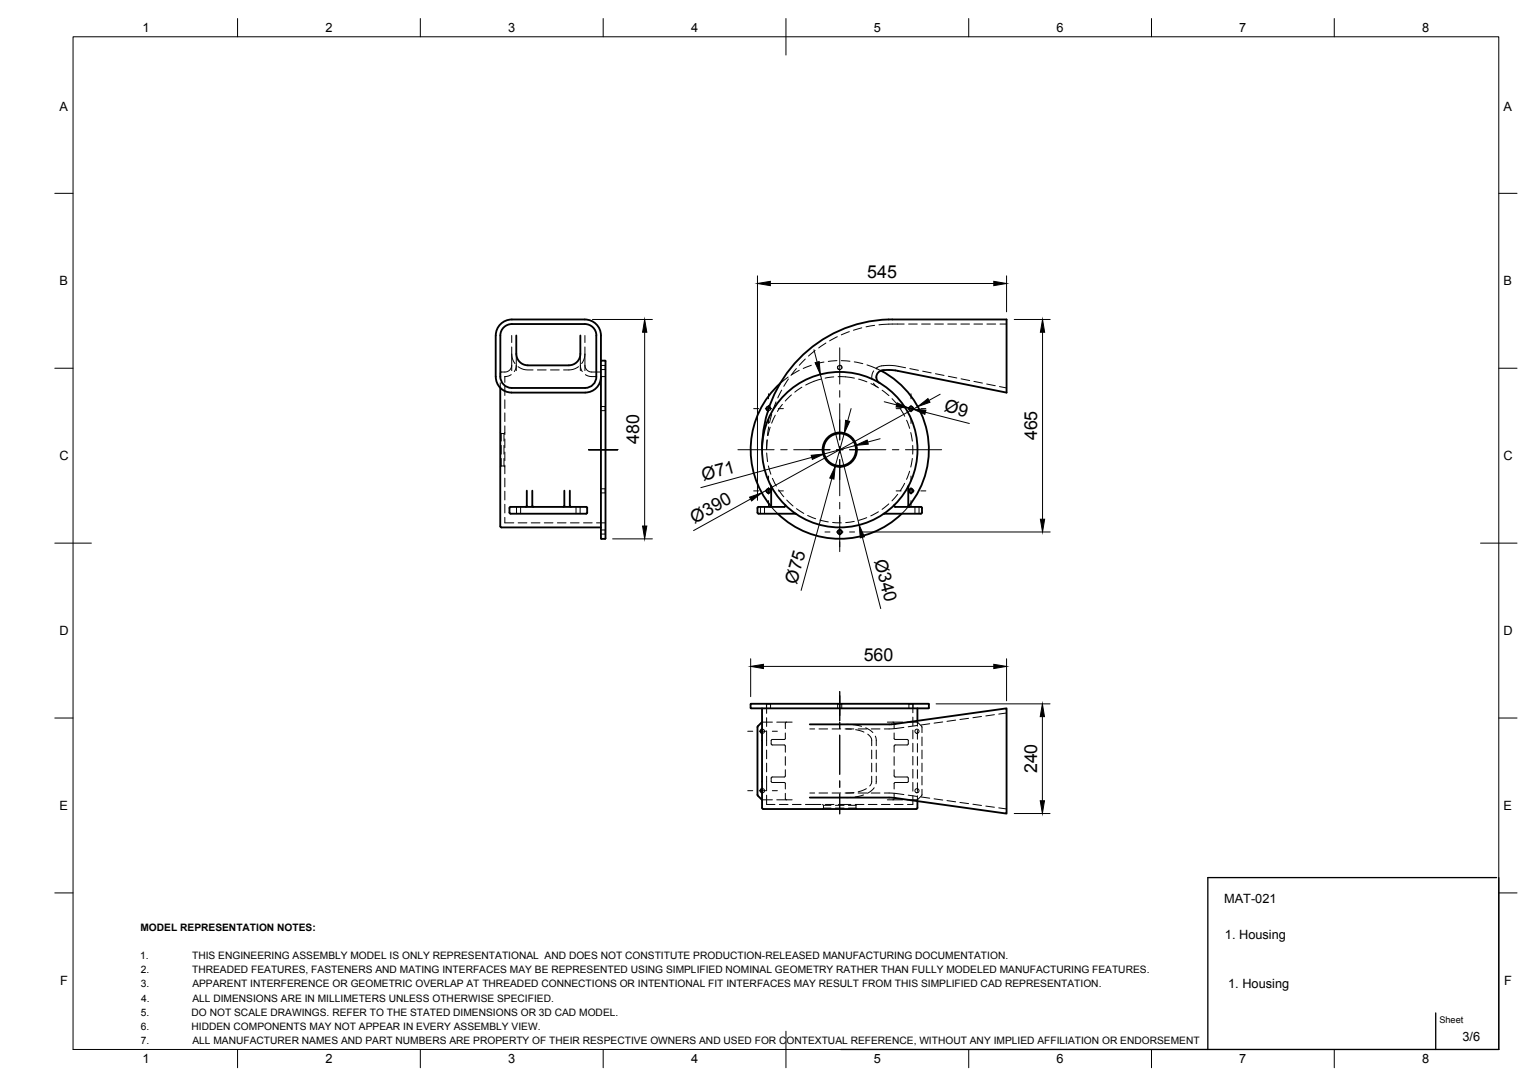
ISO-10303-21;
HEADER;
/* Generated by software containing ST-Developer
 * from STEP Tools, Inc. (www.steptools.com) 
 */

FILE_DESCRIPTION(
/* description */ ('STEP AP214'),
/* implementation_level */ '2;1');

FILE_NAME(
/* name */ '1. Housing.step',
/* time_stamp */ '2026-11-14T06:27:21-08:00',
/* author */ (''),
/* organization */ (''),
/* preprocessor_version */ 'ST-DEVELOPER v20.2',
/* originating_system */ 'Autodesk Translation Framework v15.17.0.0',
/* authorisation */ '');

FILE_SCHEMA (('AUTOMOTIVE_DESIGN { 1 0 10303 214 3 1 1 }'));
ENDSEC;

DATA;
#10=MECHANICAL_DESIGN_GEOMETRIC_PRESENTATION_REPRESENTATION('',(#35),#27541);
#27=SHAPE_REPRESENTATION_RELATIONSHIP('SRR','None',#27561,#31);
#31=ADVANCED_BREP_SHAPE_REPRESENTATION('',(#62),#27537);
#35=STYLED_ITEM('',(#27590),#62);
#62=MANIFOLD_SOLID_BREP('Body1',#11823);
#89=(
BOUNDED_SURFACE()
B_SPLINE_SURFACE(3,2,((#19385,#19386,#19387),(#19388,#19389,#19390),(#19391,
#19392,#19393),(#19394,#19395,#19396)),.UNSPECIFIED.,.F.,.F.,.F.)
B_SPLINE_SURFACE_WITH_KNOTS((4,4),(3,3),(4.8580615908835,4.90978454023457),
(0.,1.),.UNSPECIFIED.)
GEOMETRIC_REPRESENTATION_ITEM()
RATIONAL_B_SPLINE_SURFACE(((1.,0.714186893169771,1.),(1.,0.715014795561183,
1.),(1.,0.715838114785164,1.),(1.,0.716655802814478,1.)))
REPRESENTATION_ITEM('')
SURFACE()
);
#90=(
BOUNDED_SURFACE()
B_SPLINE_SURFACE(3,2,((#19398,#19399,#19400),(#19401,#19402,#19403),(#19404,
#19405,#19406),(#19407,#19408,#19409),(#19410,#19411,#19412),(#19413,#19414,
#19415)),.UNSPECIFIED.,.F.,.F.,.F.)
B_SPLINE_SURFACE_WITH_KNOTS((4,2,4),(3,3),(0.,0.00940850202008467,0.0188170040401693),
(0.,1.),.UNSPECIFIED.)
GEOMETRIC_REPRESENTATION_ITEM()
RATIONAL_B_SPLINE_SURFACE(((1.,0.707106781186548,1.),(1.,0.707160279657923,
1.),(1.,0.707792511111606,1.),(1.,0.710169444241066,1.),(1.,0.711914113489046,
1.),(1.,0.71418689316977,1.)))
REPRESENTATION_ITEM('')
SURFACE()
);
#91=(
BOUNDED_SURFACE()
B_SPLINE_SURFACE(3,2,((#19609,#19610,#19611),(#19612,#19613,#19614),(#19615,
#19616,#19617),(#19618,#19619,#19620)),.UNSPECIFIED.,.F.,.F.,.F.)
B_SPLINE_SURFACE_WITH_KNOTS((4,4),(3,3),(4.51499342053481,4.56671636988588),
(0.,1.),.UNSPECIFIED.)
GEOMETRIC_REPRESENTATION_ITEM()
RATIONAL_B_SPLINE_SURFACE(((1.,0.716655802814478,1.),(1.,0.715838114785163,
1.),(1.,0.715014795561185,1.),(1.,0.71418689316977,1.)))
REPRESENTATION_ITEM('')
SURFACE()
);
#92=(
BOUNDED_SURFACE()
B_SPLINE_SURFACE(3,2,((#19622,#19623,#19624),(#19625,#19626,#19627),(#19628,
#19629,#19630),(#19631,#19632,#19633),(#19634,#19635,#19636),(#19637,#19638,
#19639)),.UNSPECIFIED.,.F.,.F.,.F.)
B_SPLINE_SURFACE_WITH_KNOTS((4,2,4),(3,3),(0.,0.00940850202008465,0.0188170040401693),
(0.,1.),.UNSPECIFIED.)
GEOMETRIC_REPRESENTATION_ITEM()
RATIONAL_B_SPLINE_SURFACE(((1.,0.707106781186548,1.),(1.,0.707160279657923,
1.),(1.,0.707792511111607,1.),(1.,0.710169444241066,1.),(1.,0.711914113489046,
1.),(1.,0.714186893169771,1.)))
REPRESENTATION_ITEM('')
SURFACE()
);
#93=(
BOUNDED_SURFACE()
B_SPLINE_SURFACE(3,2,((#19835,#19836,#19837),(#19838,#19839,#19840),(#19841,
#19842,#19843),(#19844,#19845,#19846)),.UNSPECIFIED.,.F.,.F.,.F.)
B_SPLINE_SURFACE_WITH_KNOTS((4,4),(3,3),(0.,0.00696902930539232),(0.,1.),
 .UNSPECIFIED.)
GEOMETRIC_REPRESENTATION_ITEM()
RATIONAL_B_SPLINE_SURFACE(((1.,0.707106781186548,1.),(1.,0.707276293971192,
1.),(1.,0.707276133936197,1.),(1.,0.707106781186548,1.)))
REPRESENTATION_ITEM('')
SURFACE()
);
#94=(
BOUNDED_SURFACE()
B_SPLINE_SURFACE(3,2,((#20013,#20014,#20015),(#20016,#20017,#20018),(#20019,
#20020,#20021),(#20022,#20023,#20024)),.UNSPECIFIED.,.F.,.F.,.F.)
B_SPLINE_SURFACE_WITH_KNOTS((4,4),(3,3),(-3.46944695195361E-18,0.0069690293053924),
(0.,1.),.UNSPECIFIED.)
GEOMETRIC_REPRESENTATION_ITEM()
RATIONAL_B_SPLINE_SURFACE(((1.,0.707106781186547,1.),(1.,0.707276133936197,
1.),(1.,0.707276293971194,1.),(1.,0.707106781186547,1.)))
REPRESENTATION_ITEM('')
SURFACE()
);
#95=(
BOUNDED_SURFACE()
B_SPLINE_SURFACE(3,2,((#20196,#20197,#20198),(#20199,#20200,#20201),(#20202,
#20203,#20204),(#20205,#20206,#20207),(#20208,#20209,#20210),(#20211,#20212,
#20213),(#20214,#20215,#20216),(#20217,#20218,#20219),(#20220,#20221,#20222),
(#20223,#20224,#20225),(#20226,#20227,#20228),(#20229,#20230,#20231),(#20232,
#20233,#20234),(#20235,#20236,#20237),(#20238,#20239,#20240),(#20241,#20242,
#20243),(#20244,#20245,#20246),(#20247,#20248,#20249),(#20250,#20251,#20252),
(#20253,#20254,#20255),(#20256,#20257,#20258),(#20259,#20260,#20261),(#20262,
#20263,#20264),(#20265,#20266,#20267),(#20268,#20269,#20270),(#20271,#20272,
#20273),(#20274,#20275,#20276),(#20277,#20278,#20279),(#20280,#20281,#20282),
(#20283,#20284,#20285),(#20286,#20287,#20288),(#20289,#20290,#20291),(#20292,
#20293,#20294),(#20295,#20296,#20297),(#20298,#20299,#20300),(#20301,#20302,
#20303),(#20304,#20305,#20306),(#20307,#20308,#20309),(#20310,#20311,#20312),
(#20313,#20314,#20315),(#20316,#20317,#20318),(#20319,#20320,#20321)),
 .UNSPECIFIED.,.F.,.F.,.F.)
B_SPLINE_SURFACE_WITH_KNOTS((4,2,2,2,2,2,2,2,2,2,2,2,2,2,2,2,2,2,2,2,4),
(3,3),(-2.08303249130885E-5,0.0143336398395062,0.0286672796790123,0.0430009195185185,
0.0501677394382716,0.0573345593580246,0.0716681991975308,0.086001839037037,
0.100335478876543,0.10391888883642,0.107502298796296,0.114669118716049,
0.143336398395062,0.157670038234568,0.164836858154321,0.168420268114197,
0.172003678074074,0.200670957753086,0.215004597592592,0.222171417512345,
0.229338237432099),(-2.08303249131434E-5,1.),.UNSPECIFIED.)
GEOMETRIC_REPRESENTATION_ITEM()
RATIONAL_B_SPLINE_SURFACE(((1.0000122047894,0.707042750109083,1.),(1.00001165037919,
0.720350516962147,1.),(1.00001112382429,0.732989659531489,1.),(1.00001011791998,
0.757134849634084,1.),(1.00000963848844,0.768642868569314,1.),(1.00000871933328,
0.790705778250952,1.),(1.00000827963345,0.801260098384088,1.),(1.00000764642268,
0.816459351757556,1.),(1.00000743975533,0.821420084465031,1.),(1.00000703478498,
0.83114077643061,1.),(1.00000683745965,0.835877268408073,1.),(1.00000626125477,
0.849708182685712,1.),(1.00000589749541,0.858439668308409,1.),(1.00000520616899,
0.875033898554219,1.),(1.00000487861603,0.882896305052256,1.),(1.00000425655478,
0.897827931239669,1.),(1.00000396205458,0.904896956720407,1.),(1.00000361326943,
0.913269009275214,1.),(1.00000354448169,0.914920153464801,1.),(1.00000340882056,
0.918176490920243,1.),(1.00000334190225,0.919782762301647,1.),(1.00000314471007,
0.924516058194436,1.),(1.00000301778241,0.927562762018953,1.),(1.00000240476706,
0.942277255118144,1.),(1.00000198296934,0.952401862584738,1.),(1.0000014408388,
0.965414874578938,1.),(1.00000127533739,0.969387482068598,1.),(1.00000104925894,
0.974814148585356,1.),(1.00000097760072,0.976534194128842,1.),(1.0000008756353,
0.978981717570214,1.),(1.00000084253972,0.979776126225882,1.),(1.00000077837346,
0.981316338884772,1.),(1.00000074729348,0.982062366173435,1.),(1.00000047647086,
0.988563047871222,1.),(1.0000002985221,0.992834434768701,1.),(1.00000011982054,
0.997123891622385,1.),(1.00000007504731,0.998198604512223,1.),(1.00000003010649,
0.999277339877407,1.),(1.00000001883456,0.999547905223287,1.),(1.00000000377558,
0.999909373055038,1.),(0.999999999994412,1.00000013413799,1.),(1.,1.,1.)))
REPRESENTATION_ITEM('')
SURFACE()
);
#96=(
BOUNDED_SURFACE()
B_SPLINE_SURFACE(3,2,((#20325,#20326,#20327),(#20328,#20329,#20330),(#20331,
#20332,#20333),(#20334,#20335,#20336),(#20337,#20338,#20339),(#20340,#20341,
#20342),(#20343,#20344,#20345),(#20346,#20347,#20348),(#20349,#20350,#20351),
(#20352,#20353,#20354),(#20355,#20356,#20357),(#20358,#20359,#20360),(#20361,
#20362,#20363),(#20364,#20365,#20366),(#20367,#20368,#20369),(#20370,#20371,
#20372),(#20373,#20374,#20375),(#20376,#20377,#20378),(#20379,#20380,#20381),
(#20382,#20383,#20384),(#20385,#20386,#20387),(#20388,#20389,#20390),(#20391,
#20392,#20393),(#20394,#20395,#20396),(#20397,#20398,#20399),(#20400,#20401,
#20402),(#20403,#20404,#20405),(#20406,#20407,#20408),(#20409,#20410,#20411),
(#20412,#20413,#20414),(#20415,#20416,#20417),(#20418,#20419,#20420),(#20421,
#20422,#20423),(#20424,#20425,#20426),(#20427,#20428,#20429),(#20430,#20431,
#20432),(#20433,#20434,#20435),(#20436,#20437,#20438),(#20439,#20440,#20441),
(#20442,#20443,#20444),(#20445,#20446,#20447),(#20448,#20449,#20450),(#20451,
#20452,#20453),(#20454,#20455,#20456)),.UNSPECIFIED.,.F.,.F.,.F.)
B_SPLINE_SURFACE_WITH_KNOTS((4,2,2,2,2,2,2,2,2,2,2,2,2,2,2,2,2,2,2,2,2,
4),(3,3),(0.,0.0134129175527026,0.0268258351054052,0.0335322938817565,0.0368855232699322,
0.0402387526581078,0.0469452114344592,0.0536516702108105,0.0603581289871618,
0.0637113583753374,0.0670645877635131,0.0737710465398644,0.0804775053162157,
0.0838307347043914,0.087183964092567,0.0905371934807427,0.0938904228689183,
0.0955670375630061,0.097243652257094,0.10059688164527,0.103950111033445,
0.107303340421621),(0.,1.),.UNSPECIFIED.)
GEOMETRIC_REPRESENTATION_ITEM()
RATIONAL_B_SPLINE_SURFACE(((1.,0.707106781186548,1.),(1.,0.692435075400818,
1.),(1.,0.677415299381314,1.),(1.,0.646471084851157,1.),(1.,0.63054857897306,
1.),(1.,0.605783714123967,1.),(1.,0.597381263170599,1.),(1.,0.584523409966303,
1.),(1.,0.580195037882829,1.),(1.,0.571447189603745,1.),(1.,0.56702021135895,
1.),(1.,0.553648440044157,1.),(1.,0.544640272160397,1.),(1.,0.526415110072128,
1.),(1.,0.51719794329847,1.),(1.,0.498539063660432,1.),(1.,0.489096977102246,
1.),(1.,0.474763871347392,1.),(1.,0.469957977677047,1.),(1.,0.460292200732756,
1.),(1.,0.455439380592845,1.),(1.,0.440953583986291,1.),(1.,0.431346601606819,
1.),(1.,0.412377017907544,1.),(1.,0.403011528923584,1.),(1.,0.389351796591827,
1.),(1.,0.384854537462147,1.),(1.,0.376177060931741,1.),(1.,0.371982004193461,
1.),(1.,0.363944301803223,1.),(1.,0.360101535707161,1.),(1.,0.352850425245751,
1.),(1.,0.349441929276512,1.),(1.,0.344732409186674,1.),(1.,0.343226443951063,
1.),(1.,0.340393341785211,1.),(1.,0.339063346120003,1.),(1.,0.335345379291585,
1.),(1.,0.333229400572389,1.),(1.,0.329790328424277,1.),(1.,0.328467328740303,
1.),(1.,0.326681697649074,1.),(1.,0.326219073225421,1.),(1.,0.326219127150631,
1.)))
REPRESENTATION_ITEM('')
SURFACE()
);
#97=(
BOUNDED_SURFACE()
B_SPLINE_SURFACE(3,2,((#20457,#20458,#20459),(#20460,#20461,#20462),(#20463,
#20464,#20465),(#20466,#20467,#20468),(#20469,#20470,#20471),(#20472,#20473,
#20474),(#20475,#20476,#20477),(#20478,#20479,#20480),(#20481,#20482,#20483),
(#20484,#20485,#20486),(#20487,#20488,#20489),(#20490,#20491,#20492),(#20493,
#20494,#20495),(#20496,#20497,#20498),(#20499,#20500,#20501),(#20502,#20503,
#20504),(#20505,#20506,#20507),(#20508,#20509,#20510),(#20511,#20512,#20513),
(#20514,#20515,#20516),(#20517,#20518,#20519),(#20520,#20521,#20522),(#20523,
#20524,#20525),(#20526,#20527,#20528),(#20529,#20530,#20531),(#20532,#20533,
#20534),(#20535,#20536,#20537),(#20538,#20539,#20540),(#20541,#20542,#20543),
(#20544,#20545,#20546),(#20547,#20548,#20549),(#20550,#20551,#20552),(#20553,
#20554,#20555),(#20556,#20557,#20558),(#20559,#20560,#20561),(#20562,#20563,
#20564),(#20565,#20566,#20567),(#20568,#20569,#20570),(#20571,#20572,#20573),
(#20574,#20575,#20576),(#20577,#20578,#20579),(#20580,#20581,#20582),(#20583,
#20584,#20585),(#20586,#20587,#20588),(#20589,#20590,#20591),(#20592,#20593,
#20594)),.UNSPECIFIED.,.F.,.F.,.F.)
B_SPLINE_SURFACE_WITH_KNOTS((4,2,2,2,2,2,2,2,2,2,2,2,2,2,2,2,2,2,2,2,2,
2,4),(3,3),(0.,0.00337857504716453,0.00675715009432906,0.0101357251414936,
0.0118250126650759,0.0135143001886581,0.0168928752358226,0.0202714502829872,
0.0236500253301517,0.025339312853734,0.0270286003773162,0.0337857504716453,
0.0405429005659744,0.0439214756131389,0.0473000506603034,0.0540572007546325,
0.0608143508489615,0.0675715009432906,0.0709500759904551,0.0743286510376197,
0.0810858011319487,0.0946001013206068,0.108114401509265),(0.,1.),
 .UNSPECIFIED.)
GEOMETRIC_REPRESENTATION_ITEM()
RATIONAL_B_SPLINE_SURFACE(((1.,0.32621912715063,1.),(1.,0.326219068852315,
1.),(1.,0.326681715050001,1.),(1.,0.328468620211654,1.),(1.,0.32979287514018,
1.),(1.,0.333236641150815,1.),(1.,0.33535605687756,1.),(1.,0.339081365168914,
1.),(1.,0.340414170801098,1.),(1.,0.34325369454111,1.),(1.,0.344759275422739,
1.),(1.,0.349467998468122,1.),(1.,0.352877852486234,1.),(1.,0.360137129421262,
1.),(1.,0.363986689978637,1.),(1.,0.372044278816161,1.),(1.,0.37625241873187,
1.),(1.,0.382785172371532,1.),(1.,0.385002445825604,1.),(1.,0.389470383554178,
1.),(1.,0.391724641087319,1.),(1.,0.403081163733532,1.),(1.,0.412431784451128,
1.),(1.,0.431385484934698,1.),(1.,0.440991365631289,1.),(1.,0.455485214499389,
1.),(1.,0.460343755015816,1.),(1.,0.469998884973711,1.),(1.,0.474798889815344,
1.),(1.,0.48911283545623,1.),(1.,0.498540168051125,1.),(1.,0.517166334136202,
1.),(1.,0.526365537230034,1.),(1.,0.544552008443698,1.),(1.,0.553539446694172,
1.),(1.,0.566878228388953,1.),(1.,0.571308885947455,1.),(1.,0.580076325189919,
1.),(1.,0.584413767367782,1.),(1.,0.597296867359364,1.),(1.,0.605713540127583,
1.),(1.,0.630514573129104,1.),(1.,0.646452607022068,1.),(1.,0.677415122211174,
1.),(1.,0.692437606205447,1.),(1.,0.707106781186548,1.)))
REPRESENTATION_ITEM('')
SURFACE()
);
#98=(
BOUNDED_SURFACE()
B_SPLINE_SURFACE(3,2,((#20598,#20599,#20600),(#20601,#20602,#20603),(#20604,
#20605,#20606),(#20607,#20608,#20609),(#20610,#20611,#20612),(#20613,#20614,
#20615),(#20616,#20617,#20618),(#20619,#20620,#20621),(#20622,#20623,#20624),
(#20625,#20626,#20627),(#20628,#20629,#20630),(#20631,#20632,#20633),(#20634,
#20635,#20636),(#20637,#20638,#20639),(#20640,#20641,#20642),(#20643,#20644,
#20645),(#20646,#20647,#20648),(#20649,#20650,#20651),(#20652,#20653,#20654),
(#20655,#20656,#20657),(#20658,#20659,#20660),(#20661,#20662,#20663),(#20664,
#20665,#20666),(#20667,#20668,#20669),(#20670,#20671,#20672),(#20673,#20674,
#20675),(#20676,#20677,#20678),(#20679,#20680,#20681),(#20682,#20683,#20684),
(#20685,#20686,#20687),(#20688,#20689,#20690),(#20691,#20692,#20693),(#20694,
#20695,#20696),(#20697,#20698,#20699),(#20700,#20701,#20702),(#20703,#20704,
#20705),(#20706,#20707,#20708),(#20709,#20710,#20711),(#20712,#20713,#20714),
(#20715,#20716,#20717),(#20718,#20719,#20720),(#20721,#20722,#20723)),
 .UNSPECIFIED.,.F.,.F.,.F.)
B_SPLINE_SURFACE_WITH_KNOTS((4,2,2,2,2,2,2,2,2,2,2,2,2,2,2,2,2,2,2,2,4),
(3,3),(-2.08246099844738E-5,0.0143336398395062,0.0286672796790123,0.0430009195185185,
0.0501677394382716,0.0573345593580247,0.0716681991975308,0.086001839037037,
0.100335478876543,0.10391888883642,0.107502298796296,0.114669118716049,
0.143336398395062,0.157670038234568,0.164836858154321,0.168420268114197,
0.172003678074074,0.200670957753086,0.215004597592593,0.222171417512346,
0.229338237432099),(0.,1.00002082460998),.UNSPECIFIED.)
GEOMETRIC_REPRESENTATION_ITEM()
RATIONAL_B_SPLINE_SURFACE(((1.,0.707042767677887,1.00001220144021),(1.,
0.720350528626315,1.00001164718235),(1.,0.732989665864678,1.00001112077214),
(1.,0.757134851024669,1.00001011514401),(1.,0.768642869892271,1.000009635844),
(1.,0.790705779446232,1.00000871694103),(1.,0.801260099519581,1.00000827736183),
(1.,0.816459352806589,1.00000764432479),(1.,0.821420085485447,1.00000743771414),
(1.,0.831140777395743,1.00000703285491),(1.,0.835877269346536,1.00000683558371),
(1.,0.849708183543533,1.00000625953692),(1.,0.85843966911793,1.00000589587736),
(1.,0.875033899267846,1.00000520474062),(1.,0.882896305722012,1.00000487727752),
(1.,0.897827931823032,1.00000425538694),(1.,0.904896957262567,1.00000396096755),
(1.,0.913269009771199,1.00000361227809),(1.,0.914920153950816,1.00000354350922),
(1.,0.918176491388049,1.00000340788531),(1.,0.919782762760141,1.00000334098536),
(1.,0.924516058625678,1.00000314384728),(1.,0.927562762433317,1.00000301695444),
(1.,0.94227725544642,1.00000240410729),(1.,0.952401862855693,1.00000198242528),
(1.,0.965414874777115,1.00000144044349),(1.,0.969387482243809,1.00000127498749),
(1.,0.974814148729155,1.00000104897106),(1.,0.976534194262543,1.0000009773325),
(1.,0.97898171769053,1.00000087539506),(1.,0.979776126341324,1.00000084230856),
(1.,0.981316338991679,1.00000077815991),(1.,0.982062366275678,1.00000074708845),
(1.,0.988563047938719,1.00000047634013),(1.,0.992834434811244,1.0000002984402),
(1.,0.997123891638026,1.00000011978767),(1.,0.998198604522518,1.00000007502672),
(1.,0.999277339881537,1.00000003009823),(1.,0.999547905226004,1.00000001882939),
(1.,0.999909373055422,1.00000000377454),(1.,1.00000013413809,0.999999999994413),
(1.,1.,1.)))
REPRESENTATION_ITEM('')
SURFACE()
);
#99=(
BOUNDED_SURFACE()
B_SPLINE_SURFACE(3,2,((#20852,#20853,#20854),(#20855,#20856,#20857),(#20858,
#20859,#20860),(#20861,#20862,#20863)),.UNSPECIFIED.,.F.,.F.,.F.)
B_SPLINE_SURFACE_WITH_KNOTS((4,4),(3,3),(4.8580615908835,4.90978454023457),
(0.,1.),.UNSPECIFIED.)
GEOMETRIC_REPRESENTATION_ITEM()
RATIONAL_B_SPLINE_SURFACE(((1.,0.714186893169771,1.),(1.,0.715014795561184,
1.),(1.,0.715838114785164,1.),(1.,0.716655802814478,1.)))
REPRESENTATION_ITEM('')
SURFACE()
);
#100=(
BOUNDED_SURFACE()
B_SPLINE_SURFACE(3,2,((#20865,#20866,#20867),(#20868,#20869,#20870),(#20871,
#20872,#20873),(#20874,#20875,#20876),(#20877,#20878,#20879),(#20880,#20881,
#20882)),.UNSPECIFIED.,.F.,.F.,.F.)
B_SPLINE_SURFACE_WITH_KNOTS((4,2,4),(3,3),(0.,0.00940850202008467,0.0188170040401693),
(0.,1.),.UNSPECIFIED.)
GEOMETRIC_REPRESENTATION_ITEM()
RATIONAL_B_SPLINE_SURFACE(((1.,0.707106781186548,1.),(1.,0.707160279657923,
1.),(1.,0.707792511111606,1.),(1.,0.710169444241066,1.),(1.,0.711914113489048,
1.),(1.,0.714186893169771,1.)))
REPRESENTATION_ITEM('')
SURFACE()
);
#101=(
BOUNDED_SURFACE()
B_SPLINE_SURFACE(3,2,((#21103,#21104,#21105),(#21106,#21107,#21108),(#21109,
#21110,#21111),(#21112,#21113,#21114)),.UNSPECIFIED.,.F.,.F.,.F.)
B_SPLINE_SURFACE_WITH_KNOTS((4,4),(3,3),(4.51499342053481,4.56671636988588),
(0.,1.),.UNSPECIFIED.)
GEOMETRIC_REPRESENTATION_ITEM()
RATIONAL_B_SPLINE_SURFACE(((1.,0.716655802814478,1.),(1.,0.715838114785163,
1.),(1.,0.715014795561185,1.),(1.,0.71418689316977,1.)))
REPRESENTATION_ITEM('')
SURFACE()
);
#102=(
BOUNDED_SURFACE()
B_SPLINE_SURFACE(3,2,((#21116,#21117,#21118),(#21119,#21120,#21121),(#21122,
#21123,#21124),(#21125,#21126,#21127),(#21128,#21129,#21130),(#21131,#21132,
#21133)),.UNSPECIFIED.,.F.,.F.,.F.)
B_SPLINE_SURFACE_WITH_KNOTS((4,2,4),(3,3),(-1.38777878078145E-17,0.00940850202008464,
0.0188170040401693),(0.,1.),.UNSPECIFIED.)
GEOMETRIC_REPRESENTATION_ITEM()
RATIONAL_B_SPLINE_SURFACE(((1.,0.707106781186548,1.),(1.,0.707160279657923,
1.),(1.,0.707792511111607,1.),(1.,0.710169444241066,1.),(1.,0.711914113489046,
1.),(1.,0.714186893169771,1.)))
REPRESENTATION_ITEM('')
SURFACE()
);
#103=(
BOUNDED_SURFACE()
B_SPLINE_SURFACE(3,2,((#21362,#21363,#21364),(#21365,#21366,#21367),(#21368,
#21369,#21370),(#21371,#21372,#21373)),.UNSPECIFIED.,.F.,.F.,.F.)
B_SPLINE_SURFACE_WITH_KNOTS((4,4),(3,3),(0.,0.00696902930539231),(0.,1.),
 .UNSPECIFIED.)
GEOMETRIC_REPRESENTATION_ITEM()
RATIONAL_B_SPLINE_SURFACE(((1.,0.707106781186548,1.),(1.,0.707276293971192,
1.),(1.,0.707276133936197,1.),(1.,0.707106781186548,1.)))
REPRESENTATION_ITEM('')
SURFACE()
);
#104=(
BOUNDED_SURFACE()
B_SPLINE_SURFACE(3,2,((#21540,#21541,#21542),(#21543,#21544,#21545),(#21546,
#21547,#21548),(#21549,#21550,#21551)),.UNSPECIFIED.,.F.,.F.,.F.)
B_SPLINE_SURFACE_WITH_KNOTS((4,4),(3,3),(-3.46944695195361E-18,0.0069690293053924),
(0.,1.),.UNSPECIFIED.)
GEOMETRIC_REPRESENTATION_ITEM()
RATIONAL_B_SPLINE_SURFACE(((1.,0.707106781186547,1.),(1.,0.707276133936196,
1.),(1.,0.707276293971194,1.),(1.,0.707106781186547,1.)))
REPRESENTATION_ITEM('')
SURFACE()
);
#105=(
BOUNDED_SURFACE()
B_SPLINE_SURFACE(3,2,((#21711,#21712,#21713),(#21714,#21715,#21716),(#21717,
#21718,#21719),(#21720,#21721,#21722),(#21723,#21724,#21725),(#21726,#21727,
#21728),(#21729,#21730,#21731),(#21732,#21733,#21734),(#21735,#21736,#21737),
(#21738,#21739,#21740),(#21741,#21742,#21743),(#21744,#21745,#21746),(#21747,
#21748,#21749),(#21750,#21751,#21752),(#21753,#21754,#21755),(#21756,#21757,
#21758),(#21759,#21760,#21761),(#21762,#21763,#21764),(#21765,#21766,#21767),
(#21768,#21769,#21770),(#21771,#21772,#21773),(#21774,#21775,#21776),(#21777,
#21778,#21779),(#21780,#21781,#21782),(#21783,#21784,#21785),(#21786,#21787,
#21788),(#21789,#21790,#21791),(#21792,#21793,#21794),(#21795,#21796,#21797),
(#21798,#21799,#21800),(#21801,#21802,#21803),(#21804,#21805,#21806),(#21807,
#21808,#21809),(#21810,#21811,#21812),(#21813,#21814,#21815),(#21816,#21817,
#21818),(#21819,#21820,#21821),(#21822,#21823,#21824),(#21825,#21826,#21827),
(#21828,#21829,#21830),(#21831,#21832,#21833),(#21834,#21835,#21836)),
 .UNSPECIFIED.,.F.,.F.,.F.)
B_SPLINE_SURFACE_WITH_KNOTS((4,2,2,2,2,2,2,2,2,2,2,2,2,2,2,2,2,2,2,2,4),
(3,3),(-1.33632684703268E-5,0.0143336398395061,0.0286672796790123,0.0430009195185185,
0.0501677394382715,0.0573345593580246,0.0716681991975308,0.086001839037037,
0.100335478876543,0.10391888883642,0.107502298796296,0.114669118716049,
0.143336398395062,0.157670038234568,0.164836858154321,0.168420268114197,
0.172003678074074,0.200670957753086,0.215004597592592,0.222171417512345,
0.229338237432099),(-1.33632684703573E-5,1.),.UNSPECIFIED.)
GEOMETRIC_REPRESENTATION_ITEM()
RATIONAL_B_SPLINE_SURFACE(((1.00000782911927,0.707065704608532,1.),(1.000007473655,
0.72036575434847,1.),(1.00000713604048,0.732997937829732,1.),(1.00000649089595,
0.757136663085689,1.),(1.00000618332875,0.768644596089292,1.),(1.00000559366798,
0.790707341030961,1.),(1.00000531158966,0.801261582354705,1.),(1.00000490536929,
0.816460722237655,1.),(1.00000477278707,0.821421417903966,1.),(1.00000451298858,
0.831142037285297,1.),(1.0000043863995,0.835878493896513,1.),(1.00000401674981,
0.849709304899285,1.),(1.00000378338918,0.858440725325112,1.),(1.00000333988619,
0.875034831663981,1.),(1.00000312975286,0.882897179455003,1.),(1.00000273068518,
0.89782869414732,1.),(1.00000254175602,0.904897666844873,1.),(1.00000231800172,
0.913269656887061,1.),(1.00000227387268,0.914920788747183,1.),(1.00000218684271,
0.918177101888678,1.),(1.00000214391296,0.919783361275745,1.),(1.0000020174093,
0.924516621825683,1.),(1.00000193598206,0.92756330290103,1.),(1.00000154271755,
0.942277686126561,1.),(1.00000127212388,0.952402217994254,1.),(1.00000092433373,
0.965415132823172,1.),(1.00000081816048,0.969387710649768,1.),(1.00000067312556,
0.974814336645346,1.),(1.00000062715504,0.976534369345689,1.),(1.00000056174171,
0.978981874511646,1.),(1.00000054051007,0.979776277235544,1.),(1.00000049934583,
0.981316478393818,1.),(1.00000047940725,0.982062500111768,1.),(1.00000030566784,
0.988563133271413,1.),(1.00000019150931,0.992834488272736,1.),(1.00000007686784,
0.997123913098267,1.),(1.0000000481447,0.998198617963065,1.),(1.00000001931406,
0.999277345273439,1.),(1.00000001208284,0.999547908599034,1.),(1.00000000242213,
0.99990937373174,1.),(0.999999999996415,1.00000013413699,1.),(1.,1.,1.)))
REPRESENTATION_ITEM('')
SURFACE()
);
#106=(
BOUNDED_SURFACE()
B_SPLINE_SURFACE(3,2,((#21840,#21841,#21842),(#21843,#21844,#21845),(#21846,
#21847,#21848),(#21849,#21850,#21851),(#21852,#21853,#21854),(#21855,#21856,
#21857),(#21858,#21859,#21860),(#21861,#21862,#21863),(#21864,#21865,#21866),
(#21867,#21868,#21869),(#21870,#21871,#21872),(#21873,#21874,#21875),(#21876,
#21877,#21878),(#21879,#21880,#21881),(#21882,#21883,#21884),(#21885,#21886,
#21887),(#21888,#21889,#21890),(#21891,#21892,#21893),(#21894,#21895,#21896),
(#21897,#21898,#21899),(#21900,#21901,#21902),(#21903,#21904,#21905),(#21906,
#21907,#21908),(#21909,#21910,#21911),(#21912,#21913,#21914),(#21915,#21916,
#21917),(#21918,#21919,#21920),(#21921,#21922,#21923),(#21924,#21925,#21926),
(#21927,#21928,#21929),(#21930,#21931,#21932),(#21933,#21934,#21935),(#21936,
#21937,#21938),(#21939,#21940,#21941),(#21942,#21943,#21944),(#21945,#21946,
#21947),(#21948,#21949,#21950),(#21951,#21952,#21953),(#21954,#21955,#21956),
(#21957,#21958,#21959),(#21960,#21961,#21962),(#21963,#21964,#21965),(#21966,
#21967,#21968),(#21969,#21970,#21971),(#21972,#21973,#21974),(#21975,#21976,
#21977)),.UNSPECIFIED.,.F.,.F.,.F.)
B_SPLINE_SURFACE_WITH_KNOTS((4,2,2,2,2,2,2,2,2,2,2,2,2,2,2,2,2,2,2,2,2,
2,4),(3,3),(0.,0.0134129175527026,0.0268258351054052,0.0335322938817565,
0.0368855232699322,0.0402387526581078,0.0469452114344592,0.0536516702108105,
0.0603581289871618,0.0637113583753374,0.0670645877635131,0.0737710465398644,
0.07712427592804,0.0804775053162157,0.0838307347043914,0.087183964092567,
0.0905371934807427,0.0938904228689183,0.0955670375630061,0.097243652257094,
0.10059688164527,0.103950111033445,0.107303340421621),(0.,1.),
 .UNSPECIFIED.)
GEOMETRIC_REPRESENTATION_ITEM()
RATIONAL_B_SPLINE_SURFACE(((1.,0.707106781186548,1.),(1.,0.692435075401192,
1.),(1.,0.677415299380816,1.),(1.,0.646471084851654,1.),(1.,0.630548578972812,
1.),(1.,0.605783714124091,1.),(1.,0.597381263170474,1.),(1.,0.584523409966366,
1.),(1.,0.580195037882892,1.),(1.,0.571447189603682,1.),(1.,0.56702021135914,
1.),(1.,0.553648440043779,1.),(1.,0.544640272160396,1.),(1.,0.526415110072127,
1.),(1.,0.517197943298344,1.),(1.,0.498539063660557,1.),(1.,0.489096977102497,
1.),(1.,0.474763871347267,1.),(1.,0.469957977677141,1.),(1.,0.460292200732662,
1.),(1.,0.455439380593066,1.),(1.,0.440953583985851,1.),(1.,0.431346601607069,
1.),(1.,0.417119413832237,1.),(1.,0.412408247679678,1.),(1.,0.403077747649425,
1.),(1.,0.398458284812998,1.),(1.,0.389351796591827,1.),(1.,0.384854537462053,
1.),(1.,0.376177060931835,1.),(1.,0.371982004193336,1.),(1.,0.363944301803349,
1.),(1.,0.360101535706815,1.),(1.,0.352850425246096,1.),(1.,0.349441929276512,
1.),(1.,0.344732409186674,1.),(1.,0.343226443951127,1.),(1.,0.340393341785148,
1.),(1.,0.339063346120349,1.),(1.,0.335345379290893,1.),(1.,0.333229400572264,
1.),(1.,0.329790328424402,1.),(1.,0.328467328740178,1.),(1.,0.326681697649199,
1.),(1.,0.326219073225326,1.),(1.,0.326219127150631,1.)))
REPRESENTATION_ITEM('')
SURFACE()
);
#107=(
BOUNDED_SURFACE()
B_SPLINE_SURFACE(3,2,((#21978,#21979,#21980),(#21981,#21982,#21983),(#21984,
#21985,#21986),(#21987,#21988,#21989),(#21990,#21991,#21992),(#21993,#21994,
#21995),(#21996,#21997,#21998),(#21999,#22000,#22001),(#22002,#22003,#22004),
(#22005,#22006,#22007),(#22008,#22009,#22010),(#22011,#22012,#22013),(#22014,
#22015,#22016),(#22017,#22018,#22019),(#22020,#22021,#22022),(#22023,#22024,
#22025),(#22026,#22027,#22028),(#22029,#22030,#22031),(#22032,#22033,#22034),
(#22035,#22036,#22037),(#22038,#22039,#22040),(#22041,#22042,#22043),(#22044,
#22045,#22046),(#22047,#22048,#22049),(#22050,#22051,#22052),(#22053,#22054,
#22055),(#22056,#22057,#22058),(#22059,#22060,#22061),(#22062,#22063,#22064),
(#22065,#22066,#22067),(#22068,#22069,#22070),(#22071,#22072,#22073),(#22074,
#22075,#22076),(#22077,#22078,#22079),(#22080,#22081,#22082),(#22083,#22084,
#22085),(#22086,#22087,#22088),(#22089,#22090,#22091),(#22092,#22093,#22094),
(#22095,#22096,#22097),(#22098,#22099,#22100),(#22101,#22102,#22103),(#22104,
#22105,#22106),(#22107,#22108,#22109),(#22110,#22111,#22112),(#22113,#22114,
#22115),(#22116,#22117,#22118),(#22119,#22120,#22121)),.UNSPECIFIED.,.F.,
 .F.,.F.)
B_SPLINE_SURFACE_WITH_KNOTS((4,2,2,2,2,2,2,2,2,2,2,2,2,2,2,2,2,2,2,2,2,
2,2,4),(3,3),(0.,0.00337857504716453,0.00675715009432906,0.0101357251414936,
0.0118250126650759,0.0135143001886581,0.0168928752358226,0.0202714502829872,
0.0236500253301517,0.025339312853734,0.0270286003773162,0.0304071754244808,
0.0337857504716453,0.0405429005659744,0.0439214756131389,0.0473000506603034,
0.0540572007546325,0.0608143508489615,0.0675715009432906,0.0709500759904551,
0.0743286510376197,0.0810858011319487,0.0946001013206068,0.108114401509265),
(0.,1.),.UNSPECIFIED.)
GEOMETRIC_REPRESENTATION_ITEM()
RATIONAL_B_SPLINE_SURFACE(((1.,0.32621912715063,1.),(1.,0.326219068852551,
1.),(1.,0.326681715049687,1.),(1.,0.328468620211968,1.),(1.,0.329792875139961,
1.),(1.,0.333236641151033,1.),(1.,0.33535605687756,1.),(1.,0.339081365168914,
1.),(1.,0.340414170800971,1.),(1.,0.343253694541237,1.),(1.,0.344759275422691,
1.),(1.,0.349467998468217,1.),(1.,0.352877852486455,1.),(1.,0.360137129421043,
1.),(1.,0.363986689978511,1.),(1.,0.372044278816287,1.),(1.,0.37625241873225,
1.),(1.,0.382785172371342,1.),(1.,0.385002445825604,1.),(1.,0.389470383554178,
1.),(1.,0.391724641087209,1.),(1.,0.398538554675267,1.),(1.,0.403148955697984,
1.),(1.,0.412464720989499,1.),(1.,0.417170209572146,1.),(1.,0.431385484934447,
1.),(1.,0.44099136563173,1.),(1.,0.455485214499169,1.),(1.,0.460343755015469,
1.),(1.,0.469998884974058,1.),(1.,0.474798889815438,1.),(1.,0.489112835456042,
1.),(1.,0.498540168051997,1.),(1.,0.517166334135328,1.),(1.,0.526365537230033,
1.),(1.,0.544552008443698,1.),(1.,0.553539446694675,1.),(1.,0.566878228388702,
1.),(1.,0.571308885947581,1.),(1.,0.580076325189793,1.),(1.,0.584413767367218,
1.),(1.,0.597296867360491,1.),(1.,0.605713540127086,1.),(1.,0.630514573130101,
1.),(1.,0.646452607020576,1.),(1.,0.677415122212667,1.),(1.,0.692437606204326,
1.),(1.,0.707106781186548,1.)))
REPRESENTATION_ITEM('')
SURFACE()
);
#108=(
BOUNDED_SURFACE()
B_SPLINE_SURFACE(3,2,((#22125,#22126,#22127),(#22128,#22129,#22130),(#22131,
#22132,#22133),(#22134,#22135,#22136),(#22137,#22138,#22139),(#22140,#22141,
#22142),(#22143,#22144,#22145),(#22146,#22147,#22148),(#22149,#22150,#22151),
(#22152,#22153,#22154),(#22155,#22156,#22157),(#22158,#22159,#22160),(#22161,
#22162,#22163),(#22164,#22165,#22166),(#22167,#22168,#22169),(#22170,#22171,
#22172),(#22173,#22174,#22175),(#22176,#22177,#22178),(#22179,#22180,#22181),
(#22182,#22183,#22184),(#22185,#22186,#22187),(#22188,#22189,#22190),(#22191,
#22192,#22193),(#22194,#22195,#22196),(#22197,#22198,#22199),(#22200,#22201,
#22202),(#22203,#22204,#22205),(#22206,#22207,#22208),(#22209,#22210,#22211),
(#22212,#22213,#22214),(#22215,#22216,#22217),(#22218,#22219,#22220),(#22221,
#22222,#22223),(#22224,#22225,#22226),(#22227,#22228,#22229),(#22230,#22231,
#22232),(#22233,#22234,#22235),(#22236,#22237,#22238),(#22239,#22240,#22241),
(#22242,#22243,#22244),(#22245,#22246,#22247),(#22248,#22249,#22250)),
 .UNSPECIFIED.,.F.,.F.,.F.)
B_SPLINE_SURFACE_WITH_KNOTS((4,2,2,2,2,2,2,2,2,2,2,2,2,2,2,2,2,2,2,2,4),
(3,3),(-1.33640092427433E-5,0.0143336398395062,0.0286672796790123,0.0430009195185185,
0.0501677394382716,0.0573345593580247,0.0716681991975309,0.086001839037037,
0.100335478876543,0.10391888883642,0.107502298796296,0.114669118716049,
0.143336398395062,0.157670038234568,0.164836858154321,0.168420268114198,
0.172003678074074,0.200670957753086,0.215004597592593,0.222171417512346,
0.229338237432099),(0.,1.00001336400924),.UNSPECIFIED.)
GEOMETRIC_REPRESENTATION_ITEM()
RATIONAL_B_SPLINE_SURFACE(((1.,0.707065702331389,1.00000782955332),(1.,
0.720365752837665,1.00000747406933),(1.,0.732997937007419,1.00000713643607),
(1.,0.757136662906848,1.00000649125576),(1.,0.768644595917913,1.00000618367152),
(1.,0.790707340875925,1.00000559397806),(1.,0.801261582208021,1.0000053118841),
(1.,0.81646072210143,1.00000490564121),(1.,0.821421417771145,1.00000477305165),
(1.,0.83114203716075,1.00000451323875),(1.,0.835878493775337,1.00000438664265),
(1.,0.849709304787154,1.00000401697248),(1.,0.858440725220516,1.00000378359891),
(1.,0.875034831571146,1.00000334007133),(1.,0.882897179367727,1.00000312992635),
(1.,0.897828694072166,1.00000273083655),(1.,0.904897666774157,1.00000254189692),
(1.,0.913269656822881,1.00000231813022),(1.,0.914920788684494,1.00000227399873),
(1.,0.918177101827732,1.00000218696394),(1.,0.919783361216391,1.0000021440318),
(1.,0.924516621769634,1.00000201752113),(1.,0.927563302847372,1.00000193608938),
(1.,0.942277686083803,1.00000154280307),(1.,0.952402217960055,1.0000012721944),
(1.,0.965415132797023,1.00000092438497),(1.,0.969387710627092,1.00000081820584),
(1.,0.97481433662669,1.00000067316288),(1.,0.976534369328306,1.00000062718981),
(1.,0.978981874496077,1.00000056177285),(1.,0.979776277220496,1.00000054054004),
(1.,0.981316478380045,1.00000049937351),(1.,0.982062500098414,1.00000047943383),
(1.,0.988563133263475,1.00000030568479),(1.,0.99283448826902,1.00000019151993),
(1.,0.99712391309534,1.0000000768721),(1.,0.998198617961198,1.00000004814737),
(1.,0.99927734527317,1.00000001931513),(1.,0.999547908598833,1.00000001208351),
(1.,0.999909373731539,1.00000000242226),(1.,1.00000013413709,0.999999999996415),
(1.,1.,1.)))
REPRESENTATION_ITEM('')
SURFACE()
);
#109=(
BOUNDED_SURFACE()
B_SPLINE_SURFACE(3,2,((#22566,#22567,#22568),(#22569,#22570,#22571),(#22572,
#22573,#22574),(#22575,#22576,#22577),(#22578,#22579,#22580),(#22581,#22582,
#22583),(#22584,#22585,#22586),(#22587,#22588,#22589),(#22590,#22591,#22592),
(#22593,#22594,#22595),(#22596,#22597,#22598),(#22599,#22600,#22601),(#22602,
#22603,#22604),(#22605,#22606,#22607),(#22608,#22609,#22610),(#22611,#22612,
#22613),(#22614,#22615,#22616),(#22617,#22618,#22619),(#22620,#22621,#22622),
(#22623,#22624,#22625)),.UNSPECIFIED.,.F.,.F.,.F.)
B_SPLINE_SURFACE_WITH_KNOTS((4,2,2,2,2,2,2,2,2,4),(3,3),(0.00505837679447142,
0.00808192097035447,0.00959369305829599,0.0111054651462375,0.012617237234179,
0.0141290093221206,0.0148848953660913,0.0156407814100621,0.0163966674540328,
0.0171525534980036),(0.,1.),.UNSPECIFIED.)
GEOMETRIC_REPRESENTATION_ITEM()
RATIONAL_B_SPLINE_SURFACE(((1.,0.707106781186547,1.),(1.,0.739053872509116,
1.),(1.,0.768433399252105,1.),(1.,0.809724042302045,1.),(1.,0.823019853650823,
1.),(1.,0.848781685567262,1.),(1.,0.861247499610797,1.),(1.,0.885026508477437,
1.),(1.,0.896438871456505,1.),(1.,0.917922922305835,1.),(1.,0.927944217122039,
1.),(1.,0.94161381312465,1.),(1.,0.945967473187117,1.),(1.,0.953895740028491,
1.),(1.,0.957485583333028,1.),(1.,0.963663001673968,1.),(1.,0.966147540420567,
1.),(1.,0.969624030438212,1.),(1.,0.970601281761249,1.),(1.,0.970581776826274,
1.)))
REPRESENTATION_ITEM('')
SURFACE()
);
#110=(
BOUNDED_SURFACE()
B_SPLINE_SURFACE(3,2,((#22864,#22865,#22866),(#22867,#22868,#22869),(#22870,
#22871,#22872),(#22873,#22874,#22875),(#22876,#22877,#22878),(#22879,#22880,
#22881),(#22882,#22883,#22884),(#22885,#22886,#22887),(#22888,#22889,#22890),
(#22891,#22892,#22893),(#22894,#22895,#22896),(#22897,#22898,#22899),(#22900,
#22901,#22902),(#22903,#22904,#22905),(#22906,#22907,#22908),(#22909,#22910,
#22911),(#22912,#22913,#22914),(#22915,#22916,#22917),(#22918,#22919,#22920),
(#22921,#22922,#22923),(#22924,#22925,#22926),(#22927,#22928,#22929)),
 .UNSPECIFIED.,.F.,.F.,.F.)
B_SPLINE_SURFACE_WITH_KNOTS((4,2,2,2,2,2,2,2,2,2,4),(3,3),(0.00605768062302923,
0.00847740131122415,0.00968726165532161,0.0108971219994191,0.0115020521714678,
0.0121069823435165,0.013316842687614,0.0139217728596627,0.0145267030317114,
0.0151316332037602,0.0157365633758089),(0.,1.),.UNSPECIFIED.)
GEOMETRIC_REPRESENTATION_ITEM()
RATIONAL_B_SPLINE_SURFACE(((1.,0.707106781186548,1.),(1.,0.678435467809058,
1.),(1.,0.648724429803459,1.),(1.,0.601883782649935,1.),(1.,0.58582572598482,
1.),(1.,0.553093074718013,1.),(1.,0.5366611790602,1.),(1.,0.512036824267513,
1.),(1.,0.503834051867292,1.),(1.,0.487490014313552,1.),(1.,0.479322252109144,
1.),(1.,0.455536119849462,1.),(1.,0.440447953764078,1.),(1.,0.420111511643565,
1.),(1.,0.413771933679107,1.),(1.,0.402532175621877,1.),(1.,0.39758573118173,
1.),(1.,0.38936895214063,1.),(1.,0.386109902300535,1.),(1.,0.381795928046837,
1.),(1.,0.380693466310634,1.),(1.,0.380693493813436,1.)))
REPRESENTATION_ITEM('')
SURFACE()
);
#111=(
BOUNDED_SURFACE()
B_SPLINE_SURFACE(3,2,((#22940,#22941,#22942),(#22943,#22944,#22945),(#22946,
#22947,#22948),(#22949,#22950,#22951),(#22952,#22953,#22954),(#22955,#22956,
#22957),(#22958,#22959,#22960),(#22961,#22962,#22963),(#22964,#22965,#22966),
(#22967,#22968,#22969),(#22970,#22971,#22972),(#22973,#22974,#22975),(#22976,
#22977,#22978),(#22979,#22980,#22981),(#22982,#22983,#22984),(#22985,#22986,
#22987),(#22988,#22989,#22990),(#22991,#22992,#22993),(#22994,#22995,#22996),
(#22997,#22998,#22999),(#23000,#23001,#23002),(#23003,#23004,#23005)),
 .UNSPECIFIED.,.F.,.F.,.F.)
B_SPLINE_SURFACE_WITH_KNOTS((4,2,2,2,2,2,2,2,2,2,4),(3,3),(0.00359639911601392,
0.00436249387044424,0.00512858862487456,0.00589468337930487,0.00666077813373519,
0.00742687288816551,0.00819296764259583,0.00972515715145646,0.0112573466603171,
0.0127895361691777,0.015853915186899),(0.,1.),.UNSPECIFIED.)
GEOMETRIC_REPRESENTATION_ITEM()
RATIONAL_B_SPLINE_SURFACE(((1.,0.970581776826274,1.),(1.,0.970578649532394,
1.),(1.,0.96964070956466,1.),(1.,0.966106916844896,1.),(1.,0.963560009136893,
1.),(1.,0.95740233193304,1.),(1.,0.953739105221087,1.),(1.,0.945797353495694,
1.),(1.,0.94149269169882,1.),(1.,0.932342624911764,1.),(1.,0.927470686999509,
1.),(1.,0.917384026303788,1.),(1.,0.912174865626315,1.),(1.,0.896095641265424,
1.),(1.,0.884778088998196,1.),(1.,0.86100319646455,1.),(1.,0.848496565440572,
1.),(1.,0.822764671287953,1.),(1.,0.809488242768719,1.),(1.,0.768270175598826,
1.),(1.,0.738957849522124,1.),(1.,0.707106781186541,1.)))
REPRESENTATION_ITEM('')
SURFACE()
);
#112=(
BOUNDED_SURFACE()
B_SPLINE_SURFACE(3,2,((#23036,#23037,#23038),(#23039,#23040,#23041),(#23042,
#23043,#23044),(#23045,#23046,#23047),(#23048,#23049,#23050),(#23051,#23052,
#23053),(#23054,#23055,#23056),(#23057,#23058,#23059),(#23060,#23061,#23062),
(#23063,#23064,#23065),(#23066,#23067,#23068),(#23069,#23070,#23071),(#23072,
#23073,#23074),(#23075,#23076,#23077),(#23078,#23079,#23080),(#23081,#23082,
#23083),(#23084,#23085,#23086),(#23087,#23088,#23089),(#23090,#23091,#23092),
(#23093,#23094,#23095)),.UNSPECIFIED.,.F.,.F.,.F.)
B_SPLINE_SURFACE_WITH_KNOTS((4,2,2,2,2,2,2,2,2,4),(3,3),(0.00387143063410007,
0.00471388371892886,0.00539035064546607,0.00606681757200329,0.0067432844985405,
0.00809621835161492,0.00944915220468934,0.0108020860577638,0.0121550199108382,
0.0150268737752786),(0.,1.00016598615829),.UNSPECIFIED.)
GEOMETRIC_REPRESENTATION_ITEM()
RATIONAL_B_SPLINE_SURFACE(((1.,0.955399887158975,1.00001480600278),(1.,
0.955829132859094,1.00001466350509),(1.,0.955152845891184,1.00001488801364),
(1.,0.952140174640701,1.0000158881371),(1.,0.95012712734567,1.00001655641307),
(1.,0.945126911092976,1.00001821634644),(1.,0.942132982861274,1.00001921024773),
(1.,0.935297780612531,1.00002147934566),(1.,0.931461499156383,1.0000227528849),
(1.,0.919200779571961,1.00002682310438),(1.,0.909918466100668,1.00002990457549),
(1.,0.889588132182854,1.00003665368354),(1.,0.878801976969414,1.00004023438847),
(1.,0.856103617498776,1.00004776961545),(1.,0.844188170450328,1.00005172521401),
(1.,0.819187865450958,1.00006002462317),(1.,0.806145836648029,1.00006435421569),
(1.,0.764361494284231,1.00007822546062),(1.,0.734139217941498,1.00008825841971),
(0.999999999999999,0.701407786598383,1.0000991243488)))
REPRESENTATION_ITEM('')
SURFACE()
);
#113=(
BOUNDED_SURFACE()
B_SPLINE_SURFACE(3,2,((#23218,#23219,#23220),(#23221,#23222,#23223),(#23224,
#23225,#23226),(#23227,#23228,#23229),(#23230,#23231,#23232),(#23233,#23234,
#23235),(#23236,#23237,#23238),(#23239,#23240,#23241),(#23242,#23243,#23244),
(#23245,#23246,#23247),(#23248,#23249,#23250),(#23251,#23252,#23253),(#23254,
#23255,#23256),(#23257,#23258,#23259),(#23260,#23261,#23262),(#23263,#23264,
#23265),(#23266,#23267,#23268),(#23269,#23270,#23271),(#23272,#23273,#23274),
(#23275,#23276,#23277)),.UNSPECIFIED.,.F.,.F.,.F.)
B_SPLINE_SURFACE_WITH_KNOTS((4,2,2,2,2,2,2,2,2,4),(3,3),(0.00433666893074964,
0.00702103924194056,0.00836322439753602,0.00970540955313147,0.0110475947087269,
0.0123897798643224,0.0130608724421201,0.0137319650199178,0.0144030575977156,
0.0150741501755133),(0.,1.),.UNSPECIFIED.)
GEOMETRIC_REPRESENTATION_ITEM()
RATIONAL_B_SPLINE_SURFACE(((1.,0.707106781186548,1.),(1.,0.737894213217654,
1.),(1.,0.766274690665779,1.),(1.,0.80619741544873,1.),(1.,0.81905917672634,
1.),(1.,0.843975019036595,1.),(1.,0.856066072681341,1.),(1.,0.878882708476932,
1.),(1.,0.889682618268665,1.),(1.,0.909952939738908,1.),(1.,0.91926443717337,
1.),(1.,0.931500456841751,1.),(1.,0.935322128839039,1.),(1.,0.942157243325948,
1.),(1.,0.945149563733463,1.),(1.,0.950144827786557,1.),(1.,0.952152129590434,
1.),(1.,0.954830461683239,1.),(1.,0.955531530247581,1.),(1.,0.95553308590591,
1.)))
REPRESENTATION_ITEM('')
SURFACE()
);
#114=(
BOUNDED_SURFACE()
B_SPLINE_SURFACE(3,2,((#23495,#23496,#23497),(#23498,#23499,#23500),(#23501,
#23502,#23503),(#23504,#23505,#23506),(#23507,#23508,#23509),(#23510,#23511,
#23512),(#23513,#23514,#23515),(#23516,#23517,#23518),(#23519,#23520,#23521),
(#23522,#23523,#23524),(#23525,#23526,#23527),(#23528,#23529,#23530),(#23531,
#23532,#23533),(#23534,#23535,#23536),(#23537,#23538,#23539),(#23540,#23541,
#23542),(#23543,#23544,#23545),(#23546,#23547,#23548),(#23549,#23550,#23551),
(#23552,#23553,#23554),(#23555,#23556,#23557),(#23558,#23559,#23560),(#23561,
#23562,#23563),(#23564,#23565,#23566)),.UNSPECIFIED.,.F.,.F.,.F.)
B_SPLINE_SURFACE_WITH_KNOTS((4,2,2,2,2,2,2,2,2,2,2,4),(3,3),(0.00449003234654763,
0.00509682357326747,0.00570361479998732,0.00631040602670716,0.00691719725342701,
0.00752398848014685,0.00813077970686669,0.00873757093358654,0.00934436216030638,
0.0105579446137461,0.0117715270671858,0.0141986919740651),(0.,1.),
 .UNSPECIFIED.)
GEOMETRIC_REPRESENTATION_ITEM()
RATIONAL_B_SPLINE_SURFACE(((1.,0.38069349381344,1.),(1.,0.380693826435357,
1.),(1.,0.381828035551871,1.),(1.,0.386153151069475,1.),(1.,0.389343566002074,
1.),(1.,0.397589118267461,1.),(1.,0.402611271260585,1.),(1.,0.413872221609166,
1.),(1.,0.420140875257451,1.),(1.,0.43367980618183,1.),(1.,0.440958379002546,
1.),(1.,0.455908840578608,1.),(1.,0.463628155372052,1.),(1.,0.479401310239419,
1.),(1.,0.487456032708626,1.),(1.,0.503805154106481,1.),(1.,0.51211354879696,
1.),(1.,0.53683753947851,1.),(1.,0.553207213585367,1.),(1.,0.585605914285066,
1.),(1.,0.601711645280215,1.),(1.,0.649056040268748,1.),(1.,0.678719733465159,
1.),(1.,0.707106781186549,1.)))
REPRESENTATION_ITEM('')
SURFACE()
);
#115=(
BOUNDED_SURFACE()
B_SPLINE_SURFACE(3,2,((#23571,#23572,#23573),(#23574,#23575,#23576),(#23577,
#23578,#23579),(#23580,#23581,#23582),(#23583,#23584,#23585),(#23586,#23587,
#23588),(#23589,#23590,#23591),(#23592,#23593,#23594),(#23595,#23596,#23597),
(#23598,#23599,#23600),(#23601,#23602,#23603),(#23604,#23605,#23606),(#23607,
#23608,#23609),(#23610,#23611,#23612),(#23613,#23614,#23615),(#23616,#23617,
#23618),(#23619,#23620,#23621),(#23622,#23623,#23624),(#23625,#23626,#23627),
(#23628,#23629,#23630)),.UNSPECIFIED.,.F.,.F.,.F.)
B_SPLINE_SURFACE_WITH_KNOTS((4,2,2,2,2,2,2,2,2,4),(3,3),(0.00505837679447142,
0.00808192097035447,0.00959369305829599,0.0111054651462375,0.012617237234179,
0.0141290093221206,0.0148848953660913,0.0156407814100621,0.0163966674540328,
0.0171525534980036),(0.,1.),.UNSPECIFIED.)
GEOMETRIC_REPRESENTATION_ITEM()
RATIONAL_B_SPLINE_SURFACE(((1.,0.707106781186547,1.),(1.,0.739053872509117,
1.),(1.,0.768433399252105,1.),(1.,0.809724042302045,1.),(1.,0.823019853650822,
1.),(1.,0.848781685567261,1.),(1.,0.861247499610797,1.),(1.,0.885026508477437,
1.),(1.,0.896438871456477,1.),(1.,0.917922922305863,1.),(1.,0.927944217122039,
1.),(1.,0.94161381312465,1.),(1.,0.945967473187117,1.),(1.,0.953895740028491,
1.),(1.,0.957485583333028,1.),(1.,0.963663001673968,1.),(1.,0.966147540420553,
1.),(1.,0.969624030438226,1.),(1.,0.970601281761238,1.),(1.,0.970581776826274,
1.)))
REPRESENTATION_ITEM('')
SURFACE()
);
#116=(
BOUNDED_SURFACE()
B_SPLINE_SURFACE(3,2,((#23752,#23753,#23754),(#23755,#23756,#23757),(#23758,
#23759,#23760),(#23761,#23762,#23763),(#23764,#23765,#23766),(#23767,#23768,
#23769),(#23770,#23771,#23772),(#23773,#23774,#23775),(#23776,#23777,#23778),
(#23779,#23780,#23781),(#23782,#23783,#23784),(#23785,#23786,#23787),(#23788,
#23789,#23790),(#23791,#23792,#23793),(#23794,#23795,#23796),(#23797,#23798,
#23799),(#23800,#23801,#23802),(#23803,#23804,#23805),(#23806,#23807,#23808),
(#23809,#23810,#23811),(#23812,#23813,#23814),(#23815,#23816,#23817)),
 .UNSPECIFIED.,.F.,.F.,.F.)
B_SPLINE_SURFACE_WITH_KNOTS((4,2,2,2,2,2,2,2,2,2,4),(3,3),(0.00359639911601392,
0.00436249387044424,0.00512858862487455,0.00589468337930487,0.00666077813373519,
0.00742687288816551,0.00819296764259582,0.00972515715145646,0.0112573466603171,
0.0127895361691777,0.015853915186899),(0.,1.),.UNSPECIFIED.)
GEOMETRIC_REPRESENTATION_ITEM()
RATIONAL_B_SPLINE_SURFACE(((1.,0.970581776826274,1.),(1.,0.970578649532459,
1.),(1.,0.969640709564574,1.),(1.,0.966106916844982,1.),(1.,0.963560009136894,
1.),(1.,0.95740233193304,1.),(1.,0.953739105221087,1.),(1.,0.945797353495694,
1.),(1.,0.94149269169882,1.),(1.,0.932342624911764,1.),(1.,0.927470686999452,
1.),(1.,0.917384026303845,1.),(1.,0.912174865626315,1.),(1.,0.896095641265424,
1.),(1.,0.884778088998393,1.),(1.,0.861003196464352,1.),(1.,0.848496565440543,
1.),(1.,0.822764671287981,1.),(1.,0.809488242768579,1.),(1.,0.768270175599105,
1.),(1.,0.738957849521914,1.),(1.,0.70710678118654,1.)))
REPRESENTATION_ITEM('')
SURFACE()
);
#117=(
BOUNDED_SURFACE()
B_SPLINE_SURFACE(3,2,((#24059,#24060,#24061),(#24062,#24063,#24064),(#24065,
#24066,#24067),(#24068,#24069,#24070),(#24071,#24072,#24073),(#24074,#24075,
#24076),(#24077,#24078,#24079),(#24080,#24081,#24082),(#24083,#24084,#24085),
(#24086,#24087,#24088),(#24089,#24090,#24091),(#24092,#24093,#24094),(#24095,
#24096,#24097),(#24098,#24099,#24100),(#24101,#24102,#24103),(#24104,#24105,
#24106),(#24107,#24108,#24109),(#24110,#24111,#24112),(#24113,#24114,#24115),
(#24116,#24117,#24118),(#24119,#24120,#24121),(#24122,#24123,#24124),(#24125,
#24126,#24127),(#24128,#24129,#24130)),.UNSPECIFIED.,.F.,.F.,.F.)
B_SPLINE_SURFACE_WITH_KNOTS((4,2,2,2,2,2,2,2,2,2,2,4),(3,3),(0.00449003234654763,
0.00509682357326747,0.00570361479998732,0.00631040602670716,0.00691719725342701,
0.00752398848014685,0.00813077970686669,0.00873757093358654,0.00934436216030638,
0.0105579446137461,0.0117715270671858,0.0141986919740651),(0.,1.),
 .UNSPECIFIED.)
GEOMETRIC_REPRESENTATION_ITEM()
RATIONAL_B_SPLINE_SURFACE(((1.,0.38069349381344,1.),(1.,0.380693826435357,
1.),(1.,0.381828035551871,1.),(1.,0.386153151069475,1.),(1.,0.389343566002074,
1.),(1.,0.397589118267461,1.),(1.,0.402611271260585,1.),(1.,0.413872221609166,
1.),(1.,0.420140875257451,1.),(1.,0.43367980618183,1.),(1.,0.440958379002546,
1.),(1.,0.455908840578608,1.),(1.,0.463628155372052,1.),(1.,0.479401310239419,
1.),(1.,0.487456032708626,1.),(1.,0.503805154106481,1.),(1.,0.51211354879696,
1.),(1.,0.53683753947851,1.),(1.,0.553207213585367,1.),(1.,0.585605914285066,
1.),(1.,0.601711645280215,1.),(1.,0.649056040268748,1.),(1.,0.678719733465158,
1.),(1.,0.707106781186549,1.)))
REPRESENTATION_ITEM('')
SURFACE()
);
#118=(
BOUNDED_SURFACE()
B_SPLINE_SURFACE(3,2,((#24136,#24137,#24138),(#24139,#24140,#24141),(#24142,
#24143,#24144),(#24145,#24146,#24147),(#24148,#24149,#24150),(#24151,#24152,
#24153),(#24154,#24155,#24156),(#24157,#24158,#24159),(#24160,#24161,#24162),
(#24163,#24164,#24165),(#24166,#24167,#24168),(#24169,#24170,#24171),(#24172,
#24173,#24174),(#24175,#24176,#24177),(#24178,#24179,#24180),(#24181,#24182,
#24183),(#24184,#24185,#24186),(#24187,#24188,#24189),(#24190,#24191,#24192),
(#24193,#24194,#24195)),.UNSPECIFIED.,.F.,.F.,.F.)
B_SPLINE_SURFACE_WITH_KNOTS((4,2,2,2,2,2,2,2,2,4),(3,3),(0.00433666893074964,
0.00702103924194056,0.00836322439753602,0.00970540955313147,0.0110475947087269,
0.0123897798643224,0.0130608724421201,0.0137319650199178,0.0144030575977156,
0.0150741501755133),(0.,1.),.UNSPECIFIED.)
GEOMETRIC_REPRESENTATION_ITEM()
RATIONAL_B_SPLINE_SURFACE(((1.,0.707106781186548,1.),(1.,0.737894213217654,
1.),(1.,0.766274690665779,1.),(1.,0.80619741544873,1.),(1.,0.81905917672634,
1.),(1.,0.843975019036595,1.),(1.,0.856066072681341,1.),(1.,0.878882708476932,
1.),(1.,0.889682618268665,1.),(1.,0.909952939738908,1.),(1.,0.91926443717337,
1.),(1.,0.931500456841751,1.),(1.,0.935322128839039,1.),(1.,0.942157243325948,
1.),(1.,0.945149563733463,1.),(1.,0.950144827786557,1.),(1.,0.952152129590434,
1.),(1.,0.954830461683239,1.),(1.,0.955531530247581,1.),(1.,0.95553308590591,
1.)))
REPRESENTATION_ITEM('')
SURFACE()
);
#119=(
BOUNDED_SURFACE()
B_SPLINE_SURFACE(3,2,((#24227,#24228,#24229),(#24230,#24231,#24232),(#24233,
#24234,#24235),(#24236,#24237,#24238),(#24239,#24240,#24241),(#24242,#24243,
#24244),(#24245,#24246,#24247),(#24248,#24249,#24250),(#24251,#24252,#24253),
(#24254,#24255,#24256),(#24257,#24258,#24259),(#24260,#24261,#24262),(#24263,
#24264,#24265),(#24266,#24267,#24268),(#24269,#24270,#24271),(#24272,#24273,
#24274),(#24275,#24276,#24277),(#24278,#24279,#24280),(#24281,#24282,#24283),
(#24284,#24285,#24286)),.UNSPECIFIED.,.F.,.F.,.F.)
B_SPLINE_SURFACE_WITH_KNOTS((4,2,2,2,2,2,2,2,2,4),(3,3),(0.0038714306340967,
0.00471388371892886,0.00539035064546608,0.00606681757200329,0.0067432844985405,
0.00809621835161492,0.00944915220468935,0.0108020860577638,0.0121550199108382,
0.015026873775282),(0.,1.00016598615829),.UNSPECIFIED.)
GEOMETRIC_REPRESENTATION_ITEM()
RATIONAL_B_SPLINE_SURFACE(((1.,0.95539988715897,1.00001480600278),(1.,0.955829132859099,
1.00001466350509),(1.,0.95515284589119,1.00001488801364),(1.,0.952140174640701,
1.0000158881371),(1.,0.95012712734567,1.00001655641307),(1.,0.945126911092976,
1.00001821634644),(1.,0.942132982861274,1.00001921024773),(1.,0.935297780612531,
1.00002147934566),(1.,0.931461499156483,1.0000227528849),(1.,0.91920077957176,
1.00002682310438),(1.,0.909918466100895,1.00002990457549),(1.,0.889588132182626,
1.00003665368354),(1.,0.878801976969414,1.00004023438847),(1.,0.856103617498775,
1.00004776961545),(1.,0.844188170450328,1.00005172521401),(1.,0.819187865450958,
1.00006002462317),(1.,0.806145836648402,1.00006435421569),(1.,0.764361494283404,
1.00007822546062),(1.,0.734139217942157,1.00008825841971),(1.,0.701407786598142,
1.0000991243488)))
REPRESENTATION_ITEM('')
SURFACE()
);
#120=(
BOUNDED_SURFACE()
B_SPLINE_SURFACE(3,2,((#24515,#24516,#24517),(#24518,#24519,#24520),(#24521,
#24522,#24523),(#24524,#24525,#24526),(#24527,#24528,#24529),(#24530,#24531,
#24532),(#24533,#24534,#24535),(#24536,#24537,#24538),(#24539,#24540,#24541),
(#24542,#24543,#24544),(#24545,#24546,#24547),(#24548,#24549,#24550),(#24551,
#24552,#24553),(#24554,#24555,#24556),(#24557,#24558,#24559),(#24560,#24561,
#24562),(#24563,#24564,#24565),(#24566,#24567,#24568),(#24569,#24570,#24571),
(#24572,#24573,#24574),(#24575,#24576,#24577),(#24578,#24579,#24580)),
 .UNSPECIFIED.,.F.,.F.,.F.)
B_SPLINE_SURFACE_WITH_KNOTS((4,2,2,2,2,2,2,2,2,2,4),(3,3),(0.00359639911601392,
0.00436249387044424,0.00512858862487455,0.00589468337930487,0.00666077813373519,
0.00742687288816551,0.00819296764259582,0.00972515715145646,0.0112573466603171,
0.0127895361691777,0.015853915186899),(0.,1.),.UNSPECIFIED.)
GEOMETRIC_REPRESENTATION_ITEM()
RATIONAL_B_SPLINE_SURFACE(((1.,0.970581776826274,1.),(1.,0.970578649532459,
1.),(1.,0.969640709564574,1.),(1.,0.966106916844982,1.),(1.,0.963560009136894,
1.),(1.,0.95740233193304,1.),(1.,0.953739105221087,1.),(1.,0.945797353495694,
1.),(1.,0.94149269169882,1.),(1.,0.932342624911764,1.),(1.,0.927470686999452,
1.),(1.,0.917384026303845,1.),(1.,0.912174865626315,1.),(1.,0.896095641265424,
1.),(1.,0.884778088998393,1.),(1.,0.861003196464352,1.),(1.,0.848496565440543,
1.),(1.,0.822764671287981,1.),(1.,0.809488242768579,1.),(1.,0.768270175599105,
1.),(1.,0.738957849521914,1.),(1.,0.70710678118654,1.)))
REPRESENTATION_ITEM('')
SURFACE()
);
#121=(
BOUNDED_SURFACE()
B_SPLINE_SURFACE(3,2,((#24584,#24585,#24586),(#24587,#24588,#24589),(#24590,
#24591,#24592),(#24593,#24594,#24595),(#24596,#24597,#24598),(#24599,#24600,
#24601),(#24602,#24603,#24604),(#24605,#24606,#24607),(#24608,#24609,#24610),
(#24611,#24612,#24613),(#24614,#24615,#24616),(#24617,#24618,#24619),(#24620,
#24621,#24622),(#24623,#24624,#24625),(#24626,#24627,#24628),(#24629,#24630,
#24631),(#24632,#24633,#24634),(#24635,#24636,#24637),(#24638,#24639,#24640),
(#24641,#24642,#24643),(#24644,#24645,#24646),(#24647,#24648,#24649)),
 .UNSPECIFIED.,.F.,.F.,.F.)
B_SPLINE_SURFACE_WITH_KNOTS((4,2,2,2,2,2,2,2,2,2,4),(3,3),(0.00605768062302923,
0.00847740131122415,0.00968726165532161,0.0108971219994191,0.0115020521714678,
0.0121069823435165,0.013316842687614,0.0139217728596627,0.0145267030317115,
0.0151316332037602,0.0157365633758089),(0.,1.),.UNSPECIFIED.)
GEOMETRIC_REPRESENTATION_ITEM()
RATIONAL_B_SPLINE_SURFACE(((1.,0.707106781186548,1.),(1.,0.678435467809629,
1.),(1.,0.6487244298027,1.),(1.,0.601883782650315,1.),(1.,0.58582572598378,
1.),(1.,0.553093074719053,1.),(1.,0.536661179059662,1.),(1.,0.512036824267783,
1.),(1.,0.503834051867293,1.),(1.,0.487490014313552,1.),(1.,0.479322252109327,
1.),(1.,0.455536119849103,1.),(1.,0.440447953764904,1.),(1.,0.420111511643149,
1.),(1.,0.413771933679518,1.),(1.,0.402532175621466,1.),(1.,0.397585731180899,
1.),(1.,0.389368952141461,1.),(1.,0.386109902300579,1.),(1.,0.38179592804679,
1.),(1.,0.380693466310667,1.),(1.,0.38069349381344,1.)))
REPRESENTATION_ITEM('')
SURFACE()
);
#122=(
BOUNDED_SURFACE()
B_SPLINE_SURFACE(3,2,((#24765,#24766,#24767),(#24768,#24769,#24770),(#24771,
#24772,#24773),(#24774,#24775,#24776),(#24777,#24778,#24779),(#24780,#24781,
#24782),(#24783,#24784,#24785),(#24786,#24787,#24788),(#24789,#24790,#24791),
(#24792,#24793,#24794),(#24795,#24796,#24797),(#24798,#24799,#24800),(#24801,
#24802,#24803),(#24804,#24805,#24806),(#24807,#24808,#24809),(#24810,#24811,
#24812),(#24813,#24814,#24815),(#24816,#24817,#24818),(#24819,#24820,#24821),
(#24822,#24823,#24824)),.UNSPECIFIED.,.F.,.F.,.F.)
B_SPLINE_SURFACE_WITH_KNOTS((4,2,2,2,2,2,2,2,2,4),(3,3),(0.00505837679447141,
0.00808192097035446,0.00959369305829598,0.0111054651462375,0.012617237234179,
0.0141290093221206,0.0148848953660913,0.0156407814100621,0.0163966674540328,
0.0171525534980036),(0.,1.),.UNSPECIFIED.)
GEOMETRIC_REPRESENTATION_ITEM()
RATIONAL_B_SPLINE_SURFACE(((1.,0.707106781186547,1.),(1.,0.739053872510172,
1.),(1.,0.768433399250703,1.),(1.,0.809724042302746,1.),(1.,0.823019853650823,
1.),(1.,0.848781685567262,1.),(1.,0.861247499610966,1.),(1.,0.885026508477268,
1.),(1.,0.896438871456985,1.),(1.,0.917922922305354,1.),(1.,0.927944217122039,
1.),(1.,0.94161381312465,1.),(1.,0.945967473187047,1.),(1.,0.953895740028562,
1.),(1.,0.957485583333028,1.),(1.,0.963663001673968,1.),(1.,0.966147540420553,
1.),(1.,0.969624030438226,1.),(1.,0.970601281761238,1.),(1.,0.970581776826274,
1.)))
REPRESENTATION_ITEM('')
SURFACE()
);
#123=(
BOUNDED_SURFACE()
B_SPLINE_SURFACE(3,2,((#24952,#24953,#24954),(#24955,#24956,#24957),(#24958,
#24959,#24960),(#24961,#24962,#24963),(#24964,#24965,#24966),(#24967,#24968,
#24969),(#24970,#24971,#24972),(#24973,#24974,#24975),(#24976,#24977,#24978),
(#24979,#24980,#24981),(#24982,#24983,#24984),(#24985,#24986,#24987),(#24988,
#24989,#24990),(#24991,#24992,#24993),(#24994,#24995,#24996),(#24997,#24998,
#24999),(#25000,#25001,#25002),(#25003,#25004,#25005),(#25006,#25007,#25008),
(#25009,#25010,#25011)),.UNSPECIFIED.,.F.,.F.,.F.)
B_SPLINE_SURFACE_WITH_KNOTS((4,2,2,2,2,2,2,2,2,4),(3,3),(0.00505837679447142,
0.00808192097035447,0.00959369305829599,0.0111054651462375,0.012617237234179,
0.0141290093221206,0.0148848953660913,0.0156407814100621,0.0163966674540328,
0.0171525534980036),(0.,1.),.UNSPECIFIED.)
GEOMETRIC_REPRESENTATION_ITEM()
RATIONAL_B_SPLINE_SURFACE(((1.,0.707106781186547,1.),(1.,0.739053872509116,
1.),(1.,0.768433399252105,1.),(1.,0.809724042302045,1.),(1.,0.823019853650823,
1.),(1.,0.848781685567262,1.),(1.,0.861247499610797,1.),(1.,0.885026508477437,
1.),(1.,0.896438871456505,1.),(1.,0.917922922305835,1.),(1.,0.927944217122039,
1.),(1.,0.94161381312465,1.),(1.,0.945967473187117,1.),(1.,0.953895740028491,
1.),(1.,0.957485583333028,1.),(1.,0.963663001673968,1.),(1.,0.966147540420567,
1.),(1.,0.969624030438212,1.),(1.,0.970601281761249,1.),(1.,0.970581776826274,
1.)))
REPRESENTATION_ITEM('')
SURFACE()
);
#124=(
BOUNDED_SURFACE()
B_SPLINE_SURFACE(3,2,((#25135,#25136,#25137),(#25138,#25139,#25140),(#25141,
#25142,#25143),(#25144,#25145,#25146),(#25147,#25148,#25149),(#25150,#25151,
#25152),(#25153,#25154,#25155),(#25156,#25157,#25158),(#25159,#25160,#25161),
(#25162,#25163,#25164),(#25165,#25166,#25167),(#25168,#25169,#25170),(#25171,
#25172,#25173),(#25174,#25175,#25176),(#25177,#25178,#25179),(#25180,#25181,
#25182),(#25183,#25184,#25185),(#25186,#25187,#25188),(#25189,#25190,#25191),
(#25192,#25193,#25194),(#25195,#25196,#25197),(#25198,#25199,#25200)),
 .UNSPECIFIED.,.F.,.F.,.F.)
B_SPLINE_SURFACE_WITH_KNOTS((4,2,2,2,2,2,2,2,2,2,4),(3,3),(0.00359639911601392,
0.00436249387044424,0.00512858862487455,0.00589468337930487,0.00666077813373519,
0.00742687288816551,0.00819296764259582,0.00972515715145646,0.0112573466603171,
0.0127895361691777,0.015853915186899),(0.,1.),.UNSPECIFIED.)
GEOMETRIC_REPRESENTATION_ITEM()
RATIONAL_B_SPLINE_SURFACE(((1.,0.970581776826274,1.),(1.,0.970578649532459,
1.),(1.,0.969640709564574,1.),(1.,0.966106916844982,1.),(1.,0.963560009136894,
1.),(1.,0.95740233193304,1.),(1.,0.953739105221087,1.),(1.,0.945797353495694,
1.),(1.,0.94149269169882,1.),(1.,0.932342624911764,1.),(1.,0.927470686999466,
1.),(1.,0.917384026303831,1.),(1.,0.912174865626315,1.),(1.,0.896095641265424,
1.),(1.,0.884778088998309,1.),(1.,0.861003196464437,1.),(1.,0.848496565440628,
1.),(1.,0.822764671287897,1.),(1.,0.809488242768719,1.),(1.,0.768270175598826,
1.),(1.,0.738957849522124,1.),(1.,0.70710678118654,1.)))
REPRESENTATION_ITEM('')
SURFACE()
);
#125=ELLIPSE('',#12050,36.0279058508802,34.9999999999993);
#126=ELLIPSE('',#12051,36.0279058508828,35.0000000000005);
#127=ELLIPSE('',#12052,35.3413355718209,35.0000000000005);
#128=ELLIPSE('',#12053,35.34133557182,34.9999999999995);
#129=ELLIPSE('',#12054,25.2438111227311,25.0000000000022);
#130=ELLIPSE('',#12055,25.24381112273,25.0000000000009);
#131=ELLIPSE('',#12056,25.7342184649135,24.9999999999991);
#132=ELLIPSE('',#12057,25.7342184649167,25.0000000000005);
#205=PLANE('',#12019);
#206=PLANE('',#12020);
#207=PLANE('',#12025);
#208=PLANE('',#12030);
#209=PLANE('',#12034);
#210=PLANE('',#12044);
#211=PLANE('',#12049);
#212=PLANE('',#12058);
#213=PLANE('',#12061);
#214=PLANE('',#12063);
#215=PLANE('',#12065);
#216=PLANE('',#12109);
#217=PLANE('',#12114);
#218=PLANE('',#12124);
#219=PLANE('',#12129);
#220=PLANE('',#12132);
#221=PLANE('',#12134);
#222=PLANE('',#12136);
#223=PLANE('',#12180);
#224=PLANE('',#12181);
#225=PLANE('',#12182);
#226=PLANE('',#12184);
#227=PLANE('',#12186);
#228=PLANE('',#12187);
#229=PLANE('',#12189);
#230=PLANE('',#12191);
#231=PLANE('',#12192);
#232=PLANE('',#12194);
#233=PLANE('',#12196);
#234=PLANE('',#12197);
#235=PLANE('',#12199);
#236=PLANE('',#12201);
#237=PLANE('',#12202);
#238=PLANE('',#12204);
#239=PLANE('',#12206);
#240=PLANE('',#12207);
#241=PLANE('',#12209);
#242=PLANE('',#12211);
#243=PLANE('',#12212);
#244=PLANE('',#12213);
#245=PLANE('',#12214);
#246=PLANE('',#12215);
#247=PLANE('',#12216);
#542=FACE_BOUND('',#1419,.T.);
#543=FACE_BOUND('',#1420,.T.);
#544=FACE_BOUND('',#1422,.T.);
#545=FACE_BOUND('',#1423,.T.);
#546=FACE_BOUND('',#1425,.T.);
#547=FACE_BOUND('',#1426,.T.);
#548=FACE_BOUND('',#1428,.T.);
#549=FACE_BOUND('',#1429,.T.);
#550=FACE_BOUND('',#1431,.T.);
#551=FACE_BOUND('',#1437,.T.);
#552=FACE_BOUND('',#1470,.T.);
#553=FACE_BOUND('',#1508,.T.);
#554=FACE_BOUND('',#1509,.T.);
#555=FACE_BOUND('',#1532,.T.);
#556=FACE_BOUND('',#1533,.T.);
#557=FACE_BOUND('',#1534,.T.);
#558=FACE_BOUND('',#1535,.T.);
#559=FACE_BOUND('',#1536,.T.);
#560=FACE_BOUND('',#1537,.T.);
#561=FACE_BOUND('',#1538,.T.);
#562=FACE_BOUND('',#1540,.T.);
#563=FACE_BOUND('',#1541,.T.);
#564=FACE_BOUND('',#1542,.T.);
#565=FACE_BOUND('',#1543,.T.);
#566=FACE_BOUND('',#1544,.T.);
#567=FACE_BOUND('',#1545,.T.);
#568=FACE_BOUND('',#1546,.T.);
#617=CONICAL_SURFACE('',#11940,5.025,0.785398163397475);
#618=CONICAL_SURFACE('',#11945,5.025,0.785398163397475);
#619=CONICAL_SURFACE('',#11950,5.025,0.785398163397463);
#620=CONICAL_SURFACE('',#11955,5.025,0.785398163397475);
#621=CONICAL_SURFACE('',#11960,5.025,0.785398163397475);
#622=CONICAL_SURFACE('',#11965,5.025,0.785398163397463);
#623=CONICAL_SURFACE('',#11971,35.5,0.785398163397469);
#624=CONICAL_SURFACE('',#11974,35.5,0.785398163397469);
#634=SPHERICAL_SURFACE('',#11914,2.5);
#635=SPHERICAL_SURFACE('',#11918,2.5);
#636=SPHERICAL_SURFACE('',#11922,2.5);
#637=SPHERICAL_SURFACE('',#11926,2.5);
#638=SPHERICAL_SURFACE('',#12223,2.5);
#639=SPHERICAL_SURFACE('',#12227,2.5);
#640=SPHERICAL_SURFACE('',#12254,2.5);
#641=SPHERICAL_SURFACE('',#12256,2.5);
#642=SPHERICAL_SURFACE('',#12259,2.5);
#643=SPHERICAL_SURFACE('',#12276,2.5);
#644=SPHERICAL_SURFACE('',#12279,2.5);
#645=SPHERICAL_SURFACE('',#12292,2.5);
#646=SPHERICAL_SURFACE('',#12317,2.5);
#647=SPHERICAL_SURFACE('',#12333,2.5);
#648=SPHERICAL_SURFACE('',#12335,2.5);
#649=SPHERICAL_SURFACE('',#12337,2.5);
#650=SPHERICAL_SURFACE('',#12340,2.5);
#651=SPHERICAL_SURFACE('',#12353,2.5);
#652=SPHERICAL_SURFACE('',#12355,2.5);
#653=SPHERICAL_SURFACE('',#12366,2.5);
#654=SPHERICAL_SURFACE('',#12369,2.5);
#655=SPHERICAL_SURFACE('',#12399,2.5);
#656=SPHERICAL_SURFACE('',#12410,2.5);
#657=SPHERICAL_SURFACE('',#12420,2.5);
#658=TOROIDAL_SURFACE('',#11899,167.5,2.5);
#659=TOROIDAL_SURFACE('',#11930,194.,1.);
#660=TOROIDAL_SURFACE('',#11935,194.,1.);
#661=TOROIDAL_SURFACE('',#12081,135.,35.);
#662=TOROIDAL_SURFACE('',#12083,210.,35.);
#663=TOROIDAL_SURFACE('',#12088,135.,35.);
#664=TOROIDAL_SURFACE('',#12090,210.,35.);
#665=TOROIDAL_SURFACE('',#12093,135.,35.);
#666=TOROIDAL_SURFACE('',#12096,250.,35.);
#667=TOROIDAL_SURFACE('',#12099,135.,35.);
#668=TOROIDAL_SURFACE('',#12102,250.,35.);
#669=TOROIDAL_SURFACE('',#12104,185.,15.);
#670=TOROIDAL_SURFACE('',#12107,185.,15.);
#671=TOROIDAL_SURFACE('',#12152,135.,25.);
#672=TOROIDAL_SURFACE('',#12154,210.,25.);
#673=TOROIDAL_SURFACE('',#12159,135.,25.);
#674=TOROIDAL_SURFACE('',#12161,210.,25.);
#675=TOROIDAL_SURFACE('',#12164,135.,25.);
#676=TOROIDAL_SURFACE('',#12167,250.,25.);
#677=TOROIDAL_SURFACE('',#12170,135.,25.);
#678=TOROIDAL_SURFACE('',#12173,250.,25.);
#679=TOROIDAL_SURFACE('',#12175,185.,25.);
#680=TOROIDAL_SURFACE('',#12178,185.,25.);
#681=TOROIDAL_SURFACE('',#12221,172.5,2.5);
#682=TOROIDAL_SURFACE('',#12231,5.,2.5);
#683=TOROIDAL_SURFACE('',#12261,5.,2.5);
#684=TOROIDAL_SURFACE('',#12264,172.5,2.5);
#685=TOROIDAL_SURFACE('',#12274,172.5,2.5);
#686=TOROIDAL_SURFACE('',#12294,5.,2.5);
#687=TOROIDAL_SURFACE('',#12297,172.5,2.5);
#688=TOROIDAL_SURFACE('',#12303,172.5,2.5);
#689=TOROIDAL_SURFACE('',#12306,5.,2.5);
#690=TOROIDAL_SURFACE('',#12316,172.5,2.5);
#691=TOROIDAL_SURFACE('',#12350,172.5,2.5);
#692=TOROIDAL_SURFACE('',#12372,172.5,2.5);
#693=TOROIDAL_SURFACE('',#12379,172.5,2.5);
#694=TOROIDAL_SURFACE('',#12382,5.,2.5);
#695=TOROIDAL_SURFACE('',#12394,5.,2.5);
#696=TOROIDAL_SURFACE('',#12396,5.,2.5);
#697=TOROIDAL_SURFACE('',#12401,172.5,2.5);
#698=TOROIDAL_SURFACE('',#12408,172.5,2.5);
#699=TOROIDAL_SURFACE('',#12411,5.,2.5);
#700=TOROIDAL_SURFACE('',#12423,172.5,2.5);
#703=FACE_OUTER_BOUND('',#1384,.T.);
#704=FACE_OUTER_BOUND('',#1385,.T.);
#705=FACE_OUTER_BOUND('',#1386,.T.);
#706=FACE_OUTER_BOUND('',#1387,.T.);
#707=FACE_OUTER_BOUND('',#1388,.T.);
#708=FACE_OUTER_BOUND('',#1389,.T.);
#709=FACE_OUTER_BOUND('',#1390,.T.);
#710=FACE_OUTER_BOUND('',#1391,.T.);
#711=FACE_OUTER_BOUND('',#1392,.T.);
#712=FACE_OUTER_BOUND('',#1393,.T.);
#713=FACE_OUTER_BOUND('',#1394,.T.);
#714=FACE_OUTER_BOUND('',#1395,.T.);
#715=FACE_OUTER_BOUND('',#1396,.T.);
#716=FACE_OUTER_BOUND('',#1397,.T.);
#717=FACE_OUTER_BOUND('',#1398,.T.);
#718=FACE_OUTER_BOUND('',#1399,.T.);
#719=FACE_OUTER_BOUND('',#1400,.T.);
#720=FACE_OUTER_BOUND('',#1401,.T.);
#721=FACE_OUTER_BOUND('',#1402,.T.);
#722=FACE_OUTER_BOUND('',#1403,.T.);
#723=FACE_OUTER_BOUND('',#1404,.T.);
#724=FACE_OUTER_BOUND('',#1405,.T.);
#725=FACE_OUTER_BOUND('',#1406,.T.);
#726=FACE_OUTER_BOUND('',#1407,.T.);
#727=FACE_OUTER_BOUND('',#1408,.T.);
#728=FACE_OUTER_BOUND('',#1409,.T.);
#729=FACE_OUTER_BOUND('',#1410,.T.);
#730=FACE_OUTER_BOUND('',#1411,.T.);
#731=FACE_OUTER_BOUND('',#1412,.T.);
#732=FACE_OUTER_BOUND('',#1413,.T.);
#733=FACE_OUTER_BOUND('',#1414,.T.);
#734=FACE_OUTER_BOUND('',#1415,.T.);
#735=FACE_OUTER_BOUND('',#1416,.T.);
#736=FACE_OUTER_BOUND('',#1417,.T.);
#737=FACE_OUTER_BOUND('',#1418,.T.);
#738=FACE_OUTER_BOUND('',#1421,.T.);
#739=FACE_OUTER_BOUND('',#1424,.T.);
#740=FACE_OUTER_BOUND('',#1427,.T.);
#741=FACE_OUTER_BOUND('',#1430,.T.);
#742=FACE_OUTER_BOUND('',#1432,.T.);
#743=FACE_OUTER_BOUND('',#1433,.T.);
#744=FACE_OUTER_BOUND('',#1434,.T.);
#745=FACE_OUTER_BOUND('',#1435,.T.);
#746=FACE_OUTER_BOUND('',#1436,.T.);
#747=FACE_OUTER_BOUND('',#1438,.T.);
#748=FACE_OUTER_BOUND('',#1439,.T.);
#749=FACE_OUTER_BOUND('',#1440,.T.);
#750=FACE_OUTER_BOUND('',#1441,.T.);
#751=FACE_OUTER_BOUND('',#1442,.T.);
#752=FACE_OUTER_BOUND('',#1443,.T.);
#753=FACE_OUTER_BOUND('',#1444,.T.);
#754=FACE_OUTER_BOUND('',#1445,.T.);
#755=FACE_OUTER_BOUND('',#1446,.T.);
#756=FACE_OUTER_BOUND('',#1447,.T.);
#757=FACE_OUTER_BOUND('',#1448,.T.);
#758=FACE_OUTER_BOUND('',#1449,.T.);
#759=FACE_OUTER_BOUND('',#1450,.T.);
#760=FACE_OUTER_BOUND('',#1451,.T.);
#761=FACE_OUTER_BOUND('',#1452,.T.);
#762=FACE_OUTER_BOUND('',#1453,.T.);
#763=FACE_OUTER_BOUND('',#1454,.T.);
#764=FACE_OUTER_BOUND('',#1455,.T.);
#765=FACE_OUTER_BOUND('',#1456,.T.);
#766=FACE_OUTER_BOUND('',#1457,.T.);
#767=FACE_OUTER_BOUND('',#1458,.T.);
#768=FACE_OUTER_BOUND('',#1459,.T.);
#769=FACE_OUTER_BOUND('',#1460,.T.);
#770=FACE_OUTER_BOUND('',#1461,.T.);
#771=FACE_OUTER_BOUND('',#1462,.T.);
#772=FACE_OUTER_BOUND('',#1463,.T.);
#773=FACE_OUTER_BOUND('',#1464,.T.);
#774=FACE_OUTER_BOUND('',#1465,.T.);
#775=FACE_OUTER_BOUND('',#1466,.T.);
#776=FACE_OUTER_BOUND('',#1467,.T.);
#777=FACE_OUTER_BOUND('',#1468,.T.);
#778=FACE_OUTER_BOUND('',#1469,.T.);
#779=FACE_OUTER_BOUND('',#1471,.T.);
#780=FACE_OUTER_BOUND('',#1472,.T.);
#781=FACE_OUTER_BOUND('',#1473,.T.);
#782=FACE_OUTER_BOUND('',#1474,.T.);
#783=FACE_OUTER_BOUND('',#1475,.T.);
#784=FACE_OUTER_BOUND('',#1476,.T.);
#785=FACE_OUTER_BOUND('',#1477,.T.);
#786=FACE_OUTER_BOUND('',#1478,.T.);
#787=FACE_OUTER_BOUND('',#1479,.T.);
#788=FACE_OUTER_BOUND('',#1480,.T.);
#789=FACE_OUTER_BOUND('',#1481,.T.);
#790=FACE_OUTER_BOUND('',#1482,.T.);
#791=FACE_OUTER_BOUND('',#1483,.T.);
#792=FACE_OUTER_BOUND('',#1484,.T.);
#793=FACE_OUTER_BOUND('',#1485,.T.);
#794=FACE_OUTER_BOUND('',#1486,.T.);
#795=FACE_OUTER_BOUND('',#1487,.T.);
#796=FACE_OUTER_BOUND('',#1488,.T.);
#797=FACE_OUTER_BOUND('',#1489,.T.);
#798=FACE_OUTER_BOUND('',#1490,.T.);
#799=FACE_OUTER_BOUND('',#1491,.T.);
#800=FACE_OUTER_BOUND('',#1492,.T.);
#801=FACE_OUTER_BOUND('',#1493,.T.);
#802=FACE_OUTER_BOUND('',#1494,.T.);
#803=FACE_OUTER_BOUND('',#1495,.T.);
#804=FACE_OUTER_BOUND('',#1496,.T.);
#805=FACE_OUTER_BOUND('',#1497,.T.);
#806=FACE_OUTER_BOUND('',#1498,.T.);
#807=FACE_OUTER_BOUND('',#1499,.T.);
#808=FACE_OUTER_BOUND('',#1500,.T.);
#809=FACE_OUTER_BOUND('',#1501,.T.);
#810=FACE_OUTER_BOUND('',#1502,.T.);
#811=FACE_OUTER_BOUND('',#1503,.T.);
#812=FACE_OUTER_BOUND('',#1504,.T.);
#813=FACE_OUTER_BOUND('',#1505,.T.);
#814=FACE_OUTER_BOUND('',#1506,.T.);
#815=FACE_OUTER_BOUND('',#1507,.T.);
#816=FACE_OUTER_BOUND('',#1510,.T.);
#817=FACE_OUTER_BOUND('',#1511,.T.);
#818=FACE_OUTER_BOUND('',#1512,.T.);
#819=FACE_OUTER_BOUND('',#1513,.T.);
#820=FACE_OUTER_BOUND('',#1514,.T.);
#821=FACE_OUTER_BOUND('',#1515,.T.);
#822=FACE_OUTER_BOUND('',#1516,.T.);
#823=FACE_OUTER_BOUND('',#1517,.T.);
#824=FACE_OUTER_BOUND('',#1518,.T.);
#825=FACE_OUTER_BOUND('',#1519,.T.);
#826=FACE_OUTER_BOUND('',#1520,.T.);
#827=FACE_OUTER_BOUND('',#1521,.T.);
#828=FACE_OUTER_BOUND('',#1522,.T.);
#829=FACE_OUTER_BOUND('',#1523,.T.);
#830=FACE_OUTER_BOUND('',#1524,.T.);
#831=FACE_OUTER_BOUND('',#1525,.T.);
#832=FACE_OUTER_BOUND('',#1526,.T.);
#833=FACE_OUTER_BOUND('',#1527,.T.);
#834=FACE_OUTER_BOUND('',#1528,.T.);
#835=FACE_OUTER_BOUND('',#1529,.T.);
#836=FACE_OUTER_BOUND('',#1530,.T.);
#837=FACE_OUTER_BOUND('',#1531,.T.);
#838=FACE_OUTER_BOUND('',#1539,.T.);
#839=FACE_OUTER_BOUND('',#1547,.T.);
#840=FACE_OUTER_BOUND('',#1548,.T.);
#841=FACE_OUTER_BOUND('',#1549,.T.);
#842=FACE_OUTER_BOUND('',#1550,.T.);
#843=FACE_OUTER_BOUND('',#1551,.T.);
#844=FACE_OUTER_BOUND('',#1552,.T.);
#845=FACE_OUTER_BOUND('',#1553,.T.);
#846=FACE_OUTER_BOUND('',#1554,.T.);
#847=FACE_OUTER_BOUND('',#1555,.T.);
#848=FACE_OUTER_BOUND('',#1556,.T.);
#849=FACE_OUTER_BOUND('',#1557,.T.);
#850=FACE_OUTER_BOUND('',#1558,.T.);
#851=FACE_OUTER_BOUND('',#1559,.T.);
#852=FACE_OUTER_BOUND('',#1560,.T.);
#853=FACE_OUTER_BOUND('',#1561,.T.);
#854=FACE_OUTER_BOUND('',#1562,.T.);
#855=FACE_OUTER_BOUND('',#1563,.T.);
#856=FACE_OUTER_BOUND('',#1564,.T.);
#857=FACE_OUTER_BOUND('',#1565,.T.);
#858=FACE_OUTER_BOUND('',#1566,.T.);
#859=FACE_OUTER_BOUND('',#1567,.T.);
#860=FACE_OUTER_BOUND('',#1568,.T.);
#861=FACE_OUTER_BOUND('',#1569,.T.);
#862=FACE_OUTER_BOUND('',#1570,.T.);
#863=FACE_OUTER_BOUND('',#1571,.T.);
#864=FACE_OUTER_BOUND('',#1572,.T.);
#865=FACE_OUTER_BOUND('',#1573,.T.);
#866=FACE_OUTER_BOUND('',#1574,.T.);
#867=FACE_OUTER_BOUND('',#1575,.T.);
#868=FACE_OUTER_BOUND('',#1576,.T.);
#869=FACE_OUTER_BOUND('',#1577,.T.);
#870=FACE_OUTER_BOUND('',#1578,.T.);
#871=FACE_OUTER_BOUND('',#1579,.T.);
#872=FACE_OUTER_BOUND('',#1580,.T.);
#873=FACE_OUTER_BOUND('',#1581,.T.);
#874=FACE_OUTER_BOUND('',#1582,.T.);
#875=FACE_OUTER_BOUND('',#1583,.T.);
#876=FACE_OUTER_BOUND('',#1584,.T.);
#877=FACE_OUTER_BOUND('',#1585,.T.);
#878=FACE_OUTER_BOUND('',#1586,.T.);
#879=FACE_OUTER_BOUND('',#1587,.T.);
#880=FACE_OUTER_BOUND('',#1588,.T.);
#881=FACE_OUTER_BOUND('',#1589,.T.);
#882=FACE_OUTER_BOUND('',#1590,.T.);
#883=FACE_OUTER_BOUND('',#1591,.T.);
#884=FACE_OUTER_BOUND('',#1592,.T.);
#885=FACE_OUTER_BOUND('',#1593,.T.);
#886=FACE_OUTER_BOUND('',#1594,.T.);
#887=FACE_OUTER_BOUND('',#1595,.T.);
#888=FACE_OUTER_BOUND('',#1596,.T.);
#889=FACE_OUTER_BOUND('',#1597,.T.);
#890=FACE_OUTER_BOUND('',#1598,.T.);
#891=FACE_OUTER_BOUND('',#1599,.T.);
#892=FACE_OUTER_BOUND('',#1600,.T.);
#893=FACE_OUTER_BOUND('',#1601,.T.);
#894=FACE_OUTER_BOUND('',#1602,.T.);
#895=FACE_OUTER_BOUND('',#1603,.T.);
#896=FACE_OUTER_BOUND('',#1604,.T.);
#897=FACE_OUTER_BOUND('',#1605,.T.);
#898=FACE_OUTER_BOUND('',#1606,.T.);
#899=FACE_OUTER_BOUND('',#1607,.T.);
#900=FACE_OUTER_BOUND('',#1608,.T.);
#901=FACE_OUTER_BOUND('',#1609,.T.);
#902=FACE_OUTER_BOUND('',#1610,.T.);
#903=FACE_OUTER_BOUND('',#1611,.T.);
#904=FACE_OUTER_BOUND('',#1612,.T.);
#905=FACE_OUTER_BOUND('',#1613,.T.);
#906=FACE_OUTER_BOUND('',#1614,.T.);
#907=FACE_OUTER_BOUND('',#1615,.T.);
#908=FACE_OUTER_BOUND('',#1616,.T.);
#909=FACE_OUTER_BOUND('',#1617,.T.);
#910=FACE_OUTER_BOUND('',#1618,.T.);
#911=FACE_OUTER_BOUND('',#1619,.T.);
#912=FACE_OUTER_BOUND('',#1620,.T.);
#913=FACE_OUTER_BOUND('',#1621,.T.);
#914=FACE_OUTER_BOUND('',#1622,.T.);
#915=FACE_OUTER_BOUND('',#1623,.T.);
#916=FACE_OUTER_BOUND('',#1624,.T.);
#917=FACE_OUTER_BOUND('',#1625,.T.);
#918=FACE_OUTER_BOUND('',#1626,.T.);
#919=FACE_OUTER_BOUND('',#1627,.T.);
#920=FACE_OUTER_BOUND('',#1628,.T.);
#921=FACE_OUTER_BOUND('',#1629,.T.);
#922=FACE_OUTER_BOUND('',#1630,.T.);
#923=FACE_OUTER_BOUND('',#1631,.T.);
#924=FACE_OUTER_BOUND('',#1632,.T.);
#925=FACE_OUTER_BOUND('',#1633,.T.);
#926=FACE_OUTER_BOUND('',#1634,.T.);
#927=FACE_OUTER_BOUND('',#1635,.T.);
#928=FACE_OUTER_BOUND('',#1636,.T.);
#929=FACE_OUTER_BOUND('',#1637,.T.);
#930=FACE_OUTER_BOUND('',#1638,.T.);
#931=FACE_OUTER_BOUND('',#1639,.T.);
#932=FACE_OUTER_BOUND('',#1640,.T.);
#933=FACE_OUTER_BOUND('',#1641,.T.);
#934=FACE_OUTER_BOUND('',#1642,.T.);
#935=FACE_OUTER_BOUND('',#1643,.T.);
#936=FACE_OUTER_BOUND('',#1644,.T.);
#937=FACE_OUTER_BOUND('',#1645,.T.);
#938=FACE_OUTER_BOUND('',#1646,.T.);
#939=FACE_OUTER_BOUND('',#1647,.T.);
#940=FACE_OUTER_BOUND('',#1648,.T.);
#941=FACE_OUTER_BOUND('',#1649,.T.);
#942=FACE_OUTER_BOUND('',#1650,.T.);
#943=FACE_OUTER_BOUND('',#1651,.T.);
#944=FACE_OUTER_BOUND('',#1652,.T.);
#945=FACE_OUTER_BOUND('',#1653,.T.);
#946=FACE_OUTER_BOUND('',#1654,.T.);
#947=FACE_OUTER_BOUND('',#1655,.T.);
#948=FACE_OUTER_BOUND('',#1656,.T.);
#949=FACE_OUTER_BOUND('',#1657,.T.);
#950=FACE_OUTER_BOUND('',#1658,.T.);
#951=FACE_OUTER_BOUND('',#1659,.T.);
#1384=EDGE_LOOP('',(#7528,#7529,#7530));
#1385=EDGE_LOOP('',(#7531,#7532,#7533,#7534,#7535));
#1386=EDGE_LOOP('',(#7536,#7537,#7538,#7539));
#1387=EDGE_LOOP('',(#7540,#7541,#7542,#7543,#7544));
#1388=EDGE_LOOP('',(#7545,#7546,#7547,#7548));
#1389=EDGE_LOOP('',(#7549,#7550,#7551));
#1390=EDGE_LOOP('',(#7552,#7553,#7554));
#1391=EDGE_LOOP('',(#7555,#7556,#7557));
#1392=EDGE_LOOP('',(#7558,#7559,#7560));
#1393=EDGE_LOOP('',(#7561,#7562,#7563,#7564,#7565));
#1394=EDGE_LOOP('',(#7566,#7567,#7568,#7569,#7570));
#1395=EDGE_LOOP('',(#7571,#7572,#7573,#7574));
#1396=EDGE_LOOP('',(#7575,#7576,#7577,#7578));
#1397=EDGE_LOOP('',(#7579,#7580,#7581,#7582));
#1398=EDGE_LOOP('',(#7583,#7584,#7585,#7586));
#1399=EDGE_LOOP('',(#7587,#7588,#7589,#7590));
#1400=EDGE_LOOP('',(#7591,#7592,#7593,#7594));
#1401=EDGE_LOOP('',(#7595,#7596,#7597,#7598));
#1402=EDGE_LOOP('',(#7599,#7600,#7601,#7602));
#1403=EDGE_LOOP('',(#7603,#7604,#7605,#7606));
#1404=EDGE_LOOP('',(#7607,#7608,#7609,#7610));
#1405=EDGE_LOOP('',(#7611,#7612,#7613,#7614));
#1406=EDGE_LOOP('',(#7615,#7616,#7617,#7618));
#1407=EDGE_LOOP('',(#7619,#7620,#7621,#7622,#7623,#7624));
#1408=EDGE_LOOP('',(#7625,#7626,#7627,#7628));
#1409=EDGE_LOOP('',(#7629,#7630,#7631,#7632,#7633));
#1410=EDGE_LOOP('',(#7634,#7635,#7636,#7637,#7638));
#1411=EDGE_LOOP('',(#7639,#7640,#7641,#7642));
#1412=EDGE_LOOP('',(#7643,#7644,#7645,#7646));
#1413=EDGE_LOOP('',(#7647,#7648,#7649,#7650));
#1414=EDGE_LOOP('',(#7651,#7652,#7653,#7654));
#1415=EDGE_LOOP('',(#7655,#7656,#7657,#7658));
#1416=EDGE_LOOP('',(#7659,#7660,#7661,#7662,#7663,#7664,#7665,#7666,#7667,
#7668,#7669));
#1417=EDGE_LOOP('',(#7670,#7671,#7672,#7673,#7674,#7675));
#1418=EDGE_LOOP('',(#7676,#7677,#7678,#7679,#7680,#7681,#7682,#7683,#7684,
#7685,#7686,#7687,#7688,#7689,#7690));
#1419=EDGE_LOOP('',(#7691,#7692,#7693,#7694,#7695,#7696,#7697,#7698,#7699,
#7700,#7701,#7702,#7703,#7704,#7705,#7706,#7707,#7708,#7709,#7710));
#1420=EDGE_LOOP('',(#7711,#7712,#7713,#7714,#7715,#7716,#7717,#7718,#7719,
#7720,#7721,#7722,#7723,#7724,#7725,#7726,#7727,#7728,#7729,#7730));
#1421=EDGE_LOOP('',(#7731,#7732,#7733,#7734,#7735,#7736));
#1422=EDGE_LOOP('',(#7737));
#1423=EDGE_LOOP('',(#7738));
#1424=EDGE_LOOP('',(#7739,#7740,#7741,#7742,#7743,#7744,#7745,#7746,#7747,
#7748,#7749,#7750,#7751,#7752,#7753,#7754,#7755,#7756));
#1425=EDGE_LOOP('',(#7757));
#1426=EDGE_LOOP('',(#7758));
#1427=EDGE_LOOP('',(#7759,#7760,#7761,#7762,#7763,#7764,#7765,#7766,#7767,
#7768,#7769,#7770,#7771,#7772,#7773,#7774,#7775,#7776));
#1428=EDGE_LOOP('',(#7777));
#1429=EDGE_LOOP('',(#7778));
#1430=EDGE_LOOP('',(#7779));
#1431=EDGE_LOOP('',(#7780));
#1432=EDGE_LOOP('',(#7781,#7782,#7783,#7784));
#1433=EDGE_LOOP('',(#7785,#7786,#7787,#7788,#7789));
#1434=EDGE_LOOP('',(#7790,#7791,#7792,#7793,#7794,#7795));
#1435=EDGE_LOOP('',(#7796,#7797,#7798,#7799,#7800));
#1436=EDGE_LOOP('',(#7801,#7802,#7803,#7804,#7805,#7806,#7807,#7808));
#1437=EDGE_LOOP('',(#7809,#7810,#7811,#7812,#7813,#7814,#7815,#7816));
#1438=EDGE_LOOP('',(#7817,#7818,#7819,#7820,#7821,#7822));
#1439=EDGE_LOOP('',(#7823,#7824,#7825,#7826,#7827));
#1440=EDGE_LOOP('',(#7828,#7829,#7830,#7831,#7832));
#1441=EDGE_LOOP('',(#7833,#7834,#7835,#7836));
#1442=EDGE_LOOP('',(#7837,#7838,#7839,#7840,#7841));
#1443=EDGE_LOOP('',(#7842,#7843,#7844,#7845,#7846,#7847,#7848,#7849));
#1444=EDGE_LOOP('',(#7850,#7851,#7852,#7853,#7854));
#1445=EDGE_LOOP('',(#7855,#7856,#7857,#7858));
#1446=EDGE_LOOP('',(#7859,#7860,#7861,#7862));
#1447=EDGE_LOOP('',(#7863,#7864,#7865,#7866));
#1448=EDGE_LOOP('',(#7867,#7868,#7869,#7870));
#1449=EDGE_LOOP('',(#7871,#7872,#7873,#7874));
#1450=EDGE_LOOP('',(#7875,#7876,#7877,#7878));
#1451=EDGE_LOOP('',(#7879,#7880,#7881,#7882));
#1452=EDGE_LOOP('',(#7883,#7884,#7885,#7886));
#1453=EDGE_LOOP('',(#7887,#7888,#7889,#7890));
#1454=EDGE_LOOP('',(#7891,#7892,#7893,#7894));
#1455=EDGE_LOOP('',(#7895,#7896,#7897,#7898));
#1456=EDGE_LOOP('',(#7899,#7900,#7901,#7902));
#1457=EDGE_LOOP('',(#7903,#7904,#7905,#7906));
#1458=EDGE_LOOP('',(#7907,#7908,#7909,#7910));
#1459=EDGE_LOOP('',(#7911,#7912,#7913,#7914));
#1460=EDGE_LOOP('',(#7915,#7916,#7917,#7918));
#1461=EDGE_LOOP('',(#7919,#7920,#7921,#7922));
#1462=EDGE_LOOP('',(#7923,#7924,#7925,#7926));
#1463=EDGE_LOOP('',(#7927,#7928,#7929));
#1464=EDGE_LOOP('',(#7930,#7931,#7932,#7933));
#1465=EDGE_LOOP('',(#7934,#7935,#7936,#7937,#7938));
#1466=EDGE_LOOP('',(#7939,#7940,#7941,#7942,#7943));
#1467=EDGE_LOOP('',(#7944,#7945,#7946,#7947));
#1468=EDGE_LOOP('',(#7948,#7949,#7950));
#1469=EDGE_LOOP('',(#7951,#7952,#7953));
#1470=EDGE_LOOP('',(#7954));
#1471=EDGE_LOOP('',(#7955,#7956,#7957,#7958));
#1472=EDGE_LOOP('',(#7959,#7960,#7961,#7962,#7963));
#1473=EDGE_LOOP('',(#7964,#7965,#7966,#7967,#7968,#7969));
#1474=EDGE_LOOP('',(#7970,#7971,#7972,#7973,#7974));
#1475=EDGE_LOOP('',(#7975,#7976,#7977,#7978,#7979,#7980));
#1476=EDGE_LOOP('',(#7981,#7982,#7983,#7984,#7985));
#1477=EDGE_LOOP('',(#7986,#7987,#7988,#7989,#7990));
#1478=EDGE_LOOP('',(#7991,#7992,#7993,#7994));
#1479=EDGE_LOOP('',(#7995,#7996,#7997,#7998,#7999));
#1480=EDGE_LOOP('',(#8000,#8001,#8002,#8003,#8004,#8005,#8006,#8007));
#1481=EDGE_LOOP('',(#8008,#8009,#8010,#8011,#8012));
#1482=EDGE_LOOP('',(#8013,#8014,#8015,#8016));
#1483=EDGE_LOOP('',(#8017,#8018,#8019,#8020));
#1484=EDGE_LOOP('',(#8021,#8022,#8023,#8024));
#1485=EDGE_LOOP('',(#8025,#8026,#8027,#8028));
#1486=EDGE_LOOP('',(#8029,#8030,#8031,#8032));
#1487=EDGE_LOOP('',(#8033,#8034,#8035,#8036));
#1488=EDGE_LOOP('',(#8037,#8038,#8039,#8040));
#1489=EDGE_LOOP('',(#8041,#8042,#8043,#8044));
#1490=EDGE_LOOP('',(#8045,#8046,#8047,#8048));
#1491=EDGE_LOOP('',(#8049,#8050,#8051,#8052));
#1492=EDGE_LOOP('',(#8053,#8054,#8055,#8056));
#1493=EDGE_LOOP('',(#8057,#8058,#8059,#8060));
#1494=EDGE_LOOP('',(#8061,#8062,#8063,#8064));
#1495=EDGE_LOOP('',(#8065,#8066,#8067,#8068));
#1496=EDGE_LOOP('',(#8069,#8070,#8071,#8072));
#1497=EDGE_LOOP('',(#8073,#8074,#8075,#8076));
#1498=EDGE_LOOP('',(#8077,#8078,#8079,#8080));
#1499=EDGE_LOOP('',(#8081,#8082,#8083,#8084));
#1500=EDGE_LOOP('',(#8085,#8086,#8087));
#1501=EDGE_LOOP('',(#8088,#8089,#8090,#8091));
#1502=EDGE_LOOP('',(#8092,#8093,#8094,#8095));
#1503=EDGE_LOOP('',(#8096,#8097,#8098,#8099));
#1504=EDGE_LOOP('',(#8100,#8101,#8102,#8103));
#1505=EDGE_LOOP('',(#8104,#8105,#8106));
#1506=EDGE_LOOP('',(#8107,#8108,#8109,#8110));
#1507=EDGE_LOOP('',(#8111,#8112,#8113,#8114,#8115,#8116));
#1508=EDGE_LOOP('',(#8117));
#1509=EDGE_LOOP('',(#8118));
#1510=EDGE_LOOP('',(#8119,#8120,#8121,#8122));
#1511=EDGE_LOOP('',(#8123,#8124,#8125,#8126));
#1512=EDGE_LOOP('',(#8127,#8128,#8129,#8130));
#1513=EDGE_LOOP('',(#8131,#8132,#8133));
#1514=EDGE_LOOP('',(#8134,#8135,#8136));
#1515=EDGE_LOOP('',(#8137,#8138,#8139,#8140));
#1516=EDGE_LOOP('',(#8141,#8142,#8143));
#1517=EDGE_LOOP('',(#8144,#8145,#8146));
#1518=EDGE_LOOP('',(#8147,#8148,#8149,#8150));
#1519=EDGE_LOOP('',(#8151,#8152,#8153,#8154));
#1520=EDGE_LOOP('',(#8155,#8156,#8157,#8158));
#1521=EDGE_LOOP('',(#8159,#8160,#8161,#8162));
#1522=EDGE_LOOP('',(#8163,#8164,#8165));
#1523=EDGE_LOOP('',(#8166,#8167,#8168));
#1524=EDGE_LOOP('',(#8169,#8170,#8171,#8172));
#1525=EDGE_LOOP('',(#8173,#8174,#8175));
#1526=EDGE_LOOP('',(#8176,#8177,#8178));
#1527=EDGE_LOOP('',(#8179,#8180,#8181,#8182));
#1528=EDGE_LOOP('',(#8183,#8184,#8185,#8186));
#1529=EDGE_LOOP('',(#8187,#8188,#8189,#8190));
#1530=EDGE_LOOP('',(#8191,#8192,#8193,#8194));
#1531=EDGE_LOOP('',(#8195));
#1532=EDGE_LOOP('',(#8196));
#1533=EDGE_LOOP('',(#8197));
#1534=EDGE_LOOP('',(#8198));
#1535=EDGE_LOOP('',(#8199));
#1536=EDGE_LOOP('',(#8200));
#1537=EDGE_LOOP('',(#8201));
#1538=EDGE_LOOP('',(#8202));
#1539=EDGE_LOOP('',(#8203));
#1540=EDGE_LOOP('',(#8204));
#1541=EDGE_LOOP('',(#8205));
#1542=EDGE_LOOP('',(#8206));
#1543=EDGE_LOOP('',(#8207));
#1544=EDGE_LOOP('',(#8208));
#1545=EDGE_LOOP('',(#8209));
#1546=EDGE_LOOP('',(#8210));
#1547=EDGE_LOOP('',(#8211,#8212,#8213,#8214));
#1548=EDGE_LOOP('',(#8215,#8216,#8217,#8218));
#1549=EDGE_LOOP('',(#8219,#8220,#8221,#8222));
#1550=EDGE_LOOP('',(#8223,#8224,#8225));
#1551=EDGE_LOOP('',(#8226,#8227,#8228));
#1552=EDGE_LOOP('',(#8229,#8230,#8231,#8232));
#1553=EDGE_LOOP('',(#8233,#8234,#8235,#8236));
#1554=EDGE_LOOP('',(#8237,#8238,#8239,#8240));
#1555=EDGE_LOOP('',(#8241,#8242,#8243,#8244));
#1556=EDGE_LOOP('',(#8245,#8246,#8247,#8248));
#1557=EDGE_LOOP('',(#8249,#8250,#8251,#8252));
#1558=EDGE_LOOP('',(#8253,#8254,#8255,#8256));
#1559=EDGE_LOOP('',(#8257,#8258,#8259,#8260));
#1560=EDGE_LOOP('',(#8261,#8262,#8263,#8264));
#1561=EDGE_LOOP('',(#8265,#8266,#8267,#8268));
#1562=EDGE_LOOP('',(#8269,#8270,#8271,#8272));
#1563=EDGE_LOOP('',(#8273,#8274,#8275,#8276));
#1564=EDGE_LOOP('',(#8277,#8278,#8279,#8280));
#1565=EDGE_LOOP('',(#8281,#8282,#8283));
#1566=EDGE_LOOP('',(#8284,#8285,#8286));
#1567=EDGE_LOOP('',(#8287,#8288,#8289));
#1568=EDGE_LOOP('',(#8290,#8291,#8292,#8293));
#1569=EDGE_LOOP('',(#8294,#8295,#8296,#8297));
#1570=EDGE_LOOP('',(#8298,#8299,#8300,#8301));
#1571=EDGE_LOOP('',(#8302,#8303,#8304,#8305));
#1572=EDGE_LOOP('',(#8306,#8307,#8308,#8309));
#1573=EDGE_LOOP('',(#8310,#8311,#8312,#8313));
#1574=EDGE_LOOP('',(#8314,#8315,#8316,#8317));
#1575=EDGE_LOOP('',(#8318,#8319,#8320,#8321));
#1576=EDGE_LOOP('',(#8322,#8323,#8324,#8325));
#1577=EDGE_LOOP('',(#8326,#8327,#8328,#8329));
#1578=EDGE_LOOP('',(#8330,#8331,#8332));
#1579=EDGE_LOOP('',(#8333,#8334,#8335));
#1580=EDGE_LOOP('',(#8336,#8337,#8338,#8339));
#1581=EDGE_LOOP('',(#8340,#8341,#8342,#8343));
#1582=EDGE_LOOP('',(#8344,#8345,#8346,#8347));
#1583=EDGE_LOOP('',(#8348,#8349,#8350,#8351));
#1584=EDGE_LOOP('',(#8352,#8353,#8354,#8355));
#1585=EDGE_LOOP('',(#8356,#8357,#8358,#8359));
#1586=EDGE_LOOP('',(#8360,#8361,#8362,#8363));
#1587=EDGE_LOOP('',(#8364,#8365,#8366));
#1588=EDGE_LOOP('',(#8367,#8368,#8369,#8370));
#1589=EDGE_LOOP('',(#8371,#8372,#8373,#8374));
#1590=EDGE_LOOP('',(#8375,#8376,#8377,#8378));
#1591=EDGE_LOOP('',(#8379,#8380,#8381,#8382));
#1592=EDGE_LOOP('',(#8383,#8384,#8385,#8386));
#1593=EDGE_LOOP('',(#8387,#8388,#8389,#8390));
#1594=EDGE_LOOP('',(#8391,#8392,#8393,#8394));
#1595=EDGE_LOOP('',(#8395,#8396,#8397,#8398));
#1596=EDGE_LOOP('',(#8399,#8400,#8401,#8402));
#1597=EDGE_LOOP('',(#8403,#8404,#8405,#8406));
#1598=EDGE_LOOP('',(#8407,#8408,#8409,#8410));
#1599=EDGE_LOOP('',(#8411,#8412,#8413,#8414));
#1600=EDGE_LOOP('',(#8415,#8416,#8417,#8418));
#1601=EDGE_LOOP('',(#8419,#8420,#8421,#8422));
#1602=EDGE_LOOP('',(#8423,#8424,#8425,#8426));
#1603=EDGE_LOOP('',(#8427,#8428,#8429));
#1604=EDGE_LOOP('',(#8430,#8431,#8432,#8433));
#1605=EDGE_LOOP('',(#8434,#8435,#8436,#8437));
#1606=EDGE_LOOP('',(#8438,#8439,#8440,#8441));
#1607=EDGE_LOOP('',(#8442,#8443,#8444,#8445));
#1608=EDGE_LOOP('',(#8446,#8447,#8448,#8449));
#1609=EDGE_LOOP('',(#8450,#8451,#8452));
#1610=EDGE_LOOP('',(#8453,#8454,#8455));
#1611=EDGE_LOOP('',(#8456,#8457,#8458));
#1612=EDGE_LOOP('',(#8459,#8460,#8461));
#1613=EDGE_LOOP('',(#8462,#8463,#8464,#8465));
#1614=EDGE_LOOP('',(#8466,#8467,#8468,#8469));
#1615=EDGE_LOOP('',(#8470,#8471,#8472,#8473));
#1616=EDGE_LOOP('',(#8474,#8475,#8476,#8477));
#1617=EDGE_LOOP('',(#8478,#8479,#8480,#8481));
#1618=EDGE_LOOP('',(#8482,#8483,#8484,#8485));
#1619=EDGE_LOOP('',(#8486,#8487,#8488,#8489));
#1620=EDGE_LOOP('',(#8490,#8491,#8492));
#1621=EDGE_LOOP('',(#8493,#8494,#8495));
#1622=EDGE_LOOP('',(#8496,#8497,#8498,#8499));
#1623=EDGE_LOOP('',(#8500,#8501,#8502,#8503));
#1624=EDGE_LOOP('',(#8504,#8505,#8506,#8507));
#1625=EDGE_LOOP('',(#8508,#8509,#8510,#8511));
#1626=EDGE_LOOP('',(#8512,#8513,#8514,#8515));
#1627=EDGE_LOOP('',(#8516,#8517,#8518));
#1628=EDGE_LOOP('',(#8519,#8520,#8521));
#1629=EDGE_LOOP('',(#8522,#8523,#8524,#8525));
#1630=EDGE_LOOP('',(#8526,#8527,#8528,#8529));
#1631=EDGE_LOOP('',(#8530,#8531,#8532,#8533));
#1632=EDGE_LOOP('',(#8534,#8535,#8536,#8537));
#1633=EDGE_LOOP('',(#8538,#8539,#8540,#8541));
#1634=EDGE_LOOP('',(#8542,#8543,#8544,#8545));
#1635=EDGE_LOOP('',(#8546,#8547,#8548,#8549));
#1636=EDGE_LOOP('',(#8550,#8551,#8552,#8553));
#1637=EDGE_LOOP('',(#8554,#8555,#8556,#8557,#8558));
#1638=EDGE_LOOP('',(#8559,#8560,#8561,#8562));
#1639=EDGE_LOOP('',(#8563,#8564,#8565,#8566));
#1640=EDGE_LOOP('',(#8567,#8568,#8569,#8570));
#1641=EDGE_LOOP('',(#8571,#8572,#8573,#8574));
#1642=EDGE_LOOP('',(#8575,#8576,#8577,#8578));
#1643=EDGE_LOOP('',(#8579,#8580,#8581,#8582));
#1644=EDGE_LOOP('',(#8583,#8584,#8585,#8586));
#1645=EDGE_LOOP('',(#8587,#8588,#8589));
#1646=EDGE_LOOP('',(#8590,#8591,#8592,#8593));
#1647=EDGE_LOOP('',(#8594,#8595,#8596,#8597));
#1648=EDGE_LOOP('',(#8598,#8599,#8600,#8601));
#1649=EDGE_LOOP('',(#8602,#8603,#8604,#8605));
#1650=EDGE_LOOP('',(#8606,#8607,#8608,#8609));
#1651=EDGE_LOOP('',(#8610,#8611,#8612));
#1652=EDGE_LOOP('',(#8613,#8614,#8615,#8616));
#1653=EDGE_LOOP('',(#8617,#8618,#8619,#8620));
#1654=EDGE_LOOP('',(#8621,#8622,#8623,#8624));
#1655=EDGE_LOOP('',(#8625,#8626,#8627,#8628));
#1656=EDGE_LOOP('',(#8629,#8630,#8631,#8632));
#1657=EDGE_LOOP('',(#8633,#8634,#8635));
#1658=EDGE_LOOP('',(#8636,#8637,#8638,#8639));
#1659=EDGE_LOOP('',(#8640,#8641,#8642,#8643));
#2140=CIRCLE('',#11898,160.);
#2141=CIRCLE('',#11900,170.);
#2142=CIRCLE('',#11901,170.);
#2143=CIRCLE('',#11902,2.5);
#2144=CIRCLE('',#11903,167.5);
#2145=CIRCLE('',#11905,2.5);
#2146=CIRCLE('',#11906,2.5);
#2147=CIRCLE('',#11908,2.5);
#2148=CIRCLE('',#11909,2.5);
#2149=CIRCLE('',#11910,2.5);
#2150=CIRCLE('',#11912,2.5);
#2151=CIRCLE('',#11913,2.5);
#2152=CIRCLE('',#11915,2.5);
#2153=CIRCLE('',#11916,2.5);
#2154=CIRCLE('',#11917,2.5);
#2155=CIRCLE('',#11919,2.5);
#2156=CIRCLE('',#11920,2.5);
#2157=CIRCLE('',#11921,2.49999999999999);
#2158=CIRCLE('',#11923,2.5);
#2159=CIRCLE('',#11924,2.5);
#2160=CIRCLE('',#11925,2.5);
#2161=CIRCLE('',#11927,2.5);
#2162=CIRCLE('',#11928,2.5);
#2163=CIRCLE('',#11929,2.49999999999999);
#2164=CIRCLE('',#11931,194.);
#2165=CIRCLE('',#11932,1.);
#2166=CIRCLE('',#11933,195.);
#2167=CIRCLE('',#11934,195.);
#2168=CIRCLE('',#11936,195.);
#2169=CIRCLE('',#11937,195.);
#2170=CIRCLE('',#11938,1.);
#2171=CIRCLE('',#11939,194.);
#2172=CIRCLE('',#11941,4.49999999999998);
#2173=CIRCLE('',#11942,5.025);
#2174=CIRCLE('',#11944,4.49999999999998);
#2175=CIRCLE('',#11946,4.49999999999998);
#2176=CIRCLE('',#11947,5.025);
#2177=CIRCLE('',#11949,4.49999999999998);
#2178=CIRCLE('',#11951,4.49999999999999);
#2179=CIRCLE('',#11952,5.025);
#2180=CIRCLE('',#11954,4.49999999999997);
#2181=CIRCLE('',#11956,4.49999999999998);
#2182=CIRCLE('',#11957,5.025);
#2183=CIRCLE('',#11959,4.49999999999998);
#2184=CIRCLE('',#11961,4.49999999999998);
#2185=CIRCLE('',#11962,5.025);
#2186=CIRCLE('',#11964,4.49999999999998);
#2187=CIRCLE('',#11966,4.49999999999999);
#2188=CIRCLE('',#11967,5.025);
#2189=CIRCLE('',#11969,4.49999999999998);
#2190=CIRCLE('',#11972,35.5);
#2191=CIRCLE('',#11973,37.5);
#2192=CIRCLE('',#11975,35.5);
#2193=CIRCLE('',#11976,35.5);
#2194=CIRCLE('',#11977,37.5);
#2195=CIRCLE('',#11980,4.5);
#2196=CIRCLE('',#11981,4.5);
#2197=CIRCLE('',#11983,4.5);
#2198=CIRCLE('',#11984,4.5);
#2199=CIRCLE('',#11986,4.5);
#2200=CIRCLE('',#11987,4.5);
#2201=CIRCLE('',#11989,4.5);
#2202=CIRCLE('',#11990,4.5);
#2203=CIRCLE('',#11992,25.);
#2204=CIRCLE('',#11993,25.);
#2205=CIRCLE('',#11995,160.);
#2206=CIRCLE('',#11996,160.);
#2207=CIRCLE('',#11997,160.);
#2208=CIRCLE('',#11999,15.);
#2209=CIRCLE('',#12000,15.);
#2210=CIRCLE('',#12001,15.);
#2211=CIRCLE('',#12002,15.);
#2212=CIRCLE('',#12004,170.);
#2213=CIRCLE('',#12005,170.);
#2214=CIRCLE('',#12006,170.);
#2215=CIRCLE('',#12007,170.);
#2216=CIRCLE('',#12008,170.);
#2217=CIRCLE('',#12009,170.);
#2218=CIRCLE('',#12010,170.);
#2219=CIRCLE('',#12011,170.);
#2220=CIRCLE('',#12012,170.);
#2221=CIRCLE('',#12013,170.);
#2222=CIRCLE('',#12014,170.);
#2223=CIRCLE('',#12015,170.);
#2224=CIRCLE('',#12016,170.);
#2225=CIRCLE('',#12017,170.);
#2226=CIRCLE('',#12018,170.);
#2227=CIRCLE('',#12021,5.);
#2228=CIRCLE('',#12022,5.);
#2229=CIRCLE('',#12023,5.);
#2230=CIRCLE('',#12024,5.);
#2231=CIRCLE('',#12026,5.);
#2232=CIRCLE('',#12027,5.);
#2233=CIRCLE('',#12028,5.);
#2234=CIRCLE('',#12029,5.);
#2235=CIRCLE('',#12032,175.);
#2236=CIRCLE('',#12033,175.);
#2237=CIRCLE('',#12035,210.);
#2238=CIRCLE('',#12036,185.);
#2239=CIRCLE('',#12037,250.);
#2240=CIRCLE('',#12038,135.);
#2241=CIRCLE('',#12040,285.);
#2242=CIRCLE('',#12041,149.388176775342);
#2243=CIRCLE('',#12042,149.388176775134);
#2244=CIRCLE('',#12043,285.);
#2245=CIRCLE('',#12045,250.);
#2246=CIRCLE('',#12046,185.);
#2247=CIRCLE('',#12047,210.);
#2248=CIRCLE('',#12048,135.);
#2249=CIRCLE('',#12059,135.);
#2250=CIRCLE('',#12060,135.);
#2251=CIRCLE('',#12062,137.537590041004);
#2252=CIRCLE('',#12064,137.53759018693);
#2253=CIRCLE('',#12067,80.8416395220943);
#2254=CIRCLE('',#12068,100.);
#2255=CIRCLE('',#12070,100.);
#2256=CIRCLE('',#12071,100.);
#2257=CIRCLE('',#12072,103.415458265314);
#2258=CIRCLE('',#12073,103.415458265742);
#2259=CIRCLE('',#12075,100.);
#2260=CIRCLE('',#12076,80.8416395221478);
#2261=CIRCLE('',#12078,35.);
#2262=CIRCLE('',#12079,35.);
#2263=CIRCLE('',#12080,35.);
#2264=CIRCLE('',#12082,35.);
#2265=CIRCLE('',#12085,35.);
#2266=CIRCLE('',#12086,35.);
#2267=CIRCLE('',#12087,35.);
#2268=CIRCLE('',#12089,35.);
#2269=CIRCLE('',#12092,35.);
#2270=CIRCLE('',#12094,35.);
#2271=CIRCLE('',#12095,35.);
#2272=CIRCLE('',#12098,35.);
#2273=CIRCLE('',#12100,35.);
#2274=CIRCLE('',#12101,35.);
#2275=CIRCLE('',#12103,15.);
#2276=CIRCLE('',#12105,15.);
#2277=CIRCLE('',#12106,15.);
#2278=CIRCLE('',#12108,15.);
#2279=CIRCLE('',#12110,160.);
#2280=CIRCLE('',#12112,185.);
#2281=CIRCLE('',#12113,185.);
#2282=CIRCLE('',#12115,210.);
#2283=CIRCLE('',#12116,135.);
#2284=CIRCLE('',#12117,250.);
#2285=CIRCLE('',#12118,185.);
#2286=CIRCLE('',#12120,275.);
#2287=CIRCLE('',#12121,140.432116498651);
#2288=CIRCLE('',#12122,140.432116498845);
#2289=CIRCLE('',#12123,275.);
#2290=CIRCLE('',#12125,250.);
#2291=CIRCLE('',#12126,135.);
#2292=CIRCLE('',#12127,210.);
#2293=CIRCLE('',#12128,185.);
#2294=CIRCLE('',#12130,135.);
#2295=CIRCLE('',#12131,135.);
#2296=CIRCLE('',#12133,137.537590042586);
#2297=CIRCLE('',#12135,137.537590188513);
#2298=CIRCLE('',#12138,110.);
#2299=CIRCLE('',#12139,91.7232983475876);
#2300=CIRCLE('',#12141,113.104956182355);
#2301=CIRCLE('',#12142,113.104956182419);
#2302=CIRCLE('',#12143,110.);
#2303=CIRCLE('',#12144,110.);
#2304=CIRCLE('',#12146,91.7232983475977);
#2305=CIRCLE('',#12147,110.);
#2306=CIRCLE('',#12149,25.);
#2307=CIRCLE('',#12150,25.);
#2308=CIRCLE('',#12151,25.);
#2309=CIRCLE('',#12153,25.);
#2310=CIRCLE('',#12156,25.);
#2311=CIRCLE('',#12157,25.);
#2312=CIRCLE('',#12158,25.);
#2313=CIRCLE('',#12160,25.);
#2314=CIRCLE('',#12163,25.);
#2315=CIRCLE('',#12165,25.);
#2316=CIRCLE('',#12166,25.);
#2317=CIRCLE('',#12169,25.);
#2318=CIRCLE('',#12171,25.);
#2319=CIRCLE('',#12172,25.);
#2320=CIRCLE('',#12174,25.);
#2321=CIRCLE('',#12176,25.);
#2322=CIRCLE('',#12177,25.);
#2323=CIRCLE('',#12179,25.);
#2324=CIRCLE('',#12183,172.5);
#2325=CIRCLE('',#12185,172.5);
#2326=CIRCLE('',#12188,172.5);
#2327=CIRCLE('',#12190,172.5);
#2328=CIRCLE('',#12193,172.5);
#2329=CIRCLE('',#12195,172.5);
#2330=CIRCLE('',#12198,172.5);
#2331=CIRCLE('',#12200,172.5);
#2332=CIRCLE('',#12203,172.5);
#2333=CIRCLE('',#12205,172.5);
#2334=CIRCLE('',#12208,172.5);
#2335=CIRCLE('',#12210,172.5);
#2336=CIRCLE('',#12218,2.5);
#2337=CIRCLE('',#12220,2.5);
#2338=CIRCLE('',#12222,2.49999999999999);
#2339=CIRCLE('',#12224,2.5);
#2340=CIRCLE('',#12225,2.5);
#2341=CIRCLE('',#12226,2.5);
#2342=CIRCLE('',#12228,2.5);
#2343=CIRCLE('',#12229,2.5);
#2344=CIRCLE('',#12230,2.5);
#2345=CIRCLE('',#12232,2.5);
#2346=CIRCLE('',#12233,2.5);
#2347=CIRCLE('',#12235,2.5);
#2348=CIRCLE('',#12238,2.5);
#2349=CIRCLE('',#12240,2.49999999999999);
#2350=CIRCLE('',#12242,2.5);
#2351=CIRCLE('',#12244,2.5);
#2352=CIRCLE('',#12246,2.49999999999999);
#2353=CIRCLE('',#12248,2.5);
#2354=CIRCLE('',#12250,2.5);
#2355=CIRCLE('',#12252,2.5);
#2356=CIRCLE('',#12253,2.5);
#2357=CIRCLE('',#12255,2.5);
#2358=CIRCLE('',#12257,2.5);
#2359=CIRCLE('',#12258,2.5);
#2360=CIRCLE('',#12260,2.5);
#2361=CIRCLE('',#12262,2.5);
#2362=CIRCLE('',#12263,2.5);
#2363=CIRCLE('',#12265,2.5);
#2364=CIRCLE('',#12268,2.5);
#2365=CIRCLE('',#12270,2.5);
#2366=CIRCLE('',#12272,2.5);
#2367=CIRCLE('',#12275,2.5);
#2368=CIRCLE('',#12277,2.5);
#2369=CIRCLE('',#12278,2.5);
#2370=CIRCLE('',#12280,2.5);
#2371=CIRCLE('',#12282,2.5);
#2372=CIRCLE('',#12285,2.5);
#2373=CIRCLE('',#12287,2.49999999999999);
#2374=CIRCLE('',#12289,2.5);
#2375=CIRCLE('',#12291,2.5);
#2376=CIRCLE('',#12293,2.5);
#2377=CIRCLE('',#12295,2.5);
#2378=CIRCLE('',#12296,2.5);
#2379=CIRCLE('',#12298,2.5);
#2380=CIRCLE('',#12301,2.5);
#2381=CIRCLE('',#12304,2.49999999999999);
#2382=CIRCLE('',#12305,2.5);
#2383=CIRCLE('',#12307,2.5);
#2384=CIRCLE('',#12308,2.5);
#2385=CIRCLE('',#12309,2.5);
#2386=CIRCLE('',#12314,2.5);
#2387=CIRCLE('',#12315,2.5);
#2388=CIRCLE('',#12318,2.5);
#2389=CIRCLE('',#12319,2.5);
#2390=CIRCLE('',#12320,2.5);
#2391=CIRCLE('',#12322,2.5);
#2392=CIRCLE('',#12323,2.5);
#2393=CIRCLE('',#12325,2.5);
#2394=CIRCLE('',#12327,2.5);
#2395=CIRCLE('',#12329,2.5);
#2396=CIRCLE('',#12331,2.5);
#2397=CIRCLE('',#12332,2.5);
#2398=CIRCLE('',#12334,2.5);
#2399=CIRCLE('',#12336,2.5);
#2400=CIRCLE('',#12338,2.5);
#2401=CIRCLE('',#12339,2.5);
#2402=CIRCLE('',#12341,2.5);
#2403=CIRCLE('',#12344,2.5);
#2404=CIRCLE('',#12346,2.5);
#2405=CIRCLE('',#12348,2.49999999999999);
#2406=CIRCLE('',#12351,2.5);
#2407=CIRCLE('',#12352,2.5);
#2408=CIRCLE('',#12354,2.49999999999999);
#2409=CIRCLE('',#12356,2.5);
#2410=CIRCLE('',#12357,2.5);
#2411=CIRCLE('',#12358,2.5);
#2412=CIRCLE('',#12360,2.5);
#2413=CIRCLE('',#12362,2.5);
#2414=CIRCLE('',#12365,2.5);
#2415=CIRCLE('',#12367,2.5);
#2416=CIRCLE('',#12368,2.5);
#2417=CIRCLE('',#12370,2.5);
#2418=CIRCLE('',#12371,2.5);
#2419=CIRCLE('',#12373,2.5);
#2420=CIRCLE('',#12375,2.5);
#2421=CIRCLE('',#12377,2.5);
#2422=CIRCLE('',#12380,2.5);
#2423=CIRCLE('',#12381,2.5);
#2424=CIRCLE('',#12383,2.5);
#2425=CIRCLE('',#12385,2.5);
#2426=CIRCLE('',#12387,2.5);
#2427=CIRCLE('',#12389,2.5);
#2428=CIRCLE('',#12391,2.5);
#2429=CIRCLE('',#12392,2.5);
#2430=CIRCLE('',#12393,2.5);
#2431=CIRCLE('',#12395,2.5);
#2432=CIRCLE('',#12397,2.5);
#2433=CIRCLE('',#12398,2.5);
#2434=CIRCLE('',#12400,2.49999999999999);
#2435=CIRCLE('',#12402,2.49999999999999);
#2436=CIRCLE('',#12404,2.5);
#2437=CIRCLE('',#12406,2.5);
#2438=CIRCLE('',#12409,2.49999999999999);
#2439=CIRCLE('',#12412,2.5);
#2440=CIRCLE('',#12413,2.5);
#2441=CIRCLE('',#12414,2.5);
#2442=CIRCLE('',#12416,2.5);
#2443=CIRCLE('',#12419,2.5);
#2444=CIRCLE('',#12421,2.5);
#2445=CIRCLE('',#12422,2.5);
#2688=B_SPLINE_CURVE_WITH_KNOTS('',3,(#16760,#16761,#16762,#16763,#16764,
#16765,#16766,#16767,#16768,#16769,#16770,#16771,#16772,#16773,#16774,#16775,
#16776,#16777,#16778,#16779,#16780,#16781,#16782,#16783,#16784,#16785,#16786,
#16787,#16788,#16789,#16790,#16791,#16792,#16793,#16794,#16795,#16796,#16797,
#16798,#16799,#16800,#16801,#16802,#16803,#16804,#16805),.UNSPECIFIED.,
 .F.,.F.,(4,2,2,2,2,2,2,2,2,2,2,2,2,2,2,2,2,2,2,2,1,1,2,4),(6.93889390390723E-18,
0.012510488710389,0.025020977420778,0.037531466131167,0.0437867104863615,
0.050041954841556,0.0625524435519449,0.0750629322623339,0.0875734209727229,
0.0907010431503202,0.0938286653279175,0.100083909683112,0.12510488710389,
0.137615375814279,0.143870620169474,0.146998242347071,0.150125864524668,
0.175146841945446,0.187657330655835,0.19391257501103,0.197040197188627,
0.198604008277426,0.199385913821825,0.200167819366224),.UNSPECIFIED.);
#2689=B_SPLINE_CURVE_WITH_KNOTS('',3,(#17002,#17003,#17004,#17005,#17006,
#17007,#17008,#17009,#17010,#17011,#17012,#17013,#17014,#17015,#17016,#17017,
#17018,#17019,#17020,#17021,#17022,#17023,#17024,#17025,#17026,#17027,#17028,
#17029,#17030,#17031,#17032,#17033,#17034,#17035,#17036,#17037,#17038,#17039,
#17040,#17041,#17042,#17043,#17044,#17045,#17046,#17047,#17048,#17049,#17050,
#17051,#17052,#17053,#17054,#17055,#17056,#17057,#17058,#17059,#17060,#17061,
#17062,#17063,#17064,#17065,#17066,#17067,#17068,#17069,#17070,#17071,#17072,
#17073,#17074,#17075,#17076,#17077,#17078,#17079,#17080,#17081,#17082,#17083,
#17084,#17085,#17086,#17087,#17088,#17089,#17090,#17091,#17092,#17093,#17094,
#17095,#17096,#17097,#17098,#17099,#17100,#17101,#17102,#17103,#17104,#17105,
#17106,#17107,#17108,#17109,#17110,#17111,#17112,#17113,#17114,#17115,#17116,
#17117,#17118,#17119,#17120,#17121,#17122,#17123,#17124,#17125,#17126,#17127,
#17128,#17129,#17130,#17131,#17132,#17133,#17134,#17135,#17136,#17137,#17138,
#17139,#17140,#17141,#17142,#17143,#17144,#17145,#17146,#17147,#17148,#17149,
#17150,#17151,#17152),.UNSPECIFIED.,.F.,.F.,(4,3,3,3,3,3,3,3,3,3,3,3,3,
3,3,3,3,3,3,3,3,3,3,3,3,3,3,3,3,3,3,3,3,3,3,3,3,3,3,3,3,3,3,3,3,3,3,3,3,
3,4),(0.,0.00264830166754508,0.00338554276768276,0.00615213912871378,0.00675320003132574,
0.00887596942637685,0.0101043537731214,0.0117726415842567,0.0123042782574276,
0.0134347552290183,0.0164143891950787,0.0167346645119878,0.0184564173861414,
0.0200000359794826,0.0215324869504982,0.023233303670992,0.0245199558087172,
0.0246085565148551,0.0248386738910035,0.026435957163951,0.0283935581384038,
0.0296065751333656,0.0307606956435689,0.0327487536070114,0.0351855316944119,
0.0369128347722827,0.0389566060906663,0.0399889043366396,0.0414988150028508,
0.04202602783082,0.0430649739009964,0.0450774572275154,0.0478748168684247,
0.0492171130297102,0.0511362641149651,0.0543446847239159,0.0571422583429271,
0.0606065066150408,0.0615213912871377,0.0631013195616685,0.0645974608514946,
0.0660648494872431,0.0676735304158514,0.0690227825836785,0.0738256695445652,
0.0749288753150223,0.0805294115585075,0.0861299478019928,0.086703763200743,
0.0938021647097608,0.0984342260594203),.UNSPECIFIED.);
#2690=B_SPLINE_CURVE_WITH_KNOTS('',3,(#17154,#17155,#17156,#17157,#17158,
#17159,#17160,#17161,#17162,#17163,#17164,#17165,#17166,#17167,#17168,#17169,
#17170,#17171,#17172,#17173,#17174,#17175,#17176,#17177,#17178,#17179,#17180,
#17181,#17182,#17183,#17184,#17185,#17186,#17187,#17188,#17189,#17190,#17191,
#17192,#17193,#17194,#17195,#17196,#17197,#17198,#17199,#17200,#17201,#17202,
#17203,#17204,#17205,#17206,#17207,#17208,#17209,#17210,#17211,#17212,#17213,
#17214,#17215,#17216,#17217,#17218,#17219,#17220,#17221,#17222,#17223,#17224,
#17225,#17226,#17227,#17228,#17229,#17230,#17231,#17232,#17233,#17234,#17235,
#17236,#17237,#17238,#17239,#17240,#17241,#17242,#17243,#17244,#17245,#17246,
#17247,#17248,#17249,#17250,#17251,#17252,#17253,#17254,#17255,#17256,#17257,
#17258,#17259,#17260,#17261,#17262,#17263,#17264,#17265,#17266,#17267,#17268,
#17269,#17270,#17271,#17272,#17273,#17274,#17275,#17276,#17277,#17278,#17279,
#17280,#17281,#17282,#17283,#17284,#17285,#17286,#17287,#17288,#17289,#17290,
#17291,#17292,#17293,#17294,#17295,#17296,#17297,#17298,#17299,#17300,#17301),
 .UNSPECIFIED.,.F.,.F.,(4,3,3,3,3,3,3,3,3,3,3,3,3,3,3,3,3,3,3,3,3,3,3,3,
3,3,3,3,3,3,3,3,3,3,3,3,3,3,3,3,3,3,3,3,3,3,3,3,3,4),(0.,0.00699935009771002,
0.0115878817442571,0.0121530384978837,0.0176872713323866,0.0232215041668896,
0.0243060769957673,0.0290574768221091,0.0303825962447091,0.0319809849768297,
0.03342085586918,0.0349085984995057,0.0364591154936509,0.0398781022204002,
0.0407914186220395,0.0439575936087226,0.0467217721965195,0.0486121539915344,
0.0513731746692753,0.0527047635302581,0.0546886732404762,0.0557181757572648,
0.0571822792019564,0.0577269328649471,0.058749934730288,0.060765192489418,
0.0631518430351688,0.0648815331197537,0.0668417117383597,0.0679851377317531,
0.0698799713628306,0.0711170083048033,0.0726138269890378,0.0729182309873014,
0.0742789219025961,0.0769869909005962,0.0774720533494774,0.0789947502362431,
0.0806965684066139,0.0820330098607139,0.0839556611802726,0.0850712694851847,
0.0855980872713523,0.0872458532651735,0.0902536243928731,0.0905546388244349,
0.0911477887341263,0.0938804422276097,0.096465786429821,0.097224307983068),
 .UNSPECIFIED.);
#2691=B_SPLINE_CURVE_WITH_KNOTS('',3,(#17305,#17306,#17307,#17308,#17309,
#17310,#17311,#17312,#17313,#17314,#17315,#17316,#17317,#17318,#17319,#17320,
#17321,#17322,#17323,#17324,#17325,#17326,#17327,#17328,#17329,#17330,#17331,
#17332,#17333,#17334,#17335,#17336,#17337,#17338,#17339,#17340,#17341,#17342,
#17343,#17344,#17345,#17346,#17347,#17348,#17349,#17350),.UNSPECIFIED.,
 .F.,.F.,(4,2,1,1,2,2,2,2,2,2,2,2,2,2,2,2,2,2,2,2,2,2,2,4),(-0.000149655236900613,
0.000631565722958083,0.00141278668281678,0.00297522860253417,0.00610011244196896,
0.0123498801208385,0.0248494154785777,0.0498484861940559,0.0529733700334907,
0.0560982538729255,0.0623480215517949,0.074847556909534,0.0998466276250119,
0.106096395303881,0.109221279143316,0.112346162982751,0.12484569834049,
0.137345233698229,0.149844769055968,0.156094536734838,0.162344304413707,
0.174843839771446,0.187343375129185,0.199842910486925),.UNSPECIFIED.);
#2692=B_SPLINE_CURVE_WITH_KNOTS('',3,(#17377,#17378,#17379,#17380,#17381,
#17382,#17383,#17384,#17385,#17386,#17387,#17388,#17389,#17390,#17391,#17392,
#17393,#17394,#17395,#17396,#17397,#17398,#17399,#17400,#17401,#17402,#17403,
#17404,#17405,#17406,#17407,#17408,#17409,#17410,#17411,#17412,#17413,#17414,
#17415,#17416,#17417,#17418,#17419,#17420,#17421,#17422),.UNSPECIFIED.,
 .F.,.F.,(4,2,1,1,2,2,2,2,2,2,2,2,2,2,2,2,2,2,2,2,2,2,2,4),(-0.000143873254053562,
0.00068268999816279,0.00150925325037914,0.00316237975481185,0.00646863276367728,
0.0130811387814081,0.0263061508168699,0.0527561748877933,0.0560624278966588,
0.0593686809055243,0.0659811869232552,0.0792061989587171,0.105656223029641,
0.112268729047372,0.115574982056237,0.118881235065103,0.132106247100564,
0.145331259136026,0.158556271171488,0.165168777189219,0.17178128320695,
0.185006295242412,0.198231307277874,0.211456319313335),.UNSPECIFIED.);
#2693=B_SPLINE_CURVE_WITH_KNOTS('',3,(#17425,#17426,#17427,#17428,#17429,
#17430,#17431,#17432,#17433,#17434,#17435,#17436,#17437,#17438,#17439,#17440,
#17441,#17442,#17443,#17444,#17445,#17446,#17447,#17448,#17449,#17450,#17451,
#17452,#17453,#17454,#17455,#17456,#17457,#17458,#17459,#17460,#17461,#17462,
#17463,#17464,#17465,#17466,#17467,#17468,#17469,#17470,#17471,#17472,#17473,
#17474,#17475,#17476,#17477,#17478,#17479,#17480,#17481,#17482,#17483,#17484,
#17485,#17486,#17487,#17488,#17489,#17490,#17491,#17492,#17493,#17494,#17495,
#17496,#17497,#17498,#17499,#17500,#17501,#17502,#17503,#17504,#17505,#17506,
#17507,#17508,#17509,#17510,#17511,#17512,#17513,#17514,#17515,#17516,#17517,
#17518,#17519,#17520,#17521,#17522,#17523,#17524,#17525,#17526,#17527,#17528,
#17529,#17530,#17531,#17532,#17533,#17534,#17535,#17536,#17537,#17538,#17539,
#17540,#17541,#17542,#17543,#17544,#17545,#17546,#17547,#17548,#17549,#17550,
#17551,#17552,#17553,#17554,#17555,#17556,#17557,#17558,#17559,#17560,#17561,
#17562,#17563,#17564,#17565,#17566,#17567,#17568,#17569,#17570,#17571,#17572),
 .UNSPECIFIED.,.F.,.F.,(4,3,3,3,3,3,3,3,3,3,3,3,3,3,3,3,3,3,3,3,3,3,3,3,
3,3,3,3,3,3,3,3,3,3,3,3,3,3,3,3,3,3,3,3,3,3,3,3,3,4),(0.,0.00881316361102408,
0.012318109623398,0.012654007285576,0.0192322733979474,0.0246628334681499,
0.025308014571152,0.0308463442051709,0.03163501821394,0.0339412090926062,
0.034798520035334,0.0366217278304301,0.0370385678531182,0.037962021856728,
0.0420896412580113,0.0432496109903109,0.0470627457271248,0.0494885274351577,
0.050616029142304,0.0539401501903541,0.0557583986413853,0.056943032785092,
0.0589060145066337,0.060106534606486,0.0619089996968021,0.0620646425562423,
0.06327003642788,0.0660634006959954,0.0684230551784283,0.0695970400706682,
0.0723641943522411,0.0748437627090561,0.0759240437134563,0.0776293975979093,
0.0780803908188895,0.0790875455348503,0.0813357451113595,0.0822510473562443,
0.0846104548920026,0.0868029327330513,0.0879062841801969,0.0885780509990324,
0.0895621613745393,0.0912212332537684,0.0917415528204264,0.0945473329030429,
0.0949050546418204,0.0978841144285108,0.100727891650727,0.101232058284608),
 .UNSPECIFIED.);
#2694=B_SPLINE_CURVE_WITH_KNOTS('',3,(#17574,#17575,#17576,#17577,#17578,
#17579,#17580,#17581,#17582,#17583,#17584,#17585,#17586,#17587,#17588,#17589,
#17590,#17591,#17592,#17593,#17594,#17595,#17596,#17597,#17598,#17599,#17600,
#17601,#17602,#17603,#17604,#17605,#17606,#17607,#17608,#17609,#17610,#17611,
#17612,#17613,#17614,#17615,#17616,#17617,#17618,#17619,#17620,#17621,#17622,
#17623,#17624,#17625,#17626,#17627,#17628,#17629,#17630,#17631,#17632,#17633,
#17634,#17635,#17636,#17637,#17638,#17639,#17640,#17641,#17642,#17643,#17644,
#17645,#17646,#17647,#17648,#17649,#17650,#17651,#17652,#17653,#17654,#17655,
#17656,#17657,#17658,#17659,#17660,#17661,#17662,#17663,#17664,#17665,#17666,
#17667,#17668,#17669,#17670,#17671,#17672,#17673,#17674,#17675,#17676,#17677,
#17678,#17679,#17680,#17681,#17682,#17683,#17684,#17685,#17686,#17687,#17688,
#17689,#17690,#17691,#17692,#17693,#17694,#17695,#17696,#17697,#17698,#17699,
#17700,#17701,#17702,#17703,#17704,#17705,#17706,#17707,#17708,#17709,#17710,
#17711,#17712,#17713,#17714,#17715,#17716,#17717,#17718,#17719,#17720,#17721,
#17722,#17723,#17724,#17725,#17726,#17727,#17728,#17729,#17730,#17731,#17732,
#17733,#17734,#17735,#17736,#17737,#17738,#17739),.UNSPECIFIED.,.F.,.F.,
(4,3,3,3,3,3,3,3,3,3,3,3,3,3,3,3,3,3,3,3,3,3,3,3,3,3,3,3,3,3,3,3,3,3,3,
3,3,3,3,3,3,3,3,3,3,3,3,3,3,3,3,3,3,3,3,4),(2.08166817117217E-17,0.00290669333800962,
0.00338285849467252,0.00638266577622659,0.00675466553082774,0.00957399866433987,
0.0101158798388015,0.0111696651083965,0.0117924346723956,0.0127653315524531,
0.0134658165946075,0.0154513391424759,0.0167960113431925,0.0188942944985078,
0.0191479973286796,0.020104902412734,0.0223393302167929,0.0233947318771642,
0.0248446076333751,0.0250326894729064,0.0255306631049062,0.0266657591960594,
0.0290802964524566,0.0315436764715739,0.0319133288811327,0.0331530367439499,
0.0359945749075088,0.0382959946573593,0.0395777786403494,0.0411983131160884,
0.0414873275454726,0.0427687325086115,0.0446786604335859,0.0459499786559523,
0.0493101507548442,0.0510613262098124,0.0522860562858319,0.056141541692772,
0.0585911480323024,0.0627635580079887,0.0638266577622654,0.0648685301336492,
0.0675785692393606,0.0679976842497239,0.0702093235384919,0.0711211657829561,
0.0757381109941175,0.0765919893147184,0.0773525560315269,0.0826886438907914,
0.0881008269604734,0.0893573208671715,0.0897580784854174,0.095739986643398,
0.0989313195315113,0.102122652419625),.UNSPECIFIED.);
#2695=B_SPLINE_CURVE_WITH_KNOTS('',3,(#17742,#17743,#17744,#17745,#17746,
#17747,#17748,#17749,#17750,#17751,#17752,#17753,#17754,#17755,#17756,#17757,
#17758,#17759,#17760,#17761,#17762,#17763,#17764,#17765,#17766,#17767,#17768,
#17769,#17770,#17771,#17772,#17773,#17774,#17775,#17776,#17777,#17778,#17779,
#17780,#17781,#17782,#17783,#17784,#17785,#17786,#17787),.UNSPECIFIED.,
 .F.,.F.,(4,2,2,2,2,2,2,2,2,2,2,2,2,2,2,2,2,2,2,2,1,1,2,4),(0.,0.0132405753593167,
0.0264811507186334,0.03972172607795,0.0463420137576084,0.0529623014372667,
0.0662028767965833,0.0794434521559,0.0926840275152166,0.0959941713550458,
0.099304315194875,0.105924602874533,0.132405753593167,0.145646328952484,
0.152266616632142,0.155576760471971,0.158886904311801,0.185368055030434,
0.198608630389751,0.205228918069409,0.208539061909239,0.210194133829153,
0.211021669789111,0.211849205749068),.UNSPECIFIED.);
#2696=B_SPLINE_CURVE_WITH_KNOTS('',3,(#17791,#17792,#17793,#17794,#17795,
#17796,#17797,#17798,#17799,#17800,#17801,#17802,#17803,#17804,#17805,#17806,
#17807,#17808,#17809,#17810,#17811,#17812,#17813,#17814,#17815,#17816,#17817,
#17818,#17819,#17820,#17821,#17822,#17823,#17824,#17825,#17826,#17827,#17828,
#17829,#17830,#17831,#17832,#17833,#17834,#17835,#17836,#17837,#17838,#17839,
#17840,#17841,#17842,#17843,#17844,#17845,#17846,#17847,#17848,#17849,#17850,
#17851,#17852,#17853,#17854,#17855,#17856,#17857,#17858,#17859,#17860,#17861,
#17862,#17863,#17864,#17865,#17866,#17867,#17868,#17869,#17870,#17871,#17872,
#17873,#17874,#17875),.UNSPECIFIED.,.F.,.F.,(4,3,3,3,3,3,3,3,3,3,3,3,3,
3,3,3,3,3,3,3,3,3,3,3,3,3,3,3,4),(0.,0.00210238164606691,0.00298624731337001,
0.00299593240969137,0.00448011523757044,0.00449389861453705,0.00556805401174092,
0.00597475171775576,0.00599186481938273,0.00694008292290932,0.0074710492535578,
0.00748983102422842,0.00823006541652398,0.00891808975407265,0.00897029980881955,
0.0089877972290741,0.00949013839786762,0.00972165589821712,0.00973678033149696,
0.0102479898279996,0.0104747574652596,0.0104857634339198,0.0109645659632965,
0.0112298884386646,0.0112347465363427,0.0114330324441498,0.0116282685995547,
0.0118121268564596,0.0119837296387656),.UNSPECIFIED.);
#2697=B_SPLINE_CURVE_WITH_KNOTS('',3,(#17879,#17880,#17881,#17882,#17883,
#17884,#17885,#17886,#17887,#17888,#17889,#17890,#17891,#17892,#17893,#17894,
#17895,#17896,#17897,#17898,#17899,#17900,#17901,#17902,#17903,#17904,#17905,
#17906,#17907,#17908,#17909,#17910,#17911,#17912,#17913,#17914,#17915,#17916,
#17917,#17918,#17919,#17920,#17921,#17922,#17923,#17924,#17925,#17926,#17927,
#17928,#17929,#17930,#17931,#17932,#17933,#17934,#17935,#17936,#17937,#17938,
#17939,#17940,#17941,#17942,#17943,#17944,#17945,#17946,#17947,#17948,#17949,
#17950,#17951,#17952,#17953,#17954,#17955,#17956,#17957),.UNSPECIFIED.,
 .F.,.F.,(4,3,3,3,3,3,3,3,3,3,3,3,3,3,3,3,3,3,3,3,3,3,3,3,3,3,4),(0.,0.000757222794088626,
0.000765731273283226,0.00122273697568558,0.00151444558817725,0.00152974002781745,
0.0019409865546434,0.00227166838226588,0.00229159621626168,0.00278415722201324,
0.00302889117635451,0.00305168138595085,0.00378611397044313,0.00381043827612813,
0.00454333676453176,0.00456831455729546,0.00568821706947207,0.00605778235270903,
0.00608221480188253,0.00735604281924785,0.00757222794088631,0.00759402974301736,
0.00884048373849979,0.00908667352906358,0.0091034204318894,0.0112259507413396,
0.0121155647054181),.UNSPECIFIED.);
#2698=B_SPLINE_CURVE_WITH_KNOTS('',3,(#17960,#17961,#17962,#17963,#17964,
#17965,#17966,#17967,#17968,#17969,#17970,#17971,#17972,#17973,#17974,#17975,
#17976,#17977,#17978,#17979,#17980,#17981,#17982,#17983,#17984,#17985,#17986,
#17987,#17988,#17989,#17990,#17991,#17992,#17993,#17994,#17995,#17996,#17997,
#17998,#17999,#18000,#18001,#18002,#18003,#18004,#18005,#18006,#18007,#18008,
#18009,#18010,#18011,#18012,#18013,#18014,#18015,#18016,#18017,#18018,#18019,
#18020,#18021,#18022,#18023,#18024,#18025,#18026,#18027,#18028,#18029,#18030,
#18031,#18032,#18033,#18034,#18035,#18036,#18037,#18038,#18039,#18040,#18041,
#18042,#18043,#18044),.UNSPECIFIED.,.F.,.F.,(4,3,3,3,3,3,3,3,3,3,3,3,3,
3,3,3,3,3,3,3,3,3,3,3,3,3,3,3,4),(0.,0.00148924028645351,0.00237768466992159,
0.00240031428091277,0.00307153272987116,0.00357468500117901,0.00360047142136915,
0.00432197233413991,0.00477356764211708,0.00480062856182553,0.00528862367612776,
0.00537382713867285,0.00540070713205373,0.00597487440961078,0.00600078570228193,
0.00645684171978798,0.00657682867032061,0.00660086427251013,0.00704835769067905,
0.00717981783844028,0.00720094284273833,0.00766097488130279,0.00778383982492896,
0.00780102141296652,0.00829799353416695,0.00838897096983566,0.00840109998319472,
0.00899484866798043,0.00960125712365108),.UNSPECIFIED.);
#2699=B_SPLINE_CURVE_WITH_KNOTS('',3,(#18048,#18049,#18050,#18051,#18052,
#18053,#18054,#18055,#18056,#18057,#18058,#18059,#18060,#18061,#18062,#18063,
#18064,#18065,#18066,#18067,#18068,#18069,#18070,#18071,#18072,#18073,#18074,
#18075,#18076,#18077,#18078,#18079,#18080,#18081,#18082,#18083,#18084,#18085,
#18086,#18087,#18088,#18089,#18090,#18091,#18092,#18093,#18094,#18095,#18096,
#18097,#18098,#18099,#18100,#18101,#18102,#18103,#18104,#18105,#18106,#18107,
#18108,#18109,#18110,#18111,#18112,#18113,#18114,#18115,#18116,#18117,#18118,
#18119,#18120,#18121,#18122,#18123,#18124,#18125,#18126),.UNSPECIFIED.,
 .F.,.F.,(4,3,3,3,3,3,3,3,3,3,3,3,3,3,3,3,3,3,3,3,3,3,3,3,3,3,4),(0.,0.00162299209129682,
0.00263692856163744,0.00264790906062433,0.00395638686476062,0.0039718635909365,
0.00485040334252278,0.00527680482969886,0.00529581812124867,0.00622095880290044,
0.00659932264757816,0.00661977265156084,0.00736112912107425,0.00792503767209058,
0.00794372718187301,0.00841598728205416,0.00858967996918311,0.00860570444702908,
0.00906736572635407,0.00925571685290464,0.00926768171218515,0.00981205664257965,
0.00992324054391518,0.00992965897734122,0.0102427913968407,0.0105469048764859,
0.0105916362424973),.UNSPECIFIED.);
#2700=B_SPLINE_CURVE_WITH_KNOTS('',3,(#18130,#18131,#18132,#18133,#18134,
#18135,#18136,#18137,#18138,#18139,#18140,#18141,#18142,#18143,#18144,#18145,
#18146,#18147,#18148,#18149,#18150,#18151,#18152,#18153,#18154,#18155,#18156,
#18157,#18158,#18159,#18160,#18161,#18162,#18163,#18164,#18165,#18166,#18167,
#18168,#18169,#18170,#18171,#18172,#18173,#18174,#18175,#18176,#18177,#18178,
#18179,#18180,#18181,#18182,#18183,#18184,#18185,#18186,#18187,#18188,#18189,
#18190,#18191,#18192,#18193,#18194,#18195,#18196,#18197,#18198,#18199,#18200,
#18201,#18202,#18203,#18204,#18205),.UNSPECIFIED.,.F.,.F.,(4,3,3,3,3,3,
3,3,3,3,3,3,3,3,3,3,3,3,3,3,3,3,3,3,3,4),(0.,0.000670198241349187,0.000677695014211876,
0.00121178630208934,0.00134039648269837,0.00135448412697923,0.00180065626354131,
0.00201059472404756,0.00202974735023087,0.00248224413553994,0.00268079296539675,
0.00270360746120654,0.00357365375947468,0.00402118944809509,0.0040477069870127,
0.0048143151556897,0.00536158593079343,0.00538862458081482,0.00657578263990178,
0.00670198241349178,0.00672748973794272,0.00773324143869607,0.00804237889619012,
0.00806372813653269,0.00982128265372075,0.0107231718615868),
 .UNSPECIFIED.);
#2701=B_SPLINE_CURVE_WITH_KNOTS('',3,(#18208,#18209,#18210,#18211,#18212,
#18213,#18214,#18215,#18216,#18217,#18218,#18219,#18220,#18221,#18222,#18223,
#18224,#18225,#18226,#18227,#18228,#18229,#18230,#18231,#18232,#18233,#18234,
#18235,#18236,#18237,#18238,#18239,#18240,#18241,#18242,#18243,#18244,#18245,
#18246,#18247,#18248,#18249,#18250,#18251,#18252,#18253,#18254,#18255,#18256,
#18257,#18258,#18259,#18260,#18261,#18262,#18263,#18264,#18265,#18266,#18267,
#18268,#18269,#18270,#18271,#18272,#18273,#18274,#18275,#18276,#18277,#18278,
#18279,#18280,#18281,#18282,#18283,#18284,#18285,#18286,#18287,#18288,#18289),
 .UNSPECIFIED.,.F.,.F.,(4,3,3,3,3,3,3,3,3,3,3,3,3,3,3,3,3,3,3,3,3,3,3,3,
3,3,3,4),(0.,0.000605114434157146,0.000605179022010971,0.000885247098200934,
0.00117911739500317,0.00121035804402194,0.00121482791364222,0.00181553706603291,
0.00182453317148372,0.00233958065168244,0.00242071608804389,0.00243323369215932,
0.00345385286359851,0.00363107413206585,0.00364741411510169,0.00419813513985867,
0.00423625315407682,0.0042530657539622,0.00484143217608779,0.00485798624729427,
0.00592735701347183,0.00605179022010966,0.00606599525117838,0.00700618113292556,
0.00726214826413153,0.00727234538984921,0.00902506966773751,0.00968286435217533),
 .UNSPECIFIED.);
#2702=B_SPLINE_CURVE_WITH_KNOTS('',3,(#18293,#18294,#18295,#18296,#18297,
#18298,#18299,#18300,#18301,#18302,#18303,#18304,#18305,#18306,#18307,#18308,
#18309,#18310,#18311,#18312,#18313,#18314,#18315,#18316,#18317,#18318,#18319,
#18320,#18321,#18322,#18323,#18324,#18325,#18326,#18327,#18328,#18329,#18330,
#18331,#18332,#18333,#18334,#18335,#18336,#18337,#18338,#18339,#18340,#18341,
#18342,#18343,#18344,#18345,#18346,#18347,#18348,#18349,#18350,#18351,#18352,
#18353,#18354,#18355,#18356,#18357,#18358,#18359,#18360,#18361,#18362,#18363,
#18364,#18365,#18366,#18367,#18368,#18369,#18370,#18371,#18372,#18373,#18374,
#18375,#18376,#18377),.UNSPECIFIED.,.F.,.F.,(4,3,3,3,3,3,3,3,3,3,3,3,3,
3,3,3,3,3,3,3,3,3,3,3,3,3,3,3,4),(0.,0.00210238158617021,0.00298624731337001,
0.00299593240969137,0.00448011523757043,0.00449389861453705,0.00556805401504983,
0.00597475171775576,0.00599186481938273,0.00694008292510282,0.00747104925355784,
0.00748983102422842,0.008230065416524,0.00891808975449004,0.00897029980881959,
0.0089877972290741,0.00949013839878191,0.00972165589821711,0.00973678033149696,
0.0102479898273787,0.0104747574652596,0.0104857634339198,0.0109645659632669,
0.0112298884386646,0.0112347465363427,0.0114330324441506,0.0116282685995556,
0.0118121268564602,0.0119837296387656),.UNSPECIFIED.);
#2703=B_SPLINE_CURVE_WITH_KNOTS('',3,(#18381,#18382,#18383,#18384,#18385,
#18386,#18387,#18388,#18389,#18390,#18391,#18392,#18393,#18394,#18395,#18396,
#18397,#18398,#18399,#18400,#18401,#18402,#18403,#18404,#18405,#18406,#18407,
#18408,#18409,#18410,#18411,#18412,#18413,#18414,#18415,#18416,#18417,#18418,
#18419,#18420,#18421,#18422,#18423,#18424,#18425,#18426,#18427,#18428,#18429,
#18430,#18431,#18432,#18433,#18434,#18435,#18436,#18437,#18438,#18439,#18440,
#18441,#18442,#18443,#18444,#18445,#18446,#18447,#18448,#18449,#18450,#18451,
#18452,#18453,#18454,#18455,#18456,#18457,#18458,#18459),.UNSPECIFIED.,
 .F.,.F.,(4,3,3,3,3,3,3,3,3,3,3,3,3,3,3,3,3,3,3,3,3,3,3,3,3,3,4),(0.,0.000757222794088626,
0.000765731273283215,0.00122273697570158,0.00151444558817725,0.00152974002781745,
0.00194098655463584,0.00227166838226588,0.00229159621626168,0.00278415722201872,
0.00302889117635451,0.00305168138595085,0.00378611397044313,0.00381043827612816,
0.00454333676453176,0.00456831455729547,0.00568821706947819,0.00605778235270903,
0.00608221480188252,0.00735604281927811,0.00757222794088631,0.00759402974301739,
0.00884048373847147,0.00908667352906358,0.00910342043188939,0.0112259507411916,
0.0121155647054181),.UNSPECIFIED.);
#2704=B_SPLINE_CURVE_WITH_KNOTS('',3,(#18464,#18465,#18466,#18467,#18468,
#18469,#18470,#18471,#18472,#18473,#18474,#18475,#18476,#18477,#18478,#18479,
#18480,#18481,#18482,#18483,#18484,#18485,#18486,#18487,#18488,#18489,#18490,
#18491,#18492,#18493,#18494,#18495,#18496,#18497,#18498,#18499,#18500,#18501,
#18502,#18503,#18504,#18505,#18506,#18507,#18508,#18509,#18510,#18511,#18512,
#18513,#18514,#18515,#18516,#18517,#18518,#18519,#18520,#18521,#18522,#18523,
#18524,#18525,#18526,#18527,#18528,#18529,#18530,#18531,#18532,#18533,#18534,
#18535,#18536,#18537,#18538,#18539,#18540,#18541,#18542,#18543,#18544,#18545,
#18546,#18547,#18548),.UNSPECIFIED.,.F.,.F.,(4,3,3,3,3,3,3,3,3,3,3,3,3,
3,3,3,3,3,3,3,3,3,3,3,3,3,3,3,4),(0.,0.00210238158617021,0.00298624731337001,
0.00299593240969137,0.00448011523757043,0.00449389861453705,0.00556805401504983,
0.00597475171775576,0.00599186481938273,0.00694008292510282,0.00747104925355784,
0.00748983102422842,0.008230065416524,0.00891808975449004,0.00897029980881959,
0.0089877972290741,0.00949013839878191,0.00972165589821711,0.00973678033149696,
0.0102479898273787,0.0104747574652596,0.0104857634339198,0.0109645659632669,
0.0112298884386646,0.0112347465363427,0.0114330324441506,0.0116282685995556,
0.0118121268564602,0.0119837296387656),.UNSPECIFIED.);
#2705=B_SPLINE_CURVE_WITH_KNOTS('',3,(#18552,#18553,#18554,#18555,#18556,
#18557,#18558,#18559,#18560,#18561,#18562,#18563,#18564,#18565,#18566,#18567,
#18568,#18569,#18570,#18571,#18572,#18573,#18574,#18575,#18576,#18577,#18578,
#18579,#18580,#18581,#18582,#18583,#18584,#18585,#18586,#18587,#18588,#18589,
#18590,#18591,#18592,#18593,#18594,#18595,#18596,#18597,#18598,#18599,#18600,
#18601,#18602,#18603,#18604,#18605,#18606,#18607,#18608,#18609,#18610,#18611,
#18612,#18613,#18614,#18615,#18616,#18617,#18618,#18619,#18620,#18621,#18622,
#18623,#18624,#18625,#18626,#18627,#18628,#18629,#18630),.UNSPECIFIED.,
 .F.,.F.,(4,3,3,3,3,3,3,3,3,3,3,3,3,3,3,3,3,3,3,3,3,3,3,3,3,3,4),(0.,0.000757222794088626,
0.000765731273283228,0.00122273697432919,0.00151444558817725,0.00152974002781744,
0.00194098655327453,0.00227166838226588,0.00229159621626166,0.00278415722112148,
0.00302889117635451,0.00305168138595084,0.00378611397044313,0.00381043827612816,
0.00454333676453176,0.00456831455729547,0.00568821706029033,0.00605778235270903,
0.00608221480188251,0.00735604281963548,0.00757222794088631,0.00759402974301735,
0.0088404837342444,0.00908667352906358,0.00910342043188939,0.0112259507925462,
0.0121155647054181),.UNSPECIFIED.);
#2706=B_SPLINE_CURVE_WITH_KNOTS('',3,(#18636,#18637,#18638,#18639,#18640,
#18641,#18642,#18643,#18644,#18645,#18646,#18647,#18648,#18649,#18650,#18651,
#18652,#18653,#18654,#18655,#18656,#18657,#18658,#18659,#18660,#18661,#18662,
#18663,#18664,#18665,#18666,#18667,#18668,#18669,#18670,#18671,#18672,#18673,
#18674,#18675,#18676,#18677,#18678,#18679,#18680,#18681,#18682,#18683,#18684,
#18685,#18686,#18687,#18688,#18689,#18690,#18691,#18692,#18693,#18694,#18695,
#18696,#18697,#18698,#18699,#18700,#18701,#18702,#18703,#18704,#18705,#18706,
#18707,#18708,#18709,#18710,#18711,#18712,#18713,#18714,#18715,#18716,#18717,
#18718,#18719,#18720),.UNSPECIFIED.,.F.,.F.,(4,3,3,3,3,3,3,3,3,3,3,3,3,
3,3,3,3,3,3,3,3,3,3,3,3,3,3,3,4),(0.,0.00210238158611208,0.00298624731337002,
0.00299593240969137,0.00448011523757044,0.00449389861453705,0.00556805401505052,
0.00597475171775575,0.00599186481938273,0.00694008292511326,0.00747104925355785,
0.00748983102422842,0.008230065416524,0.00891808975448554,0.00897029980881958,
0.0089877972290741,0.00949013839877169,0.0097216558982171,0.00973678033149696,
0.0102479898273712,0.0104747574652596,0.0104857634339198,0.0109645659632994,
0.0112298884386646,0.0112347465363427,0.0114330324441497,0.0116282685995542,
0.011812126856459,0.0119837296387656),.UNSPECIFIED.);
#2707=B_SPLINE_CURVE_WITH_KNOTS('',3,(#18724,#18725,#18726,#18727,#18728,
#18729,#18730,#18731,#18732,#18733,#18734,#18735,#18736,#18737,#18738,#18739,
#18740,#18741,#18742,#18743,#18744,#18745,#18746,#18747,#18748,#18749,#18750,
#18751,#18752,#18753,#18754,#18755,#18756,#18757,#18758,#18759,#18760,#18761,
#18762,#18763,#18764,#18765,#18766,#18767,#18768,#18769,#18770,#18771,#18772,
#18773,#18774,#18775,#18776,#18777,#18778,#18779,#18780,#18781,#18782,#18783,
#18784,#18785,#18786,#18787,#18788,#18789,#18790,#18791,#18792,#18793,#18794,
#18795,#18796,#18797,#18798,#18799,#18800,#18801,#18802),.UNSPECIFIED.,
 .F.,.F.,(4,3,3,3,3,3,3,3,3,3,3,3,3,3,3,3,3,3,3,3,3,3,3,3,3,3,4),(0.,0.000757222794088626,
0.000765731273283226,0.00122273697568558,0.00151444558817725,0.00152974002781745,
0.0019409865546434,0.00227166838226588,0.00229159621626168,0.00278415722201324,
0.00302889117635451,0.00305168138595085,0.00378611397044313,0.00381043827612813,
0.00454333676453176,0.00456831455729546,0.00568821706947207,0.00605778235270903,
0.00608221480188253,0.00735604281924785,0.00757222794088631,0.00759402974301736,
0.00884048373849979,0.00908667352906358,0.0091034204318894,0.0112259507413396,
0.0121155647054181),.UNSPECIFIED.);
#2708=B_SPLINE_CURVE_WITH_KNOTS('',3,(#18807,#18808,#18809,#18810,#18811,
#18812,#18813,#18814,#18815,#18816,#18817,#18818,#18819,#18820,#18821,#18822,
#18823,#18824,#18825,#18826,#18827,#18828,#18829,#18830,#18831,#18832,#18833,
#18834,#18835,#18836,#18837,#18838,#18839,#18840,#18841,#18842,#18843,#18844,
#18845,#18846,#18847,#18848,#18849,#18850,#18851,#18852,#18853,#18854,#18855,
#18856,#18857,#18858,#18859,#18860,#18861,#18862,#18863,#18864,#18865,#18866,
#18867,#18868,#18869,#18870,#18871,#18872,#18873,#18874,#18875,#18876,#18877,
#18878,#18879,#18880,#18881,#18882,#18883,#18884,#18885,#18886,#18887,#18888,
#18889,#18890,#18891),.UNSPECIFIED.,.F.,.F.,(4,3,3,3,3,3,3,3,3,3,3,3,3,
3,3,3,3,3,3,3,3,3,3,3,3,3,3,3,4),(0.,0.00148924026782088,0.00237768466992155,
0.00240031428091271,0.00307153273081633,0.00357468500117894,0.00360047142136908,
0.00432197233415202,0.00477356764211701,0.00480062856182546,0.0052886236761061,
0.00537382713867274,0.00540070713205367,0.00597487440961069,0.00600078570228188,
0.00645684171980056,0.00657682867032059,0.00660086427251008,0.00704835769063998,
0.00717981783844027,0.00720094284273829,0.00766097488126005,0.00778383982492894,
0.0078010214129665,0.00829799353413678,0.00838897096983562,0.00840109998319471,
0.00899484866798042,0.00960125712365109),.UNSPECIFIED.);
#2709=B_SPLINE_CURVE_WITH_KNOTS('',3,(#18895,#18896,#18897,#18898,#18899,
#18900,#18901,#18902,#18903,#18904,#18905,#18906,#18907,#18908,#18909,#18910,
#18911,#18912,#18913,#18914,#18915,#18916,#18917,#18918,#18919,#18920,#18921,
#18922,#18923,#18924,#18925,#18926,#18927,#18928,#18929,#18930,#18931,#18932,
#18933,#18934,#18935,#18936,#18937,#18938,#18939,#18940,#18941,#18942,#18943,
#18944,#18945,#18946,#18947,#18948,#18949,#18950,#18951,#18952,#18953,#18954,
#18955,#18956,#18957,#18958,#18959,#18960,#18961,#18962,#18963,#18964,#18965,
#18966,#18967,#18968,#18969,#18970,#18971,#18972,#18973),.UNSPECIFIED.,
 .F.,.F.,(4,3,3,3,3,3,3,3,3,3,3,3,3,3,3,3,3,3,3,3,3,3,3,3,3,3,4),(0.,0.00162299209129682,
0.00263692856163744,0.00264790906062433,0.00395638686476062,0.0039718635909365,
0.00485040334252278,0.00527680482969886,0.00529581812124867,0.00622095880290044,
0.00659932264757816,0.00661977265156084,0.00736112912107425,0.00792503767209058,
0.00794372718187301,0.00841598728205416,0.00858967996918311,0.00860570444702908,
0.00906736572635407,0.00925571685290464,0.00926768171218515,0.00981205664257965,
0.00992324054391518,0.00992965897734122,0.0102427913968407,0.0105469048764859,
0.0105916362424973),.UNSPECIFIED.);
#2710=B_SPLINE_CURVE_WITH_KNOTS('',3,(#18977,#18978,#18979,#18980,#18981,
#18982,#18983,#18984,#18985,#18986,#18987,#18988,#18989,#18990,#18991,#18992,
#18993,#18994,#18995,#18996,#18997,#18998,#18999,#19000,#19001,#19002,#19003,
#19004,#19005,#19006,#19007,#19008,#19009,#19010,#19011,#19012,#19013,#19014,
#19015,#19016,#19017,#19018,#19019,#19020,#19021,#19022,#19023,#19024,#19025,
#19026,#19027,#19028,#19029,#19030,#19031,#19032,#19033,#19034,#19035,#19036,
#19037,#19038,#19039,#19040,#19041,#19042,#19043,#19044,#19045,#19046,#19047,
#19048,#19049,#19050,#19051,#19052),.UNSPECIFIED.,.F.,.F.,(4,3,3,3,3,3,
3,3,3,3,3,3,3,3,3,3,3,3,3,3,3,3,3,3,3,4),(0.,0.000670198241349186,0.000677695014211875,
0.00121178630209164,0.00134039648269837,0.00135448412697922,0.00180065626354447,
0.00201059472404756,0.00202974735023086,0.00248224413502192,0.00268079296539674,
0.00270360746120654,0.00357365374674483,0.00402118944809509,0.00404770698701264,
0.00481431515658267,0.00536158593079343,0.00538862458081481,0.00657578262947852,
0.00670198241349177,0.00672748973794275,0.00773324144018303,0.00804237889619011,
0.0080637281365327,0.00982128266121442,0.0107231718615868),
 .UNSPECIFIED.);
#2711=B_SPLINE_CURVE_WITH_KNOTS('',3,(#19056,#19057,#19058,#19059,#19060,
#19061,#19062,#19063,#19064,#19065,#19066,#19067,#19068,#19069,#19070,#19071,
#19072,#19073,#19074,#19075,#19076,#19077,#19078,#19079,#19080,#19081,#19082,
#19083,#19084,#19085,#19086,#19087,#19088,#19089,#19090,#19091,#19092,#19093,
#19094,#19095,#19096,#19097,#19098,#19099,#19100,#19101,#19102,#19103,#19104,
#19105,#19106,#19107,#19108,#19109,#19110,#19111,#19112,#19113,#19114,#19115,
#19116,#19117,#19118,#19119,#19120,#19121,#19122,#19123,#19124,#19125,#19126,
#19127,#19128,#19129,#19130,#19131,#19132,#19133,#19134,#19135,#19136,#19137),
 .UNSPECIFIED.,.F.,.F.,(4,3,3,3,3,3,3,3,3,3,3,3,3,3,3,3,3,3,3,3,3,3,3,3,
3,3,3,4),(0.,0.000605114434157146,0.000605179022010974,0.000885247097935683,
0.00117911739448651,0.00121035804402195,0.00121482791364224,0.00181553706603292,
0.0018245331714837,0.00233958065100891,0.0024207160880439,0.00243323369215935,
0.00345385281984219,0.00363107413206586,0.00364741411510171,0.00419813513510053,
0.00423625315407683,0.00425306575396225,0.0048414321760878,0.00485798624729432,
0.00592735697734792,0.00605179022010969,0.00606599525117843,0.00700618110877007,
0.00726214826413157,0.00727234538984928,0.00902506970597653,0.00968286435217534),
 .UNSPECIFIED.);
#2712=B_SPLINE_CURVE_WITH_KNOTS('',3,(#19315,#19316,#19317,#19318,#19319,
#19320,#19321,#19322,#19323,#19324,#19325,#19326,#19327),.UNSPECIFIED.,
 .F.,.F.,(4,3,3,3,4),(0.,0.00593450809716826,0.00700067642027143,0.0123164151030575,
0.013971448523345),.UNSPECIFIED.);
#2713=B_SPLINE_CURVE_WITH_KNOTS('',3,(#19334,#19335,#19336,#19337,#19338,
#19339,#19340,#19341,#19342,#19343,#19344,#19345,#19346),.UNSPECIFIED.,
 .F.,.F.,(4,3,3,3,4),(0.,0.00603891432879301,0.00699666903166635,0.0124146814900899,
0.0139660167977673),.UNSPECIFIED.);
#2714=B_SPLINE_CURVE_WITH_KNOTS('',3,(#19351,#19352,#19353,#19354,#19355,
#19356,#19357,#19358,#19359,#19360,#19361,#19362,#19363),.UNSPECIFIED.,
 .F.,.F.,(4,3,3,3,4),(0.,0.00541801249293307,0.00696934776611258,0.0130082622991793,
0.0139660167977673),.UNSPECIFIED.);
#2715=B_SPLINE_CURVE_WITH_KNOTS('',3,(#19367,#19368,#19369,#19370,#19371,
#19372,#19373,#19374,#19375,#19376,#19377,#19378,#19379),.UNSPECIFIED.,
 .F.,.F.,(4,3,3,3,4),(0.,0.0053157386001603,0.00697077210307279,0.0129052800531378,
0.013971448523345),.UNSPECIFIED.);
#2716=B_SPLINE_CURVE_WITH_KNOTS('',3,(#19420,#19421,#19422,#19423,#19424,
#19425,#19426,#19427,#19428,#19429,#19430,#19431,#19432,#19433,#19434,#19435,
#19436,#19437,#19438,#19439,#19440,#19441,#19442,#19443,#19444,#19445,#19446,
#19447,#19448,#19449,#19450,#19451,#19452,#19453,#19454,#19455,#19456,#19457,
#19458,#19459,#19460,#19461,#19462,#19463,#19464,#19465,#19466,#19467,#19468,
#19469,#19470,#19471,#19472,#19473,#19474,#19475,#19476,#19477,#19478,#19479,
#19480,#19481,#19482,#19483,#19484,#19485,#19486,#19487,#19488,#19489,#19490,
#19491,#19492,#19493,#19494,#19495,#19496,#19497,#19498,#19499,#19500,#19501,
#19502,#19503,#19504,#19505,#19506,#19507,#19508,#19509,#19510,#19511,#19512,
#19513,#19514,#19515,#19516,#19517,#19518,#19519,#19520,#19521,#19522,#19523,
#19524,#19525,#19526,#19527,#19528,#19529,#19530,#19531,#19532,#19533,#19534,
#19535,#19536,#19537,#19538,#19539,#19540,#19541,#19542,#19543,#19544,#19545,
#19546,#19547,#19548,#19549,#19550,#19551,#19552,#19553,#19554,#19555,#19556,
#19557,#19558,#19559,#19560,#19561,#19562,#19563,#19564,#19565,#19566,#19567,
#19568,#19569,#19570,#19571,#19572,#19573,#19574,#19575,#19576,#19577,#19578,
#19579,#19580,#19581,#19582,#19583,#19584,#19585,#19586,#19587,#19588,#19589,
#19590,#19591,#19592,#19593,#19594,#19595,#19596,#19597,#19598,#19599,#19600,
#19601,#19602,#19603,#19604,#19605,#19606),.UNSPECIFIED.,.F.,.F.,(4,3,3,
3,3,3,3,3,3,3,3,3,3,3,3,3,3,3,3,3,3,3,3,3,3,3,3,3,3,3,3,3,3,3,3,3,3,3,3,
3,3,3,3,3,3,3,3,3,3,3,3,3,3,3,3,3,3,3,3,3,3,3,4),(0.,0.00587025320007918,
0.0116518546601385,0.0124067934665253,0.0183726143829322,0.0233037093202769,
0.0248010444153625,0.0295885380214569,0.0309984330353837,0.0340966058158951,
0.0349555639804154,0.0371915812225473,0.0403989156402141,0.0433496499595692,
0.0463626041882065,0.0466074186405539,0.0494544320203084,0.0524333459706231,
0.0550366402357578,0.0554984816373034,0.0579397193509546,0.0582592733006924,
0.0584943899774514,0.0599505386907733,0.061172236965727,0.0614676725037751,
0.0640852006307616,0.0658681747284104,0.0673052831346648,0.0689343749062278,
0.0699111279608308,0.0713812569705216,0.0728240916258654,0.0729716565715825,
0.0742805734583827,0.0743570049207453,0.0752543696820683,0.0757282061389937,
0.0757370552909,0.0770136999145674,0.0782658534763903,0.078425373133182,
0.0796206612496676,0.0807923001995203,0.0810574254483178,0.0815629826209692,
0.0824911078995598,0.0833977842265763,0.0836193892491146,0.0843234661370702,
0.0844759462860038,0.0848705439497409,0.0859257149372498,0.086104607404437,
0.0871304018360168,0.0873889099510384,0.0884643762089035,0.088522473736195,
0.0895492139112199,0.090301873616073,0.0908732155466535,0.0920722709326854,
0.0932148372811076),.UNSPECIFIED.);
#2717=B_SPLINE_CURVE_WITH_KNOTS('',3,(#19644,#19645,#19646,#19647,#19648,
#19649,#19650,#19651,#19652,#19653,#19654,#19655,#19656,#19657,#19658,#19659,
#19660,#19661,#19662,#19663,#19664,#19665,#19666,#19667,#19668,#19669,#19670,
#19671,#19672,#19673,#19674,#19675,#19676,#19677,#19678,#19679,#19680,#19681,
#19682,#19683,#19684,#19685,#19686,#19687,#19688,#19689,#19690,#19691,#19692,
#19693,#19694,#19695,#19696,#19697,#19698,#19699,#19700,#19701,#19702,#19703,
#19704,#19705,#19706,#19707,#19708,#19709,#19710,#19711,#19712,#19713,#19714,
#19715,#19716,#19717,#19718,#19719,#19720,#19721,#19722,#19723,#19724,#19725,
#19726,#19727,#19728,#19729,#19730,#19731,#19732,#19733,#19734,#19735,#19736,
#19737,#19738,#19739,#19740,#19741,#19742,#19743,#19744,#19745,#19746,#19747,
#19748,#19749,#19750,#19751,#19752,#19753,#19754,#19755,#19756,#19757,#19758,
#19759,#19760,#19761,#19762,#19763,#19764,#19765,#19766,#19767,#19768,#19769,
#19770,#19771,#19772,#19773,#19774,#19775,#19776,#19777,#19778,#19779,#19780,
#19781,#19782,#19783,#19784,#19785,#19786,#19787,#19788,#19789,#19790,#19791,
#19792,#19793,#19794,#19795,#19796,#19797,#19798,#19799,#19800,#19801,#19802,
#19803,#19804,#19805,#19806,#19807,#19808,#19809,#19810,#19811,#19812,#19813,
#19814,#19815,#19816,#19817,#19818,#19819,#19820,#19821,#19822,#19823,#19824,
#19825,#19826,#19827,#19828,#19829,#19830),.UNSPECIFIED.,.F.,.F.,(4,3,3,
3,3,3,3,3,3,3,3,3,3,3,3,3,3,3,3,3,3,3,3,3,3,3,3,3,3,3,3,3,3,3,3,3,3,3,3,
3,3,3,3,3,3,3,3,3,3,3,3,3,3,3,3,3,3,3,3,3,3,3,4),(0.,0.00168391674505757,
0.00237866390505105,0.00293859235176183,0.00392909082463944,0.0047678693047076,
0.00577089595024222,0.00587718470352366,0.00685631905067378,0.00718456765064988,
0.00819626039443761,0.00842377784738116,0.00881577705528549,0.00950100003084725,
0.00968505491475855,0.0106440947494542,0.0116246591280183,0.0117543694070473,
0.0122680279762595,0.0134378823703446,0.0146316209443968,0.0149229678789823,
0.0161755629485317,0.0174530362991548,0.017631554110571,0.0176440794628084,
0.0186861278612264,0.0197665482378735,0.0204254346324111,0.0205701464623328,
0.0220460475716861,0.0235087388140946,0.0251467849670831,0.0261425175891422,
0.0279375140065151,0.0293859235176182,0.0318501667428229,0.0320309300779326,
0.03232451586938,0.0338634522140821,0.0350299832043033,0.0352631082211418,
0.0377194721447005,0.038053160253964,0.0406723517879835,0.0411402929246654,
0.0441530333501108,0.0470174776281889,0.0503147296734146,0.0528946623317125,
0.0558332546834742,0.0565308287838465,0.058771847035236,0.0596542791909667,
0.0627782764692264,0.0673012378967113,0.0690245424335766,0.0705262164422831,
0.0766202357569545,0.0815216901295768,0.0822805858493302,0.0882122169901371,
0.0940349552563772),.UNSPECIFIED.);
#2718=B_SPLINE_CURVE_WITH_KNOTS('',3,(#19849,#19850,#19851,#19852,#19853,
#19854,#19855,#19856,#19857,#19858,#19859,#19860,#19861,#19862,#19863,#19864,
#19865,#19866,#19867,#19868,#19869,#19870,#19871,#19872,#19873,#19874,#19875,
#19876,#19877,#19878,#19879,#19880,#19881,#19882,#19883,#19884,#19885,#19886,
#19887,#19888,#19889,#19890,#19891,#19892,#19893,#19894,#19895,#19896,#19897,
#19898,#19899,#19900,#19901,#19902,#19903,#19904,#19905,#19906,#19907,#19908,
#19909,#19910,#19911,#19912,#19913,#19914,#19915,#19916,#19917,#19918,#19919,
#19920,#19921,#19922,#19923,#19924,#19925,#19926,#19927,#19928,#19929,#19930,
#19931,#19932,#19933,#19934,#19935,#19936,#19937,#19938,#19939,#19940,#19941,
#19942,#19943,#19944,#19945,#19946,#19947,#19948,#19949,#19950,#19951,#19952,
#19953,#19954,#19955,#19956,#19957,#19958,#19959,#19960,#19961,#19962,#19963,
#19964,#19965,#19966,#19967,#19968,#19969,#19970,#19971,#19972,#19973,#19974,
#19975,#19976,#19977,#19978,#19979,#19980,#19981,#19982,#19983,#19984,#19985,
#19986,#19987,#19988,#19989,#19990,#19991,#19992,#19993,#19994,#19995,#19996,
#19997,#19998,#19999,#20000,#20001,#20002,#20003,#20004,#20005,#20006,#20007,
#20008),.UNSPECIFIED.,.F.,.F.,(4,3,3,3,3,3,3,3,3,3,3,3,3,3,3,3,3,3,3,3,
3,3,3,3,3,3,3,3,3,3,3,3,3,3,3,3,3,3,3,3,3,3,3,3,3,3,3,3,3,3,3,3,3,4),(-0.000127168002647682,
0.0032648289235308,0.00665682584970928,0.0119915127057078,0.0134408197020662,
0.0188458139836385,0.0242646482811836,0.0270088074067802,0.032366450211239,
0.0378110333624812,0.0431549242683411,0.0486498535422746,0.054144782816208,
0.0569376853771792,0.0597304018657013,0.060928776668565,0.0662521320816813,
0.0677127705209219,0.0730721047226204,0.0784500787856439,0.0812807582256359,
0.0865149639112802,0.0919904063422261,0.097220456464211,0.10244317541172,
0.107651997921374,0.108416733635064,0.113371574709032,0.115200727487421,
0.118592724413599,0.121984721339778,0.127208398995741,0.132456188050085,
0.135552709044492,0.140533925728601,0.145518391259785,0.150501381841558,
0.155479367307953,0.160446076154363,0.16268868445392,0.166080681380098,
0.169472678306277,0.174505619188982,0.176256672158634,0.181130495805333,
0.186006141113962,0.189824659863348,0.194381555892116,0.198912300408802,
0.203392647568062,0.207549698275247,0.2116829215882,0.215777089793746,0.216960635272776),
 .UNSPECIFIED.);
#2719=B_SPLINE_CURVE_WITH_KNOTS('',3,(#20027,#20028,#20029,#20030,#20031,
#20032,#20033,#20034,#20035,#20036,#20037,#20038,#20039,#20040,#20041,#20042,
#20043,#20044,#20045,#20046,#20047,#20048,#20049,#20050,#20051,#20052,#20053,
#20054,#20055,#20056,#20057,#20058,#20059,#20060,#20061,#20062,#20063,#20064,
#20065,#20066,#20067,#20068,#20069,#20070,#20071,#20072,#20073,#20074,#20075,
#20076,#20077,#20078,#20079,#20080,#20081,#20082,#20083,#20084,#20085,#20086,
#20087,#20088,#20089,#20090,#20091,#20092,#20093,#20094,#20095,#20096,#20097,
#20098,#20099,#20100,#20101,#20102,#20103,#20104,#20105,#20106,#20107,#20108,
#20109,#20110,#20111,#20112,#20113,#20114,#20115,#20116,#20117,#20118,#20119,
#20120,#20121,#20122,#20123,#20124,#20125,#20126,#20127,#20128,#20129,#20130,
#20131,#20132,#20133,#20134,#20135,#20136,#20137,#20138,#20139,#20140,#20141,
#20142,#20143,#20144,#20145,#20146,#20147,#20148,#20149,#20150,#20151,#20152,
#20153,#20154,#20155,#20156,#20157,#20158,#20159,#20160,#20161,#20162,#20163,
#20164,#20165,#20166,#20167,#20168,#20169,#20170,#20171,#20172,#20173,#20174,
#20175,#20176,#20177,#20178,#20179,#20180,#20181,#20182,#20183,#20184,#20185,
#20186,#20187,#20188,#20189,#20190,#20191,#20192,#20193,#20194,#20195),
 .UNSPECIFIED.,.F.,.F.,(4,3,3,3,3,3,3,3,3,3,3,3,3,3,3,3,3,3,3,3,3,3,3,3,
3,3,3,3,3,3,3,3,3,3,3,3,3,3,3,3,3,3,3,3,3,3,3,3,3,3,3,3,3,3,3,3,4),(0.,
0.00406840368139733,0.00816351919635245,0.0122918771767106,0.0134587152954293,
0.0179460716513004,0.0224622816851354,0.0269174305908586,0.0317525397182155,
0.0365884572360659,0.0403761458862878,0.045368531251652,0.0471055035340025,
0.0504701823578598,0.0538348611817171,0.0587609520050433,0.0636963883693916,
0.0686402778496681,0.0735849222481519,0.0785263152925298,0.0807522917725757,
0.08596015285935,0.0911453435853751,0.094211007068005,0.0975756858918623,
0.10094036471572,0.105855287543985,0.107669722363434,0.11283784848067,0.118275174599076,
0.123466116913776,0.128659259968161,0.133850907694542,0.134587152954293,
0.139923299838746,0.145242088010254,0.148045868249722,0.153326319753184,
0.154775225897437,0.157545654220975,0.160316002582348,0.161504583545151,
0.166777046688815,0.172188288550613,0.177494625650974,0.182958319893492,
0.18842201413601,0.193798089195622,0.199161558644946,0.201880729431439,
0.207172416254997,0.208610087079154,0.211974765903011,0.21365710531494,
0.214498275020904,0.215258241940824,0.215339444726868),.UNSPECIFIED.);
#2720=B_SPLINE_CURVE_WITH_KNOTS('',3,(#20797,#20798,#20799,#20800,#20801,
#20802,#20803,#20804,#20805,#20806),.UNSPECIFIED.,.F.,.F.,(4,3,3,4),(0.,
0.00768746870294856,0.0143567530216925,0.0153546747867968),
 .UNSPECIFIED.);
#2721=B_SPLINE_CURVE_WITH_KNOTS('',3,(#20810,#20811,#20812,#20813,#20814,
#20815,#20816,#20817,#20818,#20819),.UNSPECIFIED.,.F.,.F.,(4,3,3,4),(0.,
0.00768475212022721,0.0144698745656401,0.0153509945442703),
 .UNSPECIFIED.);
#2722=B_SPLINE_CURVE_WITH_KNOTS('',3,(#20824,#20825,#20826,#20827,#20828,
#20829,#20830,#20831,#20832,#20833),.UNSPECIFIED.,.F.,.F.,(4,3,3,4),(0.,
0.00678512276816754,0.00766624242405213,0.0153509945442702),
 .UNSPECIFIED.);
#2723=B_SPLINE_CURVE_WITH_KNOTS('',3,(#20840,#20841,#20842,#20843,#20844,
#20845,#20846,#20847,#20848,#20849),.UNSPECIFIED.,.F.,.F.,(4,3,3,4),(0.,
0.00666928397116938,0.00766720608384747,0.0153546747867968),
 .UNSPECIFIED.);
#2724=B_SPLINE_CURVE_WITH_KNOTS('',3,(#20887,#20888,#20889,#20890,#20891,
#20892,#20893,#20894,#20895,#20896,#20897,#20898,#20899,#20900,#20901,#20902,
#20903,#20904,#20905,#20906,#20907,#20908,#20909,#20910,#20911,#20912,#20913,
#20914,#20915,#20916,#20917,#20918,#20919,#20920,#20921,#20922,#20923,#20924,
#20925,#20926,#20927,#20928,#20929,#20930,#20931,#20932,#20933,#20934,#20935,
#20936,#20937,#20938,#20939,#20940,#20941,#20942,#20943,#20944,#20945,#20946,
#20947,#20948,#20949,#20950,#20951,#20952,#20953,#20954,#20955,#20956,#20957,
#20958,#20959,#20960,#20961,#20962,#20963,#20964,#20965,#20966,#20967,#20968,
#20969,#20970,#20971,#20972,#20973,#20974,#20975,#20976,#20977,#20978,#20979,
#20980,#20981,#20982,#20983,#20984,#20985,#20986,#20987,#20988,#20989,#20990,
#20991,#20992,#20993,#20994,#20995,#20996,#20997,#20998,#20999,#21000,#21001,
#21002,#21003,#21004,#21005,#21006,#21007,#21008,#21009,#21010,#21011,#21012,
#21013,#21014,#21015,#21016,#21017,#21018,#21019,#21020,#21021,#21022,#21023,
#21024,#21025,#21026,#21027,#21028,#21029,#21030,#21031,#21032,#21033,#21034,
#21035,#21036,#21037,#21038,#21039,#21040,#21041,#21042,#21043,#21044,#21045,
#21046,#21047,#21048,#21049,#21050,#21051,#21052,#21053,#21054,#21055,#21056,
#21057,#21058,#21059,#21060,#21061,#21062,#21063,#21064,#21065,#21066,#21067,
#21068,#21069,#21070,#21071,#21072,#21073,#21074,#21075,#21076,#21077,#21078,
#21079,#21080,#21081,#21082,#21083,#21084,#21085,#21086,#21087,#21088,#21089,
#21090,#21091,#21092,#21093,#21094,#21095,#21096,#21097,#21098,#21099,#21100),
 .UNSPECIFIED.,.F.,.F.,(4,3,3,3,3,3,3,3,3,3,3,3,3,3,3,3,3,3,3,3,3,3,3,3,
3,3,3,3,3,3,3,3,3,3,3,3,3,3,3,3,3,3,3,3,3,3,3,3,3,3,3,3,3,3,3,3,3,3,3,3,
3,3,3,3,3,3,3,3,3,3,3,4),(0.,0.00536121649079707,0.0107224329815941,0.0119083296245285,
0.0171328352185017,0.0214448659631883,0.023821656300005,0.0294153766011437,
0.0297871200699058,0.0321672989447824,0.0327728648551297,0.0347384176644012,
0.0357560767551434,0.0375285154355795,0.0407799405573036,0.0416735983164754,
0.0428897319263765,0.0456004412105126,0.0475140698351893,0.0500261971384477,
0.0524766748734367,0.0532652736795232,0.0536121649079707,0.0557751307553522,
0.0561021069505934,0.0562927731533692,0.057486465730024,0.0585814667716182,
0.0589040071999902,0.0589733813987678,0.0605030839512922,0.0620069983779697,
0.0634735651758426,0.0643313047141251,0.0643345978895649,0.0656393520467414,
0.0668590262243249,0.0669441062039179,0.0681025607846875,0.0692316257315129,
0.0694789204759748,0.0696958143803621,0.0706207191542974,0.0707145367732808,
0.071381438865015,0.0719262439017434,0.0723764226257606,0.0732437734129232,
0.0740922211334398,0.0742679843726784,0.0750570308711592,0.0757816961429912,
0.0764916855102009,0.0771716653451038,0.0777376391165577,0.0783385807347774,
0.0785857570505588,0.079077943239257,0.0795801179446465,0.0804182473619563,
0.0805402186897528,0.0811493850872042,0.0817226935636484,0.0817585514846556,
0.0821582857848663,0.0823614354785218,0.0827531485315508,0.0830988556073549,
0.0839616629033724,0.0840870494218764,0.0849332566373149,0.0857794638527535),
 .UNSPECIFIED.);
#2725=B_SPLINE_CURVE_WITH_KNOTS('',3,(#21138,#21139,#21140,#21141,#21142,
#21143,#21144,#21145,#21146,#21147,#21148,#21149,#21150,#21151,#21152,#21153,
#21154,#21155,#21156,#21157,#21158,#21159,#21160,#21161,#21162,#21163,#21164,
#21165,#21166,#21167,#21168,#21169,#21170,#21171,#21172,#21173,#21174,#21175,
#21176,#21177,#21178,#21179,#21180,#21181,#21182,#21183,#21184,#21185,#21186,
#21187,#21188,#21189,#21190,#21191,#21192,#21193,#21194,#21195,#21196,#21197,
#21198,#21199,#21200,#21201,#21202,#21203,#21204,#21205,#21206,#21207,#21208,
#21209,#21210,#21211,#21212,#21213,#21214,#21215,#21216,#21217,#21218,#21219,
#21220,#21221,#21222,#21223,#21224,#21225,#21226,#21227,#21228,#21229,#21230,
#21231,#21232,#21233,#21234,#21235,#21236,#21237,#21238,#21239,#21240,#21241,
#21242,#21243,#21244,#21245,#21246,#21247,#21248,#21249,#21250,#21251,#21252,
#21253,#21254,#21255,#21256,#21257,#21258,#21259,#21260,#21261,#21262,#21263,
#21264,#21265,#21266,#21267,#21268,#21269,#21270,#21271,#21272,#21273,#21274,
#21275,#21276,#21277,#21278,#21279,#21280,#21281,#21282,#21283,#21284,#21285,
#21286,#21287,#21288,#21289,#21290,#21291,#21292,#21293,#21294,#21295,#21296,
#21297,#21298,#21299,#21300,#21301,#21302,#21303,#21304,#21305,#21306,#21307,
#21308,#21309,#21310,#21311,#21312,#21313,#21314,#21315,#21316,#21317,#21318,
#21319,#21320,#21321,#21322,#21323,#21324,#21325,#21326,#21327,#21328,#21329,
#21330,#21331,#21332,#21333,#21334,#21335,#21336,#21337,#21338,#21339,#21340,
#21341,#21342,#21343,#21344,#21345,#21346,#21347,#21348,#21349,#21350,#21351,
#21352,#21353,#21354,#21355,#21356,#21357),.UNSPECIFIED.,.F.,.F.,(4,3,3,
3,3,3,3,3,3,3,3,3,3,3,3,3,3,3,3,3,3,3,3,3,3,3,3,3,3,3,3,3,3,3,3,3,3,3,3,
3,3,3,3,3,3,3,3,3,3,3,3,3,3,3,3,3,3,3,3,3,3,3,3,3,3,3,3,3,3,3,3,3,3,4),
(0.,0.000853445909658264,0.00170689181931653,0.00259346888277001,0.00270665419813819,
0.00301811004639099,0.00333278452805475,0.00338331774767277,0.00344497246138023,
0.00398704071753636,0.00405998129720734,0.00463779416072756,0.00522550383422844,
0.00528398471737718,0.00541330839627647,0.00606201299034083,0.00625331267443975,
0.00672179483998648,0.00676663549534561,0.0072193854254239,0.00725603039386378,
0.00783136218365323,0.00811996259441475,0.00880198401199615,0.00936886062699102,
0.010097738709772,0.010826616792553,0.0116132146110347,0.0124664243712336,
0.0133388490992226,0.0135332709906913,0.0139769232258912,0.0147311255351362,
0.0155210222042751,0.0162399251888296,0.0164490515806184,0.0175977301617576,
0.018775784239765,0.0190105677891651,0.0202542001113586,0.021529561127787,
0.0216498696665422,0.0216532335851062,0.0231400660109318,0.0246515136906535,
0.026202452748715,0.0270665419813828,0.0271300556873131,0.0283504938641854,
0.0296458787879955,0.0299579832896972,0.0315284258663565,0.0324798503776594,
0.0328253367756621,0.0352876648060489,0.0378107290799157,0.0386378143164369,
0.0413659622149544,0.0433064671702126,0.0445421276507487,0.0478144982641544,
0.0487197755664892,0.0505253151863032,0.0525549549009522,0.0535380477420698,
0.0541330839627658,0.0565496900761665,0.0625677704660161,0.0649597007553191,
0.0702926004909309,0.074590333644314,0.0757863175478723,0.0811996259441489,
0.0866129343404255),.UNSPECIFIED.);
#2726=B_SPLINE_CURVE_WITH_KNOTS('',3,(#21376,#21377,#21378,#21379,#21380,
#21381,#21382,#21383,#21384,#21385,#21386,#21387,#21388,#21389,#21390,#21391,
#21392,#21393,#21394,#21395,#21396,#21397,#21398,#21399,#21400,#21401,#21402,
#21403,#21404,#21405,#21406,#21407,#21408,#21409,#21410,#21411,#21412,#21413,
#21414,#21415,#21416,#21417,#21418,#21419,#21420,#21421,#21422,#21423,#21424,
#21425,#21426,#21427,#21428,#21429,#21430,#21431,#21432,#21433,#21434,#21435,
#21436,#21437,#21438,#21439,#21440,#21441,#21442,#21443,#21444,#21445,#21446,
#21447,#21448,#21449,#21450,#21451,#21452,#21453,#21454,#21455,#21456,#21457,
#21458,#21459,#21460,#21461,#21462,#21463,#21464,#21465,#21466,#21467,#21468,
#21469,#21470,#21471,#21472,#21473,#21474,#21475,#21476,#21477,#21478,#21479,
#21480,#21481,#21482,#21483,#21484,#21485,#21486,#21487,#21488,#21489,#21490,
#21491,#21492,#21493,#21494,#21495,#21496,#21497,#21498,#21499,#21500,#21501,
#21502,#21503,#21504,#21505,#21506,#21507,#21508,#21509,#21510,#21511,#21512,
#21513,#21514,#21515,#21516,#21517,#21518,#21519,#21520,#21521,#21522,#21523,
#21524,#21525,#21526,#21527,#21528,#21529,#21530,#21531,#21532,#21533,#21534,
#21535),.UNSPECIFIED.,.F.,.F.,(4,3,3,3,3,3,3,3,3,3,3,3,3,3,3,3,3,3,3,3,
3,3,3,3,3,3,3,3,3,3,3,3,3,3,3,3,3,3,3,3,3,3,3,3,3,3,3,3,3,3,3,3,3,4),(-0.000120027570413996,
0.000615336899055743,0.000687456171051644,0.00149493991251728,0.00310990739544856,
0.00633984236131111,0.0117875786308091,0.0127997122930362,0.0183066990136958,
0.0238261998769249,0.0257194521564864,0.0311821835538968,0.0366419530942659,
0.0420953213199303,0.047533539491917,0.0515589318833868,0.0543422828863298,
0.0571261530475139,0.0580188018151119,0.0634547853277745,0.0644786717468369,
0.0699590715687213,0.0754632038688581,0.0773984116102871,0.082796947367055,
0.0882065425473555,0.093617986808073,0.0990281989987573,0.103237891337187,
0.108426657628614,0.109697761268913,0.114131103460074,0.116157631200638,
0.12158252459318,0.127045744727309,0.129077371064088,0.134327451696826,
0.139602688665655,0.144887922475877,0.150186447600716,0.154916850790988,
0.158146785756851,0.161376720722713,0.166713805339851,0.167836590654438,
0.173045937956705,0.178283075697025,0.180756330517889,0.185492323643426,
0.190221955891824,0.194930033223942,0.199617768703279,0.204265609697008,
0.206595810244789),.UNSPECIFIED.);
#2727=B_SPLINE_CURVE_WITH_KNOTS('',3,(#21554,#21555,#21556,#21557,#21558,
#21559,#21560,#21561,#21562,#21563,#21564,#21565,#21566,#21567,#21568,#21569,
#21570,#21571,#21572,#21573,#21574,#21575,#21576,#21577,#21578,#21579,#21580,
#21581,#21582,#21583,#21584,#21585,#21586,#21587,#21588,#21589,#21590,#21591,
#21592,#21593,#21594,#21595,#21596,#21597,#21598,#21599,#21600,#21601,#21602,
#21603,#21604,#21605,#21606,#21607,#21608,#21609,#21610,#21611,#21612,#21613,
#21614,#21615,#21616,#21617,#21618,#21619,#21620,#21621,#21622,#21623,#21624,
#21625,#21626,#21627,#21628,#21629,#21630,#21631,#21632,#21633,#21634,#21635,
#21636,#21637,#21638,#21639,#21640,#21641,#21642,#21643,#21644,#21645,#21646,
#21647,#21648,#21649,#21650,#21651,#21652,#21653,#21654,#21655,#21656,#21657,
#21658,#21659,#21660,#21661,#21662,#21663,#21664,#21665,#21666,#21667,#21668,
#21669,#21670,#21671,#21672,#21673,#21674,#21675,#21676,#21677,#21678,#21679,
#21680,#21681,#21682,#21683,#21684,#21685,#21686,#21687,#21688,#21689,#21690,
#21691,#21692,#21693,#21694,#21695,#21696,#21697,#21698,#21699,#21700,#21701,
#21702,#21703,#21704,#21705,#21706,#21707,#21708,#21709,#21710),
 .UNSPECIFIED.,.F.,.F.,(4,3,3,3,3,3,3,3,3,3,3,3,3,3,3,3,3,3,3,3,3,3,3,3,
3,3,3,3,3,3,3,3,3,3,3,3,3,3,3,3,3,3,3,3,3,3,3,3,3,3,3,3,4),(0.,0.00465397512833474,
0.00934040158699275,0.0140625542141266,0.018797111658081,0.0235416623819038,
0.0258869012718253,0.031135724540156,0.0363582137350459,0.0388303519077379,
0.0441772368004237,0.0453020772256943,0.0485379398846724,0.0517738025436506,
0.0570839432831096,0.0623818493210589,0.0676692441431062,0.0729362028776467,
0.077660703815476,0.0831369521944653,0.088575287007654,0.0906041544513887,
0.0950460719179827,0.0970758797693451,0.102274172320935,0.103547605087301,
0.108966084914322,0.114387970814243,0.119807746002882,0.125219596524798,
0.129434506359127,0.134950329489426,0.140442991021434,0.14237795699504,
0.14782392405742,0.148849682312996,0.151638804562009,0.154427199116194,
0.155321407630952,0.160764764129599,0.166227213607188,0.171695920134864,
0.177169105885651,0.181208308902778,0.186738565261515,0.192256964824344,
0.194151759538691,0.199609501606606,0.200623484856647,0.203859347515625,
0.205477278845114,0.206286244509859,0.207095210174603),.UNSPECIFIED.);
#2728=B_SPLINE_CURVE_WITH_KNOTS('',3,(#22447,#22448,#22449,#22450,#22451,
#22452,#22453,#22454,#22455,#22456,#22457,#22458,#22459,#22460,#22461,#22462,
#22463,#22464,#22465,#22466,#22467,#22468,#22469,#22470,#22471,#22472,#22473,
#22474,#22475,#22476,#22477,#22478,#22479,#22480,#22481,#22482,#22483,#22484,
#22485,#22486,#22487,#22488,#22489,#22490,#22491,#22492,#22493,#22494,#22495,
#22496,#22497,#22498,#22499,#22500,#22501,#22502,#22503,#22504,#22505,#22506,
#22507,#22508,#22509,#22510,#22511,#22512,#22513,#22514,#22515,#22516,#22517,
#22518,#22519,#22520,#22521,#22522,#22523,#22524,#22525,#22526,#22527,#22528,
#22529,#22530,#22531,#22532,#22533,#22534,#22535,#22536,#22537,#22538,#22539,
#22540,#22541,#22542,#22543,#22544,#22545,#22546,#22547,#22548,#22549,#22550,
#22551,#22552),.UNSPECIFIED.,.F.,.F.,(4,3,3,3,3,3,3,3,3,3,3,3,3,3,3,3,3,
3,3,3,3,3,3,3,3,3,3,3,3,3,3,3,3,3,3,4),(0.,0.00197960077599861,0.00247091791055683,
0.00271406396528817,0.00353661742623442,0.00406281433229082,0.00473095927563442,
0.00494183582111366,0.00539811302525832,0.00588176117506153,0.00614016446975763,
0.0064820025407543,0.00670014847819671,0.00703750070456727,0.00735785779192122,
0.00741275373167048,0.00770998130346443,0.00793355713016827,0.00803048320930966,
0.00821222460251388,0.00838031025432408,0.00850817406567731,0.00864821268694884,
0.00877812514044343,0.00890612848419853,0.00902500075932815,0.00903413182795362,
0.00915003699627082,0.00925578338446123,0.00926594216458802,0.00948862534172098,
0.00957480690340761,0.00968337068845401,0.0097292392728174,0.00983010999353415,
0.00988367164222719),.UNSPECIFIED.);
#2729=B_SPLINE_CURVE_WITH_KNOTS('',3,(#22630,#22631,#22632,#22633,#22634,
#22635,#22636,#22637,#22638,#22639,#22640,#22641,#22642,#22643,#22644,#22645,
#22646,#22647,#22648,#22649,#22650,#22651,#22652,#22653,#22654,#22655,#22656,
#22657,#22658,#22659,#22660,#22661,#22662,#22663,#22664,#22665,#22666,#22667,
#22668,#22669,#22670,#22671,#22672,#22673,#22674,#22675,#22676,#22677,#22678,
#22679,#22680,#22681,#22682,#22683,#22684,#22685,#22686,#22687,#22688,#22689,
#22690,#22691,#22692,#22693,#22694,#22695,#22696,#22697,#22698,#22699,#22700,
#22701,#22702,#22703,#22704,#22705,#22706,#22707,#22708,#22709,#22710,#22711,
#22712,#22713,#22714,#22715,#22716,#22717,#22718,#22719,#22720,#22721,#22722,
#22723,#22724,#22725,#22726,#22727,#22728,#22729,#22730,#22731,#22732),
 .UNSPECIFIED.,.F.,.F.,(4,3,3,3,3,3,3,3,3,3,3,3,3,3,3,3,3,3,3,3,3,3,3,3,
3,3,3,3,3,3,3,3,3,3,4),(0.,0.000847545223232314,0.00164832088701133,0.00169509044646463,
0.001942948192431,0.0023393259780218,0.00271143654648364,0.00289047906148623,
0.00324472718726106,0.00339018089292925,0.00373559044008736,0.00380456263483662,
0.00411444755787733,0.00423772611616157,0.00424433990018985,0.00445722296515655,
0.00464735310941275,0.00467010603012326,0.00487822388613578,0.00508527133939388,
0.00526210164977017,0.00543234850501674,0.00546390351830185,0.00560937914391588,
0.00574753034539324,0.00582575793302101,0.0059328165626262,0.00609723736525646,
0.00616149255899438,0.00629753167797226,0.00635658917424234,0.0064781662286767,
0.0066043156769876,0.0067284745812143,0.00678036178585848),
 .UNSPECIFIED.);
#2730=B_SPLINE_CURVE_WITH_KNOTS('',3,(#22746,#22747,#22748,#22749,#22750,
#22751,#22752,#22753,#22754,#22755,#22756,#22757,#22758,#22759,#22760,#22761,
#22762,#22763,#22764,#22765,#22766,#22767,#22768,#22769,#22770,#22771,#22772,
#22773,#22774,#22775,#22776,#22777,#22778,#22779,#22780,#22781,#22782,#22783,
#22784,#22785,#22786,#22787,#22788,#22789,#22790,#22791,#22792,#22793,#22794,
#22795,#22796,#22797,#22798,#22799,#22800,#22801,#22802,#22803,#22804,#22805,
#22806,#22807,#22808,#22809,#22810,#22811,#22812,#22813,#22814,#22815,#22816,
#22817,#22818,#22819,#22820,#22821,#22822,#22823,#22824,#22825,#22826,#22827,
#22828,#22829,#22830,#22831,#22832,#22833,#22834,#22835,#22836,#22837,#22838,
#22839,#22840,#22841,#22842,#22843,#22844,#22845,#22846,#22847,#22848,#22849,
#22850,#22851,#22852,#22853,#22854,#22855,#22856,#22857,#22858,#22859,#22860),
 .UNSPECIFIED.,.F.,.F.,(4,3,3,3,3,3,3,3,3,3,3,3,3,3,3,3,3,3,3,3,3,3,3,3,
3,3,3,3,3,3,3,3,3,3,3,3,3,3,4),(0.,9.18561239655606E-5,0.000187247318122397,
0.000223179866200178,0.000322995769329295,0.000396457195248618,0.000516673504746917,
0.000622443478716646,0.000731484061345082,0.000845574170253623,0.000858929210602675,
0.000978407301811063,0.00110276605193038,0.00123492035522181,0.00124488695743329,
0.00139114459142845,0.00158341591401497,0.00178580066086868,0.00186733043614994,
0.00197093668229903,0.00218794771760141,0.00242197326922363,0.00248977391486658,
0.00258515278144125,0.00295788257484743,0.00321997742071528,0.00365085122472788,
0.00373466087229989,0.00424559974900295,0.00453032492225145,0.0049795478297332,
0.00564687419923879,0.00587646790730166,0.00672137634321008,0.007233651137532,
0.0074693217445998,0.00858965034752487,0.00971088683054975,0.00995909565946641),
 .UNSPECIFIED.);
#2731=B_SPLINE_CURVE_WITH_KNOTS('',3,(#23010,#23011,#23012,#23013,#23014,
#23015,#23016,#23017,#23018,#23019,#23020,#23021,#23022,#23023,#23024,#23025,
#23026,#23027),.UNSPECIFIED.,.F.,.F.,(4,2,2,2,2,2,2,2,4),(0.,0.000517355166269151,
0.0010347103325383,0.00155206549880745,0.0020694206650766,0.00310413099761494,
0.00413884133015328,0.00620826199522997,0.00827768266030667),
 .UNSPECIFIED.);
#2732=B_SPLINE_CURVE_WITH_KNOTS('',3,(#23105,#23106,#23107,#23108,#23109,
#23110,#23111,#23112,#23113,#23114,#23115,#23116,#23117,#23118,#23119,#23120,
#23121,#23122,#23123,#23124,#23125,#23126,#23127,#23128,#23129,#23130,#23131,
#23132,#23133,#23134,#23135,#23136,#23137,#23138,#23139,#23140,#23141,#23142,
#23143,#23144,#23145,#23146,#23147,#23148,#23149,#23150,#23151,#23152,#23153,
#23154,#23155,#23156,#23157,#23158,#23159,#23160,#23161,#23162,#23163,#23164,
#23165,#23166,#23167,#23168,#23169,#23170,#23171,#23172,#23173,#23174,#23175,
#23176,#23177,#23178,#23179,#23180,#23181,#23182,#23183,#23184,#23185,#23186,
#23187,#23188,#23189,#23190,#23191,#23192,#23193,#23194,#23195,#23196,#23197,
#23198,#23199,#23200,#23201,#23202,#23203,#23204,#23205,#23206,#23207,#23208,
#23209,#23210),.UNSPECIFIED.,.F.,.F.,(4,3,3,3,3,3,3,3,3,3,3,3,3,3,3,3,3,
3,3,3,3,3,3,3,3,3,3,3,3,3,3,3,3,3,3,4),(0.,0.00135723929435243,0.00204946145676226,
0.00228622203285677,0.00292292848099983,0.00341673681344062,0.0039067606490192,
0.00409892291352452,0.00448120231546935,0.00453023630184375,0.0049206132320938,
0.00512365364190566,0.00542385726001582,0.00560331504583438,0.00586060524797844,
0.0061050977016897,0.00614838437028681,0.00637684630907044,0.00658758940133999,
0.00660530824785407,0.0066607497344774,0.00681852624425174,0.00696704562612621,
0.00706377833482601,0.00717311509866798,0.00729505291280085,0.00741140394444247,
0.00748396395177441,0.00758472220731649,0.00768548046285857,0.00777764568926981,
0.00785794851170659,0.00794166314495388,0.00803100987111596,0.00811779416605641,
0.00819784582704918),.UNSPECIFIED.);
#2733=B_SPLINE_CURVE_WITH_KNOTS('',3,(#23287,#23288,#23289,#23290,#23291,
#23292,#23293,#23294,#23295,#23296,#23297,#23298,#23299,#23300,#23301,#23302,
#23303,#23304,#23305,#23306,#23307,#23308,#23309,#23310,#23311,#23312,#23313,
#23314,#23315,#23316,#23317,#23318,#23319,#23320,#23321,#23322,#23323,#23324,
#23325,#23326,#23327,#23328,#23329,#23330,#23331,#23332,#23333,#23334,#23335,
#23336,#23337,#23338,#23339,#23340,#23341,#23342,#23343,#23344,#23345,#23346,
#23347,#23348,#23349,#23350,#23351,#23352,#23353,#23354,#23355,#23356,#23357,
#23358,#23359,#23360,#23361,#23362,#23363,#23364,#23365,#23366,#23367,#23368,
#23369,#23370,#23371,#23372,#23373,#23374,#23375,#23376,#23377,#23378,#23379,
#23380,#23381,#23382,#23383),.UNSPECIFIED.,.F.,.F.,(4,3,3,3,3,3,3,3,3,3,
3,3,3,3,3,3,3,3,3,3,3,3,3,3,3,3,3,3,3,3,3,3,4),(0.,0.000170769119259004,
0.000305904332796239,0.000426640701961217,0.000599187316529111,0.00062182697372188,
0.000756823578195052,0.000853281403922433,0.000962782991909417,0.00113222926114292,
0.00127992210588365,0.001328896990288,0.00148406066630655,0.00164727023196531,
0.00170656280784487,0.00171810399452786,0.00194497343526638,0.00212783935765393,
0.00237961725595501,0.00255603792528681,0.00255984421176727,0.0027868478112769,
0.00299980946583919,0.00330293529271853,0.00341312561568967,0.00377553104277187,
0.00392002161607634,0.00428886752640719,0.00468125453704979,0.00487455036175816,
0.00511968842353449,0.0061218062232531,0.00682625123137931),
 .UNSPECIFIED.);
#2734=B_SPLINE_CURVE_WITH_KNOTS('',3,(#23387,#23388,#23389,#23390,#23391,
#23392,#23393,#23394,#23395,#23396,#23397,#23398,#23399,#23400,#23401,#23402,
#23403,#23404,#23405,#23406,#23407,#23408,#23409,#23410,#23411,#23412,#23413,
#23414,#23415,#23416,#23417,#23418,#23419,#23420,#23421,#23422,#23423,#23424,
#23425,#23426,#23427,#23428,#23429,#23430,#23431,#23432,#23433,#23434,#23435,
#23436,#23437,#23438,#23439,#23440,#23441,#23442,#23443,#23444,#23445,#23446,
#23447,#23448,#23449,#23450,#23451,#23452,#23453,#23454,#23455,#23456,#23457,
#23458,#23459,#23460,#23461,#23462,#23463,#23464,#23465,#23466,#23467,#23468,
#23469,#23470,#23471,#23472,#23473,#23474,#23475,#23476,#23477,#23478,#23479,
#23480,#23481,#23482,#23483,#23484,#23485,#23486,#23487,#23488,#23489,#23490,
#23491,#23492),.UNSPECIFIED.,.F.,.F.,(4,3,3,3,3,3,3,3,3,3,3,3,3,3,3,3,3,
3,3,3,3,3,3,3,3,3,3,3,3,3,3,3,3,3,3,4),(0.,0.00197960077597682,0.00247091791055683,
0.00271406396528818,0.00353661742623437,0.00406281433229082,0.00473095927563172,
0.00494183582111366,0.00539811302525833,0.0058817611750583,0.00614016446975659,
0.00648200254113197,0.00670014847819671,0.00703750070456741,0.00735785779192378,
0.00741275373167048,0.00770998130346427,0.00793355713016827,0.00803048320930966,
0.00821222460251474,0.0083803102543245,0.00850817406567731,0.00864821268694884,
0.00877812514044313,0.00890612848419838,0.00902500075932787,0.00903413182795362,
0.00915003699627082,0.00925578338446087,0.00926594216458802,0.00948862534172096,
0.00957480690340761,0.00968337068845101,0.0097292392728174,0.00983010999353228,
0.00988367164222719),.UNSPECIFIED.);
#2735=B_SPLINE_CURVE_WITH_KNOTS('',3,(#23635,#23636,#23637,#23638,#23639,
#23640,#23641,#23642,#23643,#23644,#23645,#23646,#23647,#23648,#23649,#23650,
#23651,#23652,#23653,#23654,#23655,#23656,#23657,#23658,#23659,#23660,#23661,
#23662,#23663,#23664,#23665,#23666,#23667,#23668,#23669,#23670,#23671,#23672,
#23673,#23674,#23675,#23676,#23677,#23678,#23679,#23680,#23681,#23682,#23683,
#23684,#23685,#23686,#23687,#23688,#23689,#23690,#23691,#23692,#23693,#23694,
#23695,#23696,#23697,#23698,#23699,#23700,#23701,#23702,#23703,#23704,#23705,
#23706,#23707,#23708,#23709,#23710,#23711,#23712,#23713,#23714,#23715,#23716,
#23717,#23718,#23719,#23720,#23721,#23722,#23723,#23724,#23725,#23726,#23727,
#23728,#23729,#23730,#23731,#23732,#23733,#23734,#23735,#23736,#23737,#23738,
#23739,#23740,#23741,#23742,#23743,#23744,#23745,#23746,#23747,#23748,#23749),
 .UNSPECIFIED.,.F.,.F.,(4,3,3,3,3,3,3,3,3,3,3,3,3,3,3,3,3,3,3,3,3,3,3,3,
3,3,3,3,3,3,3,3,3,3,3,3,3,3,4),(0.,9.18561239650228E-5,0.000187247318121302,
0.000223179866200187,0.000322995769329302,0.000396457195248715,0.000516673504700863,
0.000622443478716646,0.000731484061341045,0.000845574170246189,0.000858929210603472,
0.000978407301793839,0.00110276605189386,0.00123492035516868,0.00124488695743329,
0.00139114459142878,0.00158341591400849,0.0017858006608566,0.00186733043614994,
0.00197093668229905,0.00218794771763813,0.0024219732692966,0.00248977391486658,
0.0025851527814412,0.00295788257505407,0.00321997742071546,0.00365085122470423,
0.00373466087229989,0.00424559974907391,0.00453032492225087,0.0049795478297332,
0.00564687419895804,0.00587646790729939,0.00672137634272312,0.00723365113753139,
0.0074693217445998,0.00858965034915604,0.00971088683381047,0.00995909565946641),
 .UNSPECIFIED.);
#2736=B_SPLINE_CURVE_WITH_KNOTS('',3,(#23846,#23847,#23848,#23849,#23850,
#23851,#23852,#23853,#23854,#23855,#23856,#23857,#23858,#23859,#23860,#23861,
#23862,#23863,#23864,#23865,#23866,#23867,#23868,#23869,#23870,#23871,#23872,
#23873,#23874,#23875,#23876,#23877,#23878,#23879,#23880,#23881,#23882,#23883,
#23884,#23885,#23886,#23887,#23888,#23889,#23890,#23891,#23892,#23893,#23894,
#23895,#23896,#23897,#23898,#23899,#23900,#23901,#23902,#23903,#23904,#23905,
#23906,#23907,#23908,#23909,#23910,#23911,#23912,#23913,#23914,#23915,#23916,
#23917,#23918,#23919,#23920,#23921,#23922,#23923,#23924,#23925,#23926,#23927,
#23928,#23929,#23930,#23931,#23932,#23933,#23934,#23935,#23936,#23937,#23938,
#23939,#23940,#23941,#23942),.UNSPECIFIED.,.F.,.F.,(4,3,3,3,3,3,3,3,3,3,
3,3,3,3,3,3,3,3,3,3,3,3,3,3,3,3,3,3,3,3,3,3,4),(0.,0.00017076911926328,
0.000305904332796252,0.000426640701961203,0.000599187316529732,0.000621826973721879,
0.000756823578194972,0.000853281403922405,0.000962782991909374,0.00113222926114158,
0.00127992210588361,0.00132889699028796,0.00148406066630834,0.0016472702319681,
0.00170656280784481,0.00171810399452776,0.00194497343526742,0.00212783935765386,
0.00237961725595523,0.00255603792528674,0.00255984421176721,0.00278684781127691,
0.00299980946583915,0.00330293529271767,0.00341312561568961,0.00377553104277046,
0.00392002161607631,0.00428886752635139,0.0046812545369514,0.00487455036175753,
0.00511968842353445,0.00612180622110039,0.00682625123137929),
 .UNSPECIFIED.);
#2737=B_SPLINE_CURVE_WITH_KNOTS('',3,(#23950,#23951,#23952,#23953,#23954,
#23955,#23956,#23957,#23958,#23959,#23960,#23961,#23962,#23963,#23964,#23965,
#23966,#23967,#23968,#23969,#23970,#23971,#23972,#23973,#23974,#23975,#23976,
#23977,#23978,#23979,#23980,#23981,#23982,#23983,#23984,#23985,#23986,#23987,
#23988,#23989,#23990,#23991,#23992,#23993,#23994,#23995,#23996,#23997,#23998,
#23999,#24000,#24001,#24002,#24003,#24004,#24005,#24006,#24007,#24008,#24009,
#24010,#24011,#24012,#24013,#24014,#24015,#24016,#24017,#24018,#24019,#24020,
#24021,#24022,#24023,#24024,#24025,#24026,#24027,#24028,#24029,#24030,#24031,
#24032,#24033,#24034,#24035,#24036,#24037,#24038,#24039,#24040,#24041,#24042,
#24043,#24044,#24045,#24046,#24047,#24048,#24049,#24050,#24051,#24052,#24053,
#24054,#24055),.UNSPECIFIED.,.F.,.F.,(4,3,3,3,3,3,3,3,3,3,3,3,3,3,3,3,3,
3,3,3,3,3,3,3,3,3,3,3,3,3,3,3,3,3,3,4),(0.,0.00135723929435243,0.00204946145676226,
0.00228622203285677,0.00292292848099983,0.00341673681344062,0.0039067606490192,
0.00409892291352452,0.00448120231546935,0.00453023630184375,0.0049206132320938,
0.00512365364190566,0.00542385726001582,0.00560331504583438,0.00586060524797844,
0.0061050977016897,0.00614838437028681,0.00637684630907044,0.00658758940133999,
0.00660530824785407,0.0066607497344774,0.00681852624425174,0.00696704562612621,
0.00706377833482601,0.00717311509866798,0.00729505291280085,0.00741140394444247,
0.00748396395177441,0.00758472220731649,0.00768548046285857,0.00777764568926981,
0.00785794851170659,0.00794166314495388,0.00803100987111596,0.00811779416605641,
0.00819784582704918),.UNSPECIFIED.);
#2738=B_SPLINE_CURVE_WITH_KNOTS('',3,(#24202,#24203,#24204,#24205,#24206,
#24207,#24208,#24209,#24210,#24211,#24212,#24213,#24214,#24215,#24216,#24217,
#24218,#24219),.UNSPECIFIED.,.F.,.F.,(4,2,2,2,2,2,2,2,4),(0.,0.000517355166269167,
0.00103471033253833,0.0015520654988075,0.00206942066507667,0.00310413099761498,
0.0041388413301533,0.00620826199522999,0.00827768266030668),
 .UNSPECIFIED.);
#2739=B_SPLINE_CURVE_WITH_KNOTS('',3,(#24292,#24293,#24294,#24295,#24296,
#24297,#24298,#24299,#24300,#24301,#24302,#24303,#24304,#24305,#24306,#24307,
#24308,#24309,#24310,#24311,#24312,#24313,#24314,#24315,#24316,#24317,#24318,
#24319,#24320,#24321,#24322,#24323,#24324,#24325,#24326,#24327,#24328,#24329,
#24330,#24331,#24332,#24333,#24334,#24335,#24336,#24337,#24338,#24339,#24340,
#24341,#24342,#24343,#24344,#24345,#24346,#24347,#24348,#24349,#24350,#24351,
#24352,#24353,#24354,#24355,#24356,#24357,#24358,#24359,#24360,#24361,#24362,
#24363,#24364,#24365,#24366,#24367,#24368,#24369,#24370,#24371,#24372,#24373,
#24374,#24375,#24376,#24377,#24378,#24379,#24380,#24381,#24382,#24383,#24384,
#24385,#24386,#24387,#24388,#24389,#24390,#24391,#24392,#24393,#24394,#24395,
#24396,#24397,#24398,#24399,#24400,#24401,#24402,#24403,#24404,#24405,#24406),
 .UNSPECIFIED.,.F.,.F.,(4,3,3,3,3,3,3,3,3,3,3,3,3,3,3,3,3,3,3,3,3,3,3,3,
3,3,3,3,3,3,3,3,3,3,3,3,3,3,4),(0.,9.18561239650228E-5,0.000187247318121302,
0.000223179866200187,0.000322995769329302,0.000396457195248715,0.000516673504700863,
0.000622443478716646,0.000731484061341045,0.000845574170246189,0.000858929210603472,
0.000978407301793839,0.00110276605189386,0.00123492035516868,0.00124488695743329,
0.00139114459142878,0.00158341591400849,0.0017858006608566,0.00186733043614994,
0.00197093668229905,0.00218794771763813,0.0024219732692966,0.00248977391486658,
0.0025851527814412,0.00295788257505407,0.00321997742071546,0.00365085122470423,
0.00373466087229989,0.00424559974907391,0.00453032492225087,0.0049795478297332,
0.00564687419895804,0.00587646790729939,0.00672137634272312,0.00723365113753139,
0.0074693217445998,0.00858965034915604,0.00971088683381047,0.00995909565946641),
 .UNSPECIFIED.);
#2740=B_SPLINE_CURVE_WITH_KNOTS('',3,(#24410,#24411,#24412,#24413,#24414,
#24415,#24416,#24417,#24418,#24419,#24420,#24421,#24422,#24423,#24424,#24425,
#24426,#24427,#24428,#24429,#24430,#24431,#24432,#24433,#24434,#24435,#24436,
#24437,#24438,#24439,#24440,#24441,#24442,#24443,#24444,#24445,#24446,#24447,
#24448,#24449,#24450,#24451,#24452,#24453,#24454,#24455,#24456,#24457,#24458,
#24459,#24460,#24461,#24462,#24463,#24464,#24465,#24466,#24467,#24468,#24469,
#24470,#24471,#24472,#24473,#24474,#24475,#24476,#24477,#24478,#24479,#24480,
#24481,#24482,#24483,#24484,#24485,#24486,#24487,#24488,#24489,#24490,#24491,
#24492,#24493,#24494,#24495,#24496,#24497,#24498,#24499,#24500,#24501,#24502,
#24503,#24504,#24505,#24506,#24507,#24508,#24509,#24510,#24511,#24512),
 .UNSPECIFIED.,.F.,.F.,(4,3,3,3,3,3,3,3,3,3,3,3,3,3,3,3,3,3,3,3,3,3,3,3,
3,3,3,3,3,3,3,3,3,3,4),(0.,0.000847545223232322,0.00164832088234661,0.00169509044646464,
0.00194294819243123,0.00233932597799748,0.00271143654641038,0.0028904790614833,
0.00324472718723284,0.00339018089292929,0.00373559044000401,0.0038045626348364,
0.00411444755781185,0.00423772611616159,0.0042443399001899,0.00445722296515594,
0.00464735310929138,0.00467010603012198,0.00487822388608553,0.0050852713393939,
0.0052621016497477,0.00543234850496587,0.00546390351830187,0.00560937914397249,
0.00574753034550799,0.00582575793302147,0.0059328165626262,0.00609723736487279,
0.00616149255899418,0.00629753167790733,0.00635658917424235,0.00647816622867606,
0.00660431567688951,0.0067284745810643,0.0067803617858585),
 .UNSPECIFIED.);
#2741=B_SPLINE_CURVE_WITH_KNOTS('',3,(#24654,#24655,#24656,#24657,#24658,
#24659,#24660,#24661,#24662,#24663,#24664,#24665,#24666,#24667,#24668,#24669,
#24670,#24671,#24672,#24673,#24674,#24675,#24676,#24677,#24678,#24679,#24680,
#24681,#24682,#24683,#24684,#24685,#24686,#24687,#24688,#24689,#24690,#24691,
#24692,#24693,#24694,#24695,#24696,#24697,#24698,#24699,#24700,#24701,#24702,
#24703,#24704,#24705,#24706,#24707,#24708,#24709,#24710,#24711,#24712,#24713,
#24714,#24715,#24716,#24717,#24718,#24719,#24720,#24721,#24722,#24723,#24724,
#24725,#24726,#24727,#24728,#24729,#24730,#24731,#24732,#24733,#24734,#24735,
#24736,#24737,#24738,#24739,#24740,#24741,#24742,#24743,#24744,#24745,#24746,
#24747,#24748,#24749,#24750,#24751,#24752,#24753,#24754,#24755,#24756,#24757,
#24758,#24759),.UNSPECIFIED.,.F.,.F.,(4,3,3,3,3,3,3,3,3,3,3,3,3,3,3,3,3,
3,3,3,3,3,3,3,3,3,3,3,3,3,3,3,3,3,3,4),(0.,0.00197960077764265,0.00247091791055683,
0.00271406396528808,0.00353661742634433,0.00406281433229014,0.00473095927595116,
0.00494183582111366,0.00539811302525782,0.0058817611751927,0.00614016447010104,
0.00648200254249054,0.00670014847819659,0.00703750070457104,0.00735785779193372,
0.00741275373167048,0.0077099813035103,0.00793355713016826,0.00803048320930966,
0.00821222460247987,0.00838031025425421,0.00850817406567739,0.00864821268694884,
0.00877812514043141,0.00890612848419257,0.00902500075930251,0.00903413182795372,
0.00915003699627087,0.00925578338446177,0.00926594216458802,0.00948862534172095,
0.00957480690340761,0.00968337068845094,0.0097292392728174,0.00983010999352899,
0.00988367164222719),.UNSPECIFIED.);
#2742=B_SPLINE_CURVE_WITH_KNOTS('',3,(#24840,#24841,#24842,#24843,#24844,
#24845,#24846,#24847,#24848,#24849,#24850,#24851,#24852,#24853,#24854,#24855,
#24856,#24857,#24858,#24859,#24860,#24861,#24862,#24863,#24864,#24865,#24866,
#24867,#24868,#24869,#24870,#24871,#24872,#24873,#24874,#24875,#24876,#24877,
#24878,#24879,#24880,#24881,#24882,#24883,#24884,#24885,#24886,#24887,#24888,
#24889,#24890,#24891,#24892,#24893,#24894,#24895,#24896,#24897,#24898,#24899,
#24900,#24901,#24902,#24903,#24904,#24905,#24906,#24907,#24908,#24909,#24910,
#24911,#24912,#24913,#24914,#24915,#24916,#24917,#24918,#24919,#24920,#24921,
#24922,#24923,#24924,#24925,#24926,#24927,#24928,#24929,#24930,#24931,#24932,
#24933,#24934,#24935,#24936,#24937,#24938,#24939,#24940,#24941,#24942,#24943,
#24944,#24945),.UNSPECIFIED.,.F.,.F.,(4,3,3,3,3,3,3,3,3,3,3,3,3,3,3,3,3,
3,3,3,3,3,3,3,3,3,3,3,3,3,3,3,3,3,3,4),(0.,0.00197960077599861,0.00247091791055683,
0.00271406396528817,0.00353661742623442,0.00406281433229082,0.00473095927563442,
0.00494183582111366,0.00539811302525832,0.00588176117506153,0.00614016446975763,
0.0064820025407543,0.00670014847819671,0.00703750070456727,0.00735785779192122,
0.00741275373167048,0.00770998130346443,0.00793355713016827,0.00803048320930966,
0.00821222460251388,0.00838031025432408,0.00850817406567731,0.00864821268694884,
0.00877812514044343,0.00890612848419853,0.00902500075932815,0.00903413182795362,
0.00915003699627082,0.00925578338446123,0.00926594216458802,0.00948862534172098,
0.00957480690340761,0.00968337068845401,0.0097292392728174,0.00983010999353415,
0.00988367164222719),.UNSPECIFIED.);
#2743=B_SPLINE_CURVE_WITH_KNOTS('',3,(#25016,#25017,#25018,#25019,#25020,
#25021,#25022,#25023,#25024,#25025,#25026,#25027,#25028,#25029,#25030,#25031,
#25032,#25033,#25034,#25035,#25036,#25037,#25038,#25039,#25040,#25041,#25042,
#25043,#25044,#25045,#25046,#25047,#25048,#25049,#25050,#25051,#25052,#25053,
#25054,#25055,#25056,#25057,#25058,#25059,#25060,#25061,#25062,#25063,#25064,
#25065,#25066,#25067,#25068,#25069,#25070,#25071,#25072,#25073,#25074,#25075,
#25076,#25077,#25078,#25079,#25080,#25081,#25082,#25083,#25084,#25085,#25086,
#25087,#25088,#25089,#25090,#25091,#25092,#25093,#25094,#25095,#25096,#25097,
#25098,#25099,#25100,#25101,#25102,#25103,#25104,#25105,#25106,#25107,#25108,
#25109,#25110,#25111,#25112,#25113,#25114,#25115,#25116,#25117,#25118,#25119,
#25120,#25121,#25122,#25123,#25124,#25125,#25126,#25127,#25128,#25129,#25130),
 .UNSPECIFIED.,.F.,.F.,(4,3,3,3,3,3,3,3,3,3,3,3,3,3,3,3,3,3,3,3,3,3,3,3,
3,3,3,3,3,3,3,3,3,3,3,3,3,3,4),(0.,9.18561239655192E-5,0.000187247318122313,
0.000223179866200178,0.000322995769329295,0.000396457195248687,0.000516673504700411,
0.000622443478716646,0.000731484061341489,0.000845574170246325,0.000858929210603472,
0.000978407301793866,0.0011027660518945,0.0012349203551681,0.00124488695743329,
0.00139114459142878,0.00158341591400812,0.00178580066085747,0.00186733043614994,
0.00197093668229905,0.00218794771764027,0.00242197326929741,0.00248977391486658,
0.0025851527814412,0.00295788257505396,0.00321997742071547,0.00365085122470463,
0.00373466087229989,0.00424559974907373,0.00453032492225088,0.0049795478297332,
0.00564687419896703,0.0058764679072994,0.00672137634272318,0.00723365113753139,
0.0074693217445998,0.00858965034916116,0.00971088683382174,0.00995909565946641),
 .UNSPECIFIED.);
#2744=LINE('',#16758,#3756);
#2745=LINE('',#16820,#3757);
#2746=LINE('',#16823,#3758);
#2747=LINE('',#16831,#3759);
#2748=LINE('',#16834,#3760);
#2749=LINE('',#16840,#3761);
#2750=LINE('',#16843,#3762);
#2751=LINE('',#16892,#3763);
#2752=LINE('',#16897,#3764);
#2753=LINE('',#16902,#3765);
#2754=LINE('',#16907,#3766);
#2755=LINE('',#16912,#3767);
#2756=LINE('',#16917,#3768);
#2757=LINE('',#16922,#3769);
#2758=LINE('',#16927,#3770);
#2759=LINE('',#16932,#3771);
#2760=LINE('',#16937,#3772);
#2761=LINE('',#16942,#3773);
#2762=LINE('',#16947,#3774);
#2763=LINE('',#16949,#3775);
#2764=LINE('',#16954,#3776);
#2765=LINE('',#16962,#3777);
#2766=LINE('',#16965,#3778);
#2767=LINE('',#16970,#3779);
#2768=LINE('',#16976,#3780);
#2769=LINE('',#16982,#3781);
#2770=LINE('',#16988,#3782);
#2771=LINE('',#16995,#3783);
#2772=LINE('',#16998,#3784);
#2773=LINE('',#17352,#3785);
#2774=LINE('',#17354,#3786);
#2775=LINE('',#17362,#3787);
#2776=LINE('',#17367,#3788);
#2777=LINE('',#17370,#3789);
#2778=LINE('',#17372,#3790);
#2779=LINE('',#17374,#3791);
#2780=LINE('',#17877,#3792);
#2781=LINE('',#18128,#3793);
#2782=LINE('',#18379,#3794);
#2783=LINE('',#18550,#3795);
#2784=LINE('',#18632,#3796);
#2785=LINE('',#18722,#3797);
#2786=LINE('',#18805,#3798);
#2787=LINE('',#18975,#3799);
#2788=LINE('',#19138,#3800);
#2789=LINE('',#19142,#3801);
#2790=LINE('',#19144,#3802);
#2791=LINE('',#19146,#3803);
#2792=LINE('',#19148,#3804);
#2793=LINE('',#19150,#3805);
#2794=LINE('',#19151,#3806);
#2795=LINE('',#19155,#3807);
#2796=LINE('',#19157,#3808);
#2797=LINE('',#19159,#3809);
#2798=LINE('',#19161,#3810);
#2799=LINE('',#19162,#3811);
#2800=LINE('',#19164,#3812);
#2801=LINE('',#19168,#3813);
#2802=LINE('',#19171,#3814);
#2803=LINE('',#19172,#3815);
#2804=LINE('',#19174,#3816);
#2805=LINE('',#19178,#3817);
#2806=LINE('',#19181,#3818);
#2807=LINE('',#19183,#3819);
#2808=LINE('',#19184,#3820);
#2809=LINE('',#19187,#3821);
#2810=LINE('',#19189,#3822);
#2811=LINE('',#19191,#3823);
#2812=LINE('',#19193,#3824);
#2813=LINE('',#19195,#3825);
#2814=LINE('',#19196,#3826);
#2815=LINE('',#19198,#3827);
#2816=LINE('',#19202,#3828);
#2817=LINE('',#19205,#3829);
#2818=LINE('',#19207,#3830);
#2819=LINE('',#19211,#3831);
#2820=LINE('',#19219,#3832);
#2821=LINE('',#19229,#3833);
#2822=LINE('',#19237,#3834);
#2823=LINE('',#19251,#3835);
#2824=LINE('',#19255,#3836);
#2825=LINE('',#19259,#3837);
#2826=LINE('',#19263,#3838);
#2827=LINE('',#19267,#3839);
#2828=LINE('',#19271,#3840);
#2829=LINE('',#19275,#3841);
#2830=LINE('',#19279,#3842);
#2831=LINE('',#19283,#3843);
#2832=LINE('',#19288,#3844);
#2833=LINE('',#19290,#3845);
#2834=LINE('',#19294,#3846);
#2835=LINE('',#19298,#3847);
#2836=LINE('',#19299,#3848);
#2837=LINE('',#19303,#3849);
#2838=LINE('',#19306,#3850);
#2839=LINE('',#19307,#3851);
#2840=LINE('',#19310,#3852);
#2841=LINE('',#19312,#3853);
#2842=LINE('',#19313,#3854);
#2843=LINE('',#20730,#3855);
#2844=LINE('',#20739,#3856);
#2845=LINE('',#20749,#3857);
#2846=LINE('',#20758,#3858);
#2847=LINE('',#20767,#3859);
#2848=LINE('',#20769,#3860);
#2849=LINE('',#20773,#3861);
#2850=LINE('',#20775,#3862);
#2851=LINE('',#20777,#3863);
#2852=LINE('',#20782,#3864);
#2853=LINE('',#20783,#3865);
#2854=LINE('',#20785,#3866);
#2855=LINE('',#20789,#3867);
#2856=LINE('',#20791,#3868);
#2857=LINE('',#20792,#3869);
#2858=LINE('',#22254,#3870);
#2859=LINE('',#22256,#3871);
#2860=LINE('',#22258,#3872);
#2861=LINE('',#22259,#3873);
#2862=LINE('',#22263,#3874);
#2863=LINE('',#22265,#3875);
#2864=LINE('',#22267,#3876);
#2865=LINE('',#22269,#3877);
#2866=LINE('',#22271,#3878);
#2867=LINE('',#22272,#3879);
#2868=LINE('',#22276,#3880);
#2869=LINE('',#22278,#3881);
#2870=LINE('',#22280,#3882);
#2871=LINE('',#22285,#3883);
#2872=LINE('',#22289,#3884);
#2873=LINE('',#22290,#3885);
#2874=LINE('',#22294,#3886);
#2875=LINE('',#22296,#3887);
#2876=LINE('',#22298,#3888);
#2877=LINE('',#22299,#3889);
#2878=LINE('',#22303,#3890);
#2879=LINE('',#22306,#3891);
#2880=LINE('',#22310,#3892);
#2881=LINE('',#22313,#3893);
#2882=LINE('',#22317,#3894);
#2883=LINE('',#22319,#3895);
#2884=LINE('',#22321,#3896);
#2885=LINE('',#22322,#3897);
#2886=LINE('',#22326,#3898);
#2887=LINE('',#22329,#3899);
#2888=LINE('',#22333,#3900);
#2889=LINE('',#22336,#3901);
#2890=LINE('',#22340,#3902);
#2891=LINE('',#22342,#3903);
#2892=LINE('',#22344,#3904);
#2893=LINE('',#22345,#3905);
#2894=LINE('',#22349,#3906);
#2895=LINE('',#22351,#3907);
#2896=LINE('',#22354,#3908);
#2897=LINE('',#22358,#3909);
#2898=LINE('',#22362,#3910);
#2899=LINE('',#22363,#3911);
#2900=LINE('',#22367,#3912);
#2901=LINE('',#22369,#3913);
#2902=LINE('',#22371,#3914);
#2903=LINE('',#22372,#3915);
#2904=LINE('',#22376,#3916);
#2905=LINE('',#22378,#3917);
#2906=LINE('',#22381,#3918);
#2907=LINE('',#22384,#3919);
#2908=LINE('',#22388,#3920);
#2909=LINE('',#22390,#3921);
#2910=LINE('',#22392,#3922);
#2911=LINE('',#22393,#3923);
#2912=LINE('',#22396,#3924);
#2913=LINE('',#22399,#3925);
#2914=LINE('',#22403,#3926);
#2915=LINE('',#22405,#3927);
#2916=LINE('',#22409,#3928);
#2917=LINE('',#22411,#3929);
#2918=LINE('',#22413,#3930);
#2919=LINE('',#22414,#3931);
#2920=LINE('',#22418,#3932);
#2921=LINE('',#22420,#3933);
#2922=LINE('',#22422,#3934);
#2923=LINE('',#22423,#3935);
#2924=LINE('',#22427,#3936);
#2925=LINE('',#22429,#3937);
#2926=LINE('',#22431,#3938);
#2927=LINE('',#22432,#3939);
#2928=LINE('',#22436,#3940);
#2929=LINE('',#22438,#3941);
#2930=LINE('',#22440,#3942);
#2931=LINE('',#22441,#3943);
#3756=VECTOR('',#13183,160.);
#3757=VECTOR('',#13200,1000.);
#3758=VECTOR('',#13203,1000.);
#3759=VECTOR('',#13210,1000.);
#3760=VECTOR('',#13213,1000.);
#3761=VECTOR('',#13218,1000.);
#3762=VECTOR('',#13221,1000.);
#3763=VECTOR('',#13278,5.025);
#3764=VECTOR('',#13285,4.49999999999998);
#3765=VECTOR('',#13290,5.025);
#3766=VECTOR('',#13297,4.49999999999998);
#3767=VECTOR('',#13302,5.025);
#3768=VECTOR('',#13309,4.49999999999998);
#3769=VECTOR('',#13314,5.025);
#3770=VECTOR('',#13321,4.49999999999998);
#3771=VECTOR('',#13326,5.025);
#3772=VECTOR('',#13333,4.49999999999998);
#3773=VECTOR('',#13338,5.025);
#3774=VECTOR('',#13345,4.49999999999998);
#3775=VECTOR('',#13348,195.);
#3776=VECTOR('',#13353,35.5);
#3777=VECTOR('',#13362,35.5);
#3778=VECTOR('',#13367,35.5);
#3779=VECTOR('',#13372,4.5);
#3780=VECTOR('',#13379,4.5);
#3781=VECTOR('',#13386,4.5);
#3782=VECTOR('',#13393,4.5);
#3783=VECTOR('',#13400,1000.);
#3784=VECTOR('',#13403,1000.);
#3785=VECTOR('',#13410,160.);
#3786=VECTOR('',#13413,1000.);
#3787=VECTOR('',#13420,1000.);
#3788=VECTOR('',#13425,1000.);
#3789=VECTOR('',#13428,170.);
#3790=VECTOR('',#13429,1000.);
#3791=VECTOR('',#13430,170.);
#3792=VECTOR('',#13439,1000.);
#3793=VECTOR('',#13444,1000.);
#3794=VECTOR('',#13449,1000.);
#3795=VECTOR('',#13454,1000.);
#3796=VECTOR('',#13457,1000.);
#3797=VECTOR('',#13460,1000.);
#3798=VECTOR('',#13463,1000.);
#3799=VECTOR('',#13466,1000.);
#3800=VECTOR('',#13469,1000.);
#3801=VECTOR('',#13472,1000.);
#3802=VECTOR('',#13473,1000.);
#3803=VECTOR('',#13474,1000.);
#3804=VECTOR('',#13475,1000.);
#3805=VECTOR('',#13476,1000.);
#3806=VECTOR('',#13477,1000.);
#3807=VECTOR('',#13480,1000.);
#3808=VECTOR('',#13481,1000.);
#3809=VECTOR('',#13482,1000.);
#3810=VECTOR('',#13483,1000.);
#3811=VECTOR('',#13484,1000.);
#3812=VECTOR('',#13485,1000.);
#3813=VECTOR('',#13488,1000.);
#3814=VECTOR('',#13491,1000.);
#3815=VECTOR('',#13492,1000.);
#3816=VECTOR('',#13493,1000.);
#3817=VECTOR('',#13496,1000.);
#3818=VECTOR('',#13499,1000.);
#3819=VECTOR('',#13500,1000.);
#3820=VECTOR('',#13501,1000.);
#3821=VECTOR('',#13504,1000.);
#3822=VECTOR('',#13505,1000.);
#3823=VECTOR('',#13506,1000.);
#3824=VECTOR('',#13507,1000.);
#3825=VECTOR('',#13508,1000.);
#3826=VECTOR('',#13509,1000.);
#3827=VECTOR('',#13510,1000.);
#3828=VECTOR('',#13513,1000.);
#3829=VECTOR('',#13516,1000.);
#3830=VECTOR('',#13517,1000.);
#3831=VECTOR('',#13520,1000.);
#3832=VECTOR('',#13531,1000.);
#3833=VECTOR('',#13540,1000.);
#3834=VECTOR('',#13549,1000.);
#3835=VECTOR('',#13564,1000.);
#3836=VECTOR('',#13567,1000.);
#3837=VECTOR('',#13570,1000.);
#3838=VECTOR('',#13573,1000.);
#3839=VECTOR('',#13576,1000.);
#3840=VECTOR('',#13579,1000.);
#3841=VECTOR('',#13582,1000.);
#3842=VECTOR('',#13585,1000.);
#3843=VECTOR('',#13588,1000.);
#3844=VECTOR('',#13595,1000.);
#3845=VECTOR('',#13596,1000.);
#3846=VECTOR('',#13601,1000.);
#3847=VECTOR('',#13604,1000.);
#3848=VECTOR('',#13605,1000.);
#3849=VECTOR('',#13608,1000.);
#3850=VECTOR('',#13611,1000.);
#3851=VECTOR('',#13612,1000.);
#3852=VECTOR('',#13615,1000.);
#3853=VECTOR('',#13616,1000.);
#3854=VECTOR('',#13617,1000.);
#3855=VECTOR('',#13712,1000.);
#3856=VECTOR('',#13721,1000.);
#3857=VECTOR('',#13732,1000.);
#3858=VECTOR('',#13741,1000.);
#3859=VECTOR('',#13752,1000.);
#3860=VECTOR('',#13753,1000.);
#3861=VECTOR('',#13758,1000.);
#3862=VECTOR('',#13759,1000.);
#3863=VECTOR('',#13760,1000.);
#3864=VECTOR('',#13765,1000.);
#3865=VECTOR('',#13766,1000.);
#3866=VECTOR('',#13767,1000.);
#3867=VECTOR('',#13772,1000.);
#3868=VECTOR('',#13773,1000.);
#3869=VECTOR('',#13774,1000.);
#3870=VECTOR('',#13863,1000.);
#3871=VECTOR('',#13864,1000.);
#3872=VECTOR('',#13865,1000.);
#3873=VECTOR('',#13866,1000.);
#3874=VECTOR('',#13869,1000.);
#3875=VECTOR('',#13870,1000.);
#3876=VECTOR('',#13871,1000.);
#3877=VECTOR('',#13872,1000.);
#3878=VECTOR('',#13873,1000.);
#3879=VECTOR('',#13874,1000.);
#3880=VECTOR('',#13877,1000.);
#3881=VECTOR('',#13878,1000.);
#3882=VECTOR('',#13879,1000.);
#3883=VECTOR('',#13884,1000.);
#3884=VECTOR('',#13887,1000.);
#3885=VECTOR('',#13888,1000.);
#3886=VECTOR('',#13891,1000.);
#3887=VECTOR('',#13892,1000.);
#3888=VECTOR('',#13893,1000.);
#3889=VECTOR('',#13894,1000.);
#3890=VECTOR('',#13897,1000.);
#3891=VECTOR('',#13900,1000.);
#3892=VECTOR('',#13903,1000.);
#3893=VECTOR('',#13906,1000.);
#3894=VECTOR('',#13909,1000.);
#3895=VECTOR('',#13910,1000.);
#3896=VECTOR('',#13911,1000.);
#3897=VECTOR('',#13912,1000.);
#3898=VECTOR('',#13915,1000.);
#3899=VECTOR('',#13918,1000.);
#3900=VECTOR('',#13921,1000.);
#3901=VECTOR('',#13924,1000.);
#3902=VECTOR('',#13927,1000.);
#3903=VECTOR('',#13928,1000.);
#3904=VECTOR('',#13929,1000.);
#3905=VECTOR('',#13930,1000.);
#3906=VECTOR('',#13933,1000.);
#3907=VECTOR('',#13934,1000.);
#3908=VECTOR('',#13937,1000.);
#3909=VECTOR('',#13940,1000.);
#3910=VECTOR('',#13943,1000.);
#3911=VECTOR('',#13944,1000.);
#3912=VECTOR('',#13947,1000.);
#3913=VECTOR('',#13948,1000.);
#3914=VECTOR('',#13949,1000.);
#3915=VECTOR('',#13950,1000.);
#3916=VECTOR('',#13953,1000.);
#3917=VECTOR('',#13956,1000.);
#3918=VECTOR('',#13959,1000.);
#3919=VECTOR('',#13962,1000.);
#3920=VECTOR('',#13965,1000.);
#3921=VECTOR('',#13966,1000.);
#3922=VECTOR('',#13967,1000.);
#3923=VECTOR('',#13968,1000.);
#3924=VECTOR('',#13971,1000.);
#3925=VECTOR('',#13974,1000.);
#3926=VECTOR('',#13977,1000.);
#3927=VECTOR('',#13980,1000.);
#3928=VECTOR('',#13983,1000.);
#3929=VECTOR('',#13984,1000.);
#3930=VECTOR('',#13985,1000.);
#3931=VECTOR('',#13986,1000.);
#3932=VECTOR('',#13989,1000.);
#3933=VECTOR('',#13990,1000.);
#3934=VECTOR('',#13991,1000.);
#3935=VECTOR('',#13992,1000.);
#3936=VECTOR('',#13995,1000.);
#3937=VECTOR('',#13996,1000.);
#3938=VECTOR('',#13997,1000.);
#3939=VECTOR('',#13998,1000.);
#3940=VECTOR('',#14001,1000.);
#3941=VECTOR('',#14002,1000.);
#3942=VECTOR('',#14003,1000.);
#3943=VECTOR('',#14004,1000.);
#4768=VERTEX_POINT('',#16756);
#4769=VERTEX_POINT('',#16757);
#4770=VERTEX_POINT('',#16759);
#4771=VERTEX_POINT('',#16808);
#4772=VERTEX_POINT('',#16809);
#4773=VERTEX_POINT('',#16812);
#4774=VERTEX_POINT('',#16816);
#4775=VERTEX_POINT('',#16817);
#4776=VERTEX_POINT('',#16819);
#4777=VERTEX_POINT('',#16821);
#4778=VERTEX_POINT('',#16825);
#4779=VERTEX_POINT('',#16826);
#4780=VERTEX_POINT('',#16828);
#4781=VERTEX_POINT('',#16830);
#4782=VERTEX_POINT('',#16832);
#4783=VERTEX_POINT('',#16836);
#4784=VERTEX_POINT('',#16837);
#4785=VERTEX_POINT('',#16839);
#4786=VERTEX_POINT('',#16841);
#4787=VERTEX_POINT('',#16845);
#4788=VERTEX_POINT('',#16846);
#4789=VERTEX_POINT('',#16848);
#4790=VERTEX_POINT('',#16852);
#4791=VERTEX_POINT('',#16853);
#4792=VERTEX_POINT('',#16855);
#4793=VERTEX_POINT('',#16859);
#4794=VERTEX_POINT('',#16860);
#4795=VERTEX_POINT('',#16862);
#4796=VERTEX_POINT('',#16866);
#4797=VERTEX_POINT('',#16867);
#4798=VERTEX_POINT('',#16869);
#4799=VERTEX_POINT('',#16873);
#4800=VERTEX_POINT('',#16875);
#4801=VERTEX_POINT('',#16877);
#4802=VERTEX_POINT('',#16881);
#4803=VERTEX_POINT('',#16882);
#4804=VERTEX_POINT('',#16885);
#4805=VERTEX_POINT('',#16889);
#4806=VERTEX_POINT('',#16891);
#4807=VERTEX_POINT('',#16895);
#4808=VERTEX_POINT('',#16899);
#4809=VERTEX_POINT('',#16901);
#4810=VERTEX_POINT('',#16905);
#4811=VERTEX_POINT('',#16909);
#4812=VERTEX_POINT('',#16911);
#4813=VERTEX_POINT('',#16915);
#4814=VERTEX_POINT('',#16919);
#4815=VERTEX_POINT('',#16921);
#4816=VERTEX_POINT('',#16925);
#4817=VERTEX_POINT('',#16929);
#4818=VERTEX_POINT('',#16931);
#4819=VERTEX_POINT('',#16935);
#4820=VERTEX_POINT('',#16939);
#4821=VERTEX_POINT('',#16941);
#4822=VERTEX_POINT('',#16945);
#4823=VERTEX_POINT('',#16951);
#4824=VERTEX_POINT('',#16953);
#4825=VERTEX_POINT('',#16957);
#4826=VERTEX_POINT('',#16958);
#4827=VERTEX_POINT('',#16961);
#4828=VERTEX_POINT('',#16967);
#4829=VERTEX_POINT('',#16969);
#4830=VERTEX_POINT('',#16973);
#4831=VERTEX_POINT('',#16975);
#4832=VERTEX_POINT('',#16979);
#4833=VERTEX_POINT('',#16981);
#4834=VERTEX_POINT('',#16985);
#4835=VERTEX_POINT('',#16987);
#4836=VERTEX_POINT('',#16991);
#4837=VERTEX_POINT('',#16992);
#4838=VERTEX_POINT('',#16994);
#4839=VERTEX_POINT('',#16996);
#4840=VERTEX_POINT('',#17000);
#4841=VERTEX_POINT('',#17153);
#4842=VERTEX_POINT('',#17302);
#4843=VERTEX_POINT('',#17304);
#4844=VERTEX_POINT('',#17351);
#4845=VERTEX_POINT('',#17356);
#4846=VERTEX_POINT('',#17357);
#4847=VERTEX_POINT('',#17359);
#4848=VERTEX_POINT('',#17361);
#4849=VERTEX_POINT('',#17363);
#4850=VERTEX_POINT('',#17365);
#4851=VERTEX_POINT('',#17369);
#4852=VERTEX_POINT('',#17371);
#4853=VERTEX_POINT('',#17373);
#4854=VERTEX_POINT('',#17376);
#4855=VERTEX_POINT('',#17423);
#4856=VERTEX_POINT('',#17573);
#4857=VERTEX_POINT('',#17740);
#4858=VERTEX_POINT('',#17788);
#4859=VERTEX_POINT('',#17790);
#4860=VERTEX_POINT('',#17876);
#4861=VERTEX_POINT('',#17878);
#4862=VERTEX_POINT('',#17959);
#4863=VERTEX_POINT('',#18045);
#4864=VERTEX_POINT('',#18047);
#4865=VERTEX_POINT('',#18127);
#4866=VERTEX_POINT('',#18129);
#4867=VERTEX_POINT('',#18206);
#4868=VERTEX_POINT('',#18290);
#4869=VERTEX_POINT('',#18292);
#4870=VERTEX_POINT('',#18378);
#4871=VERTEX_POINT('',#18380);
#4872=VERTEX_POINT('',#18461);
#4873=VERTEX_POINT('',#18463);
#4874=VERTEX_POINT('',#18549);
#4875=VERTEX_POINT('',#18551);
#4876=VERTEX_POINT('',#18633);
#4877=VERTEX_POINT('',#18635);
#4878=VERTEX_POINT('',#18721);
#4879=VERTEX_POINT('',#18723);
#4880=VERTEX_POINT('',#18804);
#4881=VERTEX_POINT('',#18806);
#4882=VERTEX_POINT('',#18892);
#4883=VERTEX_POINT('',#18894);
#4884=VERTEX_POINT('',#18974);
#4885=VERTEX_POINT('',#18976);
#4886=VERTEX_POINT('',#19053);
#4887=VERTEX_POINT('',#19055);
#4888=VERTEX_POINT('',#19140);
#4889=VERTEX_POINT('',#19141);
#4890=VERTEX_POINT('',#19143);
#4891=VERTEX_POINT('',#19145);
#4892=VERTEX_POINT('',#19147);
#4893=VERTEX_POINT('',#19149);
#4894=VERTEX_POINT('',#19153);
#4895=VERTEX_POINT('',#19154);
#4896=VERTEX_POINT('',#19156);
#4897=VERTEX_POINT('',#19158);
#4898=VERTEX_POINT('',#19160);
#4899=VERTEX_POINT('',#19163);
#4900=VERTEX_POINT('',#19165);
#4901=VERTEX_POINT('',#19167);
#4902=VERTEX_POINT('',#19169);
#4903=VERTEX_POINT('',#19173);
#4904=VERTEX_POINT('',#19175);
#4905=VERTEX_POINT('',#19177);
#4906=VERTEX_POINT('',#19179);
#4907=VERTEX_POINT('',#19182);
#4908=VERTEX_POINT('',#19186);
#4909=VERTEX_POINT('',#19188);
#4910=VERTEX_POINT('',#19190);
#4911=VERTEX_POINT('',#19192);
#4912=VERTEX_POINT('',#19194);
#4913=VERTEX_POINT('',#19197);
#4914=VERTEX_POINT('',#19199);
#4915=VERTEX_POINT('',#19201);
#4916=VERTEX_POINT('',#19203);
#4917=VERTEX_POINT('',#19206);
#4918=VERTEX_POINT('',#19208);
#4919=VERTEX_POINT('',#19210);
#4920=VERTEX_POINT('',#19215);
#4921=VERTEX_POINT('',#19217);
#4922=VERTEX_POINT('',#19221);
#4923=VERTEX_POINT('',#19222);
#4924=VERTEX_POINT('',#19224);
#4925=VERTEX_POINT('',#19226);
#4926=VERTEX_POINT('',#19228);
#4927=VERTEX_POINT('',#19232);
#4928=VERTEX_POINT('',#19234);
#4929=VERTEX_POINT('',#19236);
#4930=VERTEX_POINT('',#19238);
#4931=VERTEX_POINT('',#19242);
#4932=VERTEX_POINT('',#19243);
#4933=VERTEX_POINT('',#19245);
#4934=VERTEX_POINT('',#19247);
#4935=VERTEX_POINT('',#19249);
#4936=VERTEX_POINT('',#19253);
#4937=VERTEX_POINT('',#19254);
#4938=VERTEX_POINT('',#19256);
#4939=VERTEX_POINT('',#19258);
#4940=VERTEX_POINT('',#19260);
#4941=VERTEX_POINT('',#19262);
#4942=VERTEX_POINT('',#19264);
#4943=VERTEX_POINT('',#19266);
#4944=VERTEX_POINT('',#19269);
#4945=VERTEX_POINT('',#19270);
#4946=VERTEX_POINT('',#19272);
#4947=VERTEX_POINT('',#19274);
#4948=VERTEX_POINT('',#19276);
#4949=VERTEX_POINT('',#19278);
#4950=VERTEX_POINT('',#19280);
#4951=VERTEX_POINT('',#19282);
#4952=VERTEX_POINT('',#19286);
#4953=VERTEX_POINT('',#19289);
#4954=VERTEX_POINT('',#19293);
#4955=VERTEX_POINT('',#19295);
#4956=VERTEX_POINT('',#19297);
#4957=VERTEX_POINT('',#19301);
#4958=VERTEX_POINT('',#19302);
#4959=VERTEX_POINT('',#19304);
#4960=VERTEX_POINT('',#19309);
#4961=VERTEX_POINT('',#19311);
#4962=VERTEX_POINT('',#19328);
#4963=VERTEX_POINT('',#19332);
#4964=VERTEX_POINT('',#19333);
#4965=VERTEX_POINT('',#19348);
#4966=VERTEX_POINT('',#19350);
#4967=VERTEX_POINT('',#19380);
#4968=VERTEX_POINT('',#20727);
#4969=VERTEX_POINT('',#20729);
#4970=VERTEX_POINT('',#20733);
#4971=VERTEX_POINT('',#20734);
#4972=VERTEX_POINT('',#20736);
#4973=VERTEX_POINT('',#20738);
#4974=VERTEX_POINT('',#20740);
#4975=VERTEX_POINT('',#20744);
#4976=VERTEX_POINT('',#20746);
#4977=VERTEX_POINT('',#20748);
#4978=VERTEX_POINT('',#20750);
#4979=VERTEX_POINT('',#20754);
#4980=VERTEX_POINT('',#20755);
#4981=VERTEX_POINT('',#20757);
#4982=VERTEX_POINT('',#20759);
#4983=VERTEX_POINT('',#20761);
#4984=VERTEX_POINT('',#20765);
#4985=VERTEX_POINT('',#20768);
#4986=VERTEX_POINT('',#20772);
#4987=VERTEX_POINT('',#20774);
#4988=VERTEX_POINT('',#20776);
#4989=VERTEX_POINT('',#20780);
#4990=VERTEX_POINT('',#20781);
#4991=VERTEX_POINT('',#20784);
#4992=VERTEX_POINT('',#20788);
#4993=VERTEX_POINT('',#20790);
#4994=VERTEX_POINT('',#20794);
#4995=VERTEX_POINT('',#20808);
#4996=VERTEX_POINT('',#20809);
#4997=VERTEX_POINT('',#20821);
#4998=VERTEX_POINT('',#20823);
#4999=VERTEX_POINT('',#20837);
#5000=VERTEX_POINT('',#22252);
#5001=VERTEX_POINT('',#22253);
#5002=VERTEX_POINT('',#22255);
#5003=VERTEX_POINT('',#22257);
#5004=VERTEX_POINT('',#22261);
#5005=VERTEX_POINT('',#22262);
#5006=VERTEX_POINT('',#22264);
#5007=VERTEX_POINT('',#22266);
#5008=VERTEX_POINT('',#22268);
#5009=VERTEX_POINT('',#22270);
#5010=VERTEX_POINT('',#22274);
#5011=VERTEX_POINT('',#22275);
#5012=VERTEX_POINT('',#22277);
#5013=VERTEX_POINT('',#22279);
#5014=VERTEX_POINT('',#22283);
#5015=VERTEX_POINT('',#22284);
#5016=VERTEX_POINT('',#22286);
#5017=VERTEX_POINT('',#22288);
#5018=VERTEX_POINT('',#22292);
#5019=VERTEX_POINT('',#22293);
#5020=VERTEX_POINT('',#22295);
#5021=VERTEX_POINT('',#22297);
#5022=VERTEX_POINT('',#22301);
#5023=VERTEX_POINT('',#22302);
#5024=VERTEX_POINT('',#22304);
#5025=VERTEX_POINT('',#22308);
#5026=VERTEX_POINT('',#22309);
#5027=VERTEX_POINT('',#22311);
#5028=VERTEX_POINT('',#22315);
#5029=VERTEX_POINT('',#22316);
#5030=VERTEX_POINT('',#22318);
#5031=VERTEX_POINT('',#22320);
#5032=VERTEX_POINT('',#22324);
#5033=VERTEX_POINT('',#22325);
#5034=VERTEX_POINT('',#22327);
#5035=VERTEX_POINT('',#22331);
#5036=VERTEX_POINT('',#22332);
#5037=VERTEX_POINT('',#22334);
#5038=VERTEX_POINT('',#22338);
#5039=VERTEX_POINT('',#22339);
#5040=VERTEX_POINT('',#22341);
#5041=VERTEX_POINT('',#22343);
#5042=VERTEX_POINT('',#22347);
#5043=VERTEX_POINT('',#22348);
#5044=VERTEX_POINT('',#22350);
#5045=VERTEX_POINT('',#22352);
#5046=VERTEX_POINT('',#22356);
#5047=VERTEX_POINT('',#22357);
#5048=VERTEX_POINT('',#22359);
#5049=VERTEX_POINT('',#22361);
#5050=VERTEX_POINT('',#22365);
#5051=VERTEX_POINT('',#22366);
#5052=VERTEX_POINT('',#22368);
#5053=VERTEX_POINT('',#22370);
#5054=VERTEX_POINT('',#22374);
#5055=VERTEX_POINT('',#22375);
#5056=VERTEX_POINT('',#22380);
#5057=VERTEX_POINT('',#22382);
#5058=VERTEX_POINT('',#22386);
#5059=VERTEX_POINT('',#22387);
#5060=VERTEX_POINT('',#22389);
#5061=VERTEX_POINT('',#22391);
#5062=VERTEX_POINT('',#22395);
#5063=VERTEX_POINT('',#22397);
#5064=VERTEX_POINT('',#22401);
#5065=VERTEX_POINT('',#22402);
#5066=VERTEX_POINT('',#22407);
#5067=VERTEX_POINT('',#22408);
#5068=VERTEX_POINT('',#22410);
#5069=VERTEX_POINT('',#22412);
#5070=VERTEX_POINT('',#22416);
#5071=VERTEX_POINT('',#22417);
#5072=VERTEX_POINT('',#22419);
#5073=VERTEX_POINT('',#22421);
#5074=VERTEX_POINT('',#22425);
#5075=VERTEX_POINT('',#22426);
#5076=VERTEX_POINT('',#22428);
#5077=VERTEX_POINT('',#22430);
#5078=VERTEX_POINT('',#22434);
#5079=VERTEX_POINT('',#22435);
#5080=VERTEX_POINT('',#22437);
#5081=VERTEX_POINT('',#22439);
#5832=EDGE_CURVE('',#4768,#4769,#2744,.T.);
#5833=EDGE_CURVE('',#4770,#4768,#2688,.T.);
#5834=EDGE_CURVE('',#4769,#4770,#2140,.T.);
#5835=EDGE_CURVE('',#4771,#4772,#2141,.T.);
#5836=EDGE_CURVE('',#4772,#4771,#2142,.T.);
#5837=EDGE_CURVE('',#4772,#4773,#2143,.T.);
#5838=EDGE_CURVE('',#4773,#4773,#2144,.T.);
#5839=EDGE_CURVE('',#4774,#4775,#2145,.T.);
#5840=EDGE_CURVE('',#4776,#4774,#2745,.T.);
#5841=EDGE_CURVE('',#4776,#4777,#2146,.T.);
#5842=EDGE_CURVE('',#4775,#4777,#2746,.T.);
#5843=EDGE_CURVE('',#4778,#4779,#2147,.T.);
#5844=EDGE_CURVE('',#4779,#4780,#2148,.T.);
#5845=EDGE_CURVE('',#4781,#4780,#2747,.T.);
#5846=EDGE_CURVE('',#4782,#4781,#2149,.T.);
#5847=EDGE_CURVE('',#4778,#4782,#2748,.T.);
#5848=EDGE_CURVE('',#4783,#4784,#2150,.T.);
#5849=EDGE_CURVE('',#4785,#4783,#2749,.T.);
#5850=EDGE_CURVE('',#4785,#4786,#2151,.T.);
#5851=EDGE_CURVE('',#4784,#4786,#2750,.T.);
#5852=EDGE_CURVE('',#4787,#4788,#2152,.T.);
#5853=EDGE_CURVE('',#4787,#4789,#2153,.T.);
#5854=EDGE_CURVE('',#4789,#4788,#2154,.T.);
#5855=EDGE_CURVE('',#4790,#4791,#2155,.T.);
#5856=EDGE_CURVE('',#4791,#4792,#2156,.T.);
#5857=EDGE_CURVE('',#4790,#4792,#2157,.T.);
#5858=EDGE_CURVE('',#4793,#4794,#2158,.T.);
#5859=EDGE_CURVE('',#4794,#4795,#2159,.T.);
#5860=EDGE_CURVE('',#4793,#4795,#2160,.T.);
#5861=EDGE_CURVE('',#4796,#4797,#2161,.T.);
#5862=EDGE_CURVE('',#4796,#4798,#2162,.T.);
#5863=EDGE_CURVE('',#4798,#4797,#2163,.T.);
#5864=EDGE_CURVE('',#4799,#4799,#2164,.T.);
#5865=EDGE_CURVE('',#4799,#4800,#2165,.T.);
#5866=EDGE_CURVE('',#4801,#4800,#2166,.T.);
#5867=EDGE_CURVE('',#4800,#4801,#2167,.T.);
#5868=EDGE_CURVE('',#4802,#4803,#2168,.T.);
#5869=EDGE_CURVE('',#4803,#4802,#2169,.T.);
#5870=EDGE_CURVE('',#4803,#4804,#2170,.T.);
#5871=EDGE_CURVE('',#4804,#4804,#2171,.T.);
#5872=EDGE_CURVE('',#4805,#4805,#2172,.T.);
#5873=EDGE_CURVE('',#4805,#4806,#2751,.T.);
#5874=EDGE_CURVE('',#4806,#4806,#2173,.T.);
#5875=EDGE_CURVE('',#4807,#4807,#2174,.T.);
#5876=EDGE_CURVE('',#4807,#4805,#2752,.T.);
#5877=EDGE_CURVE('',#4808,#4808,#2175,.T.);
#5878=EDGE_CURVE('',#4808,#4809,#2753,.T.);
#5879=EDGE_CURVE('',#4809,#4809,#2176,.T.);
#5880=EDGE_CURVE('',#4810,#4810,#2177,.T.);
#5881=EDGE_CURVE('',#4810,#4808,#2754,.T.);
#5882=EDGE_CURVE('',#4811,#4811,#2178,.T.);
#5883=EDGE_CURVE('',#4811,#4812,#2755,.T.);
#5884=EDGE_CURVE('',#4812,#4812,#2179,.T.);
#5885=EDGE_CURVE('',#4813,#4813,#2180,.T.);
#5886=EDGE_CURVE('',#4813,#4811,#2756,.T.);
#5887=EDGE_CURVE('',#4814,#4814,#2181,.T.);
#5888=EDGE_CURVE('',#4814,#4815,#2757,.T.);
#5889=EDGE_CURVE('',#4815,#4815,#2182,.T.);
#5890=EDGE_CURVE('',#4816,#4816,#2183,.T.);
#5891=EDGE_CURVE('',#4816,#4814,#2758,.T.);
#5892=EDGE_CURVE('',#4817,#4817,#2184,.T.);
#5893=EDGE_CURVE('',#4817,#4818,#2759,.T.);
#5894=EDGE_CURVE('',#4818,#4818,#2185,.T.);
#5895=EDGE_CURVE('',#4819,#4819,#2186,.T.);
#5896=EDGE_CURVE('',#4819,#4817,#2760,.T.);
#5897=EDGE_CURVE('',#4820,#4820,#2187,.T.);
#5898=EDGE_CURVE('',#4820,#4821,#2761,.T.);
#5899=EDGE_CURVE('',#4821,#4821,#2188,.T.);
#5900=EDGE_CURVE('',#4822,#4822,#2189,.T.);
#5901=EDGE_CURVE('',#4822,#4820,#2762,.T.);
#5902=EDGE_CURVE('',#4802,#4801,#2763,.T.);
#5903=EDGE_CURVE('',#4823,#4823,#2190,.T.);
#5904=EDGE_CURVE('',#4823,#4824,#2764,.T.);
#5905=EDGE_CURVE('',#4824,#4824,#2191,.T.);
#5906=EDGE_CURVE('',#4825,#4826,#2192,.T.);
#5907=EDGE_CURVE('',#4826,#4825,#2193,.T.);
#5908=EDGE_CURVE('',#4826,#4827,#2765,.T.);
#5909=EDGE_CURVE('',#4827,#4827,#2194,.T.);
#5910=EDGE_CURVE('',#4825,#4823,#2766,.T.);
#5911=EDGE_CURVE('',#4828,#4828,#2195,.T.);
#5912=EDGE_CURVE('',#4828,#4829,#2767,.T.);
#5913=EDGE_CURVE('',#4829,#4829,#2196,.T.);
#5914=EDGE_CURVE('',#4830,#4830,#2197,.T.);
#5915=EDGE_CURVE('',#4830,#4831,#2768,.T.);
#5916=EDGE_CURVE('',#4831,#4831,#2198,.T.);
#5917=EDGE_CURVE('',#4832,#4832,#2199,.T.);
#5918=EDGE_CURVE('',#4832,#4833,#2769,.T.);
#5919=EDGE_CURVE('',#4833,#4833,#2200,.T.);
#5920=EDGE_CURVE('',#4834,#4834,#2201,.T.);
#5921=EDGE_CURVE('',#4834,#4835,#2770,.T.);
#5922=EDGE_CURVE('',#4835,#4835,#2202,.T.);
#5923=EDGE_CURVE('',#4836,#4837,#2203,.T.);
#5924=EDGE_CURVE('',#4837,#4838,#2771,.T.);
#5925=EDGE_CURVE('',#4839,#4838,#2204,.T.);
#5926=EDGE_CURVE('',#4839,#4836,#2772,.T.);
#5927=EDGE_CURVE('',#4840,#4769,#2205,.T.);
#5928=EDGE_CURVE('',#4836,#4840,#2689,.T.);
#5929=EDGE_CURVE('',#4841,#4839,#2690,.T.);
#5930=EDGE_CURVE('',#4842,#4841,#2206,.T.);
#5931=EDGE_CURVE('',#4843,#4842,#2691,.T.);
#5932=EDGE_CURVE('',#4844,#4843,#2773,.T.);
#5933=EDGE_CURVE('',#4844,#4844,#2207,.T.);
#5934=EDGE_CURVE('',#4843,#4768,#2774,.T.);
#5935=EDGE_CURVE('',#4845,#4846,#2208,.T.);
#5936=EDGE_CURVE('',#4847,#4845,#2209,.T.);
#5937=EDGE_CURVE('',#4848,#4847,#2775,.T.);
#5938=EDGE_CURVE('',#4848,#4849,#2210,.T.);
#5939=EDGE_CURVE('',#4849,#4850,#2211,.T.);
#5940=EDGE_CURVE('',#4846,#4850,#2776,.T.);
#5941=EDGE_CURVE('',#4771,#4851,#2777,.T.);
#5942=EDGE_CURVE('',#4852,#4851,#2778,.T.);
#5943=EDGE_CURVE('',#4852,#4853,#2779,.T.);
#5944=EDGE_CURVE('',#4853,#4853,#2212,.T.);
#5945=EDGE_CURVE('',#4852,#4854,#2692,.T.);
#5946=EDGE_CURVE('',#4854,#4855,#2213,.T.);
#5947=EDGE_CURVE('',#4855,#4848,#2693,.T.);
#5948=EDGE_CURVE('',#4847,#4856,#2694,.T.);
#5949=EDGE_CURVE('',#4856,#4857,#2214,.T.);
#5950=EDGE_CURVE('',#4857,#4851,#2695,.T.);
#5951=EDGE_CURVE('',#4777,#4858,#2215,.T.);
#5952=EDGE_CURVE('',#4858,#4859,#2696,.T.);
#5953=EDGE_CURVE('',#4859,#4860,#2780,.T.);
#5954=EDGE_CURVE('',#4860,#4861,#2697,.T.);
#5955=EDGE_CURVE('',#4861,#4784,#2216,.T.);
#5956=EDGE_CURVE('',#4862,#4786,#2698,.T.);
#5957=EDGE_CURVE('',#4862,#4863,#2217,.T.);
#5958=EDGE_CURVE('',#4863,#4864,#2699,.T.);
#5959=EDGE_CURVE('',#4864,#4865,#2781,.T.);
#5960=EDGE_CURVE('',#4865,#4866,#2700,.T.);
#5961=EDGE_CURVE('',#4866,#4867,#2218,.T.);
#5962=EDGE_CURVE('',#4778,#4867,#2701,.T.);
#5963=EDGE_CURVE('',#4782,#4868,#2219,.T.);
#5964=EDGE_CURVE('',#4868,#4869,#2702,.T.);
#5965=EDGE_CURVE('',#4869,#4870,#2782,.T.);
#5966=EDGE_CURVE('',#4870,#4871,#2703,.T.);
#5967=EDGE_CURVE('',#4871,#4775,#2220,.T.);
#5968=EDGE_CURVE('',#4797,#4872,#2221,.T.);
#5969=EDGE_CURVE('',#4872,#4873,#2704,.T.);
#5970=EDGE_CURVE('',#4873,#4874,#2783,.T.);
#5971=EDGE_CURVE('',#4874,#4875,#2705,.T.);
#5972=EDGE_CURVE('',#4875,#4793,#2222,.T.);
#5973=EDGE_CURVE('',#4793,#4790,#2784,.T.);
#5974=EDGE_CURVE('',#4790,#4876,#2223,.T.);
#5975=EDGE_CURVE('',#4876,#4877,#2706,.T.);
#5976=EDGE_CURVE('',#4877,#4878,#2785,.T.);
#5977=EDGE_CURVE('',#4878,#4879,#2707,.T.);
#5978=EDGE_CURVE('',#4879,#4788,#2224,.T.);
#5979=EDGE_CURVE('',#4788,#4880,#2786,.T.);
#5980=EDGE_CURVE('',#4881,#4880,#2708,.T.);
#5981=EDGE_CURVE('',#4881,#4882,#2225,.T.);
#5982=EDGE_CURVE('',#4882,#4883,#2709,.T.);
#5983=EDGE_CURVE('',#4883,#4884,#2787,.T.);
#5984=EDGE_CURVE('',#4884,#4885,#2710,.T.);
#5985=EDGE_CURVE('',#4885,#4886,#2226,.T.);
#5986=EDGE_CURVE('',#4887,#4886,#2711,.T.);
#5987=EDGE_CURVE('',#4887,#4797,#2788,.T.);
#5988=EDGE_CURVE('',#4888,#4889,#2789,.T.);
#5989=EDGE_CURVE('',#4889,#4890,#2790,.T.);
#5990=EDGE_CURVE('',#4890,#4891,#2791,.T.);
#5991=EDGE_CURVE('',#4891,#4892,#2792,.T.);
#5992=EDGE_CURVE('',#4892,#4893,#2793,.T.);
#5993=EDGE_CURVE('',#4893,#4888,#2794,.T.);
#5994=EDGE_CURVE('',#4894,#4895,#2795,.T.);
#5995=EDGE_CURVE('',#4895,#4896,#2796,.T.);
#5996=EDGE_CURVE('',#4896,#4897,#2797,.T.);
#5997=EDGE_CURVE('',#4897,#4898,#2798,.T.);
#5998=EDGE_CURVE('',#4898,#4789,#2799,.T.);
#5999=EDGE_CURVE('',#4789,#4899,#2800,.T.);
#6000=EDGE_CURVE('',#4900,#4899,#2227,.T.);
#6001=EDGE_CURVE('',#4900,#4901,#2801,.T.);
#6002=EDGE_CURVE('',#4902,#4901,#2228,.T.);
#6003=EDGE_CURVE('',#4902,#4791,#2802,.T.);
#6004=EDGE_CURVE('',#4791,#4795,#2803,.T.);
#6005=EDGE_CURVE('',#4795,#4903,#2804,.T.);
#6006=EDGE_CURVE('',#4904,#4903,#2229,.T.);
#6007=EDGE_CURVE('',#4904,#4905,#2805,.T.);
#6008=EDGE_CURVE('',#4906,#4905,#2230,.T.);
#6009=EDGE_CURVE('',#4906,#4796,#2806,.T.);
#6010=EDGE_CURVE('',#4796,#4907,#2807,.T.);
#6011=EDGE_CURVE('',#4907,#4894,#2808,.T.);
#6012=EDGE_CURVE('',#4908,#4781,#2809,.T.);
#6013=EDGE_CURVE('',#4780,#4909,#2810,.T.);
#6014=EDGE_CURVE('',#4909,#4910,#2811,.T.);
#6015=EDGE_CURVE('',#4910,#4911,#2812,.T.);
#6016=EDGE_CURVE('',#4911,#4912,#2813,.T.);
#6017=EDGE_CURVE('',#4912,#4785,#2814,.T.);
#6018=EDGE_CURVE('',#4783,#4913,#2815,.T.);
#6019=EDGE_CURVE('',#4914,#4913,#2231,.T.);
#6020=EDGE_CURVE('',#4914,#4915,#2816,.T.);
#6021=EDGE_CURVE('',#4916,#4915,#2232,.T.);
#6022=EDGE_CURVE('',#4916,#4776,#2817,.T.);
#6023=EDGE_CURVE('',#4774,#4917,#2818,.T.);
#6024=EDGE_CURVE('',#4918,#4917,#2233,.T.);
#6025=EDGE_CURVE('',#4918,#4919,#2819,.T.);
#6026=EDGE_CURVE('',#4908,#4919,#2234,.T.);
#6027=EDGE_CURVE('',#4920,#4846,#2235,.T.);
#6028=EDGE_CURVE('',#4850,#4921,#2236,.T.);
#6029=EDGE_CURVE('',#4921,#4920,#2820,.T.);
#6030=EDGE_CURVE('',#4922,#4923,#2237,.T.);
#6031=EDGE_CURVE('',#4923,#4924,#2238,.T.);
#6032=EDGE_CURVE('',#4924,#4925,#2239,.T.);
#6033=EDGE_CURVE('',#4925,#4926,#2821,.T.);
#6034=EDGE_CURVE('',#4926,#4922,#2240,.T.);
#6035=EDGE_CURVE('',#4851,#4927,#2241,.T.);
#6036=EDGE_CURVE('',#4927,#4928,#2242,.T.);
#6037=EDGE_CURVE('',#4929,#4928,#2822,.T.);
#6038=EDGE_CURVE('',#4929,#4930,#2243,.T.);
#6039=EDGE_CURVE('',#4930,#4852,#2244,.T.);
#6040=EDGE_CURVE('',#4931,#4932,#2245,.T.);
#6041=EDGE_CURVE('',#4932,#4933,#2246,.T.);
#6042=EDGE_CURVE('',#4933,#4934,#2247,.T.);
#6043=EDGE_CURVE('',#4934,#4935,#2248,.T.);
#6044=EDGE_CURVE('',#4935,#4931,#2823,.T.);
#6045=EDGE_CURVE('',#4936,#4937,#2824,.T.);
#6046=EDGE_CURVE('',#4937,#4938,#125,.T.);
#6047=EDGE_CURVE('',#4938,#4939,#2825,.T.);
#6048=EDGE_CURVE('',#4939,#4940,#126,.T.);
#6049=EDGE_CURVE('',#4940,#4941,#2826,.T.);
#6050=EDGE_CURVE('',#4941,#4942,#127,.T.);
#6051=EDGE_CURVE('',#4942,#4943,#2827,.T.);
#6052=EDGE_CURVE('',#4943,#4936,#128,.T.);
#6053=EDGE_CURVE('',#4944,#4945,#2828,.T.);
#6054=EDGE_CURVE('',#4946,#4944,#129,.T.);
#6055=EDGE_CURVE('',#4947,#4946,#2829,.T.);
#6056=EDGE_CURVE('',#4948,#4947,#130,.T.);
#6057=EDGE_CURVE('',#4949,#4948,#2830,.T.);
#6058=EDGE_CURVE('',#4950,#4949,#131,.T.);
#6059=EDGE_CURVE('',#4951,#4950,#2831,.T.);
#6060=EDGE_CURVE('',#4945,#4951,#132,.T.);
#6061=EDGE_CURVE('',#4928,#4952,#2249,.T.);
#6062=EDGE_CURVE('',#4952,#4943,#2832,.T.);
#6063=EDGE_CURVE('',#4942,#4953,#2833,.T.);
#6064=EDGE_CURVE('',#4953,#4929,#2250,.T.);
#6065=EDGE_CURVE('',#4940,#4954,#2834,.T.);
#6066=EDGE_CURVE('',#4954,#4955,#2251,.T.);
#6067=EDGE_CURVE('',#4955,#4956,#2835,.T.);
#6068=EDGE_CURVE('',#4956,#4941,#2836,.T.);
#6069=EDGE_CURVE('',#4957,#4958,#2837,.T.);
#6070=EDGE_CURVE('',#4958,#4959,#2252,.T.);
#6071=EDGE_CURVE('',#4959,#4937,#2838,.T.);
#6072=EDGE_CURVE('',#4936,#4957,#2839,.T.);
#6073=EDGE_CURVE('',#4938,#4960,#2840,.T.);
#6074=EDGE_CURVE('',#4960,#4961,#2841,.T.);
#6075=EDGE_CURVE('',#4961,#4939,#2842,.T.);
#6076=EDGE_CURVE('',#4955,#4926,#2712,.T.);
#6077=EDGE_CURVE('',#4925,#4962,#2253,.T.);
#6078=EDGE_CURVE('',#4962,#4956,#2254,.T.);
#6079=EDGE_CURVE('',#4963,#4964,#2713,.T.);
#6080=EDGE_CURVE('',#4964,#4920,#2255,.T.);
#6081=EDGE_CURVE('',#4921,#4965,#2256,.T.);
#6082=EDGE_CURVE('',#4965,#4966,#2714,.T.);
#6083=EDGE_CURVE('',#4966,#4961,#2257,.T.);
#6084=EDGE_CURVE('',#4960,#4963,#2258,.T.);
#6085=EDGE_CURVE('',#4935,#4958,#2715,.T.);
#6086=EDGE_CURVE('',#4957,#4967,#2259,.T.);
#6087=EDGE_CURVE('',#4967,#4931,#2260,.T.);
#6088=EDGE_CURVE('',#4960,#4959,#2261,.T.);
#6089=EDGE_CURVE('',#4963,#4958,#2262,.T.);
#6090=EDGE_CURVE('',#4964,#4935,#2263,.T.);
#6091=EDGE_CURVE('',#4920,#4934,#2264,.T.);
#6092=EDGE_CURVE('',#4933,#4846,#2716,.T.);
#6093=EDGE_CURVE('',#4954,#4961,#2265,.T.);
#6094=EDGE_CURVE('',#4955,#4966,#2266,.T.);
#6095=EDGE_CURVE('',#4926,#4965,#2267,.T.);
#6096=EDGE_CURVE('',#4922,#4921,#2268,.T.);
#6097=EDGE_CURVE('',#4850,#4923,#2717,.T.);
#6098=EDGE_CURVE('',#4957,#4952,#2269,.T.);
#6099=EDGE_CURVE('',#4967,#4928,#2270,.T.);
#6100=EDGE_CURVE('',#4931,#4927,#2271,.T.);
#6101=EDGE_CURVE('',#4851,#4932,#2718,.T.);
#6102=EDGE_CURVE('',#4953,#4956,#2272,.T.);
#6103=EDGE_CURVE('',#4929,#4962,#2273,.T.);
#6104=EDGE_CURVE('',#4930,#4925,#2274,.T.);
#6105=EDGE_CURVE('',#4924,#4852,#2719,.T.);
#6106=EDGE_CURVE('',#4854,#4924,#2275,.T.);
#6107=EDGE_CURVE('',#4855,#4923,#2276,.T.);
#6108=EDGE_CURVE('',#4856,#4933,#2277,.T.);
#6109=EDGE_CURVE('',#4857,#4932,#2278,.T.);
#6110=EDGE_CURVE('',#4840,#4770,#2279,.T.);
#6111=EDGE_CURVE('',#4968,#4837,#2280,.T.);
#6112=EDGE_CURVE('',#4969,#4968,#2843,.T.);
#6113=EDGE_CURVE('',#4838,#4969,#2281,.T.);
#6114=EDGE_CURVE('',#4970,#4971,#2282,.T.);
#6115=EDGE_CURVE('',#4972,#4970,#2283,.T.);
#6116=EDGE_CURVE('',#4973,#4972,#2844,.T.);
#6117=EDGE_CURVE('',#4974,#4973,#2284,.T.);
#6118=EDGE_CURVE('',#4971,#4974,#2285,.T.);
#6119=EDGE_CURVE('',#4975,#4843,#2286,.T.);
#6120=EDGE_CURVE('',#4976,#4975,#2287,.T.);
#6121=EDGE_CURVE('',#4976,#4977,#2845,.T.);
#6122=EDGE_CURVE('',#4978,#4977,#2288,.T.);
#6123=EDGE_CURVE('',#4768,#4978,#2289,.T.);
#6124=EDGE_CURVE('',#4979,#4980,#2290,.T.);
#6125=EDGE_CURVE('',#4981,#4979,#2846,.T.);
#6126=EDGE_CURVE('',#4982,#4981,#2291,.T.);
#6127=EDGE_CURVE('',#4983,#4982,#2292,.T.);
#6128=EDGE_CURVE('',#4980,#4983,#2293,.T.);
#6129=EDGE_CURVE('',#4984,#4976,#2294,.T.);
#6130=EDGE_CURVE('',#4947,#4984,#2847,.T.);
#6131=EDGE_CURVE('',#4985,#4946,#2848,.T.);
#6132=EDGE_CURVE('',#4977,#4985,#2295,.T.);
#6133=EDGE_CURVE('',#4949,#4986,#2849,.T.);
#6134=EDGE_CURVE('',#4987,#4948,#2850,.T.);
#6135=EDGE_CURVE('',#4988,#4987,#2851,.T.);
#6136=EDGE_CURVE('',#4986,#4988,#2296,.T.);
#6137=EDGE_CURVE('',#4989,#4990,#2852,.T.);
#6138=EDGE_CURVE('',#4944,#4989,#2853,.T.);
#6139=EDGE_CURVE('',#4991,#4945,#2854,.T.);
#6140=EDGE_CURVE('',#4990,#4991,#2297,.T.);
#6141=EDGE_CURVE('',#4992,#4950,#2855,.T.);
#6142=EDGE_CURVE('',#4993,#4992,#2856,.T.);
#6143=EDGE_CURVE('',#4951,#4993,#2857,.T.);
#6144=EDGE_CURVE('',#4994,#4987,#2298,.T.);
#6145=EDGE_CURVE('',#4973,#4994,#2299,.T.);
#6146=EDGE_CURVE('',#4988,#4972,#2720,.T.);
#6147=EDGE_CURVE('',#4995,#4996,#2721,.T.);
#6148=EDGE_CURVE('',#4993,#4995,#2300,.T.);
#6149=EDGE_CURVE('',#4997,#4992,#2301,.T.);
#6150=EDGE_CURVE('',#4998,#4997,#2722,.T.);
#6151=EDGE_CURVE('',#4969,#4998,#2302,.T.);
#6152=EDGE_CURVE('',#4996,#4968,#2303,.T.);
#6153=EDGE_CURVE('',#4999,#4979,#2304,.T.);
#6154=EDGE_CURVE('',#4989,#4999,#2305,.T.);
#6155=EDGE_CURVE('',#4981,#4990,#2723,.T.);
#6156=EDGE_CURVE('',#4993,#4991,#2306,.T.);
#6157=EDGE_CURVE('',#4995,#4990,#2307,.T.);
#6158=EDGE_CURVE('',#4996,#4981,#2308,.T.);
#6159=EDGE_CURVE('',#4968,#4982,#2309,.T.);
#6160=EDGE_CURVE('',#4983,#4837,#2724,.T.);
#6161=EDGE_CURVE('',#4986,#4992,#2310,.T.);
#6162=EDGE_CURVE('',#4988,#4997,#2311,.T.);
#6163=EDGE_CURVE('',#4972,#4998,#2312,.T.);
#6164=EDGE_CURVE('',#4970,#4969,#2313,.T.);
#6165=EDGE_CURVE('',#4838,#4971,#2725,.T.);
#6166=EDGE_CURVE('',#4989,#4985,#2314,.T.);
#6167=EDGE_CURVE('',#4999,#4977,#2315,.T.);
#6168=EDGE_CURVE('',#4979,#4978,#2316,.T.);
#6169=EDGE_CURVE('',#4768,#4980,#2726,.T.);
#6170=EDGE_CURVE('',#4984,#4987,#2317,.T.);
#6171=EDGE_CURVE('',#4976,#4994,#2318,.T.);
#6172=EDGE_CURVE('',#4975,#4973,#2319,.T.);
#6173=EDGE_CURVE('',#4974,#4843,#2727,.T.);
#6174=EDGE_CURVE('',#4842,#4974,#2320,.T.);
#6175=EDGE_CURVE('',#4841,#4971,#2321,.T.);
#6176=EDGE_CURVE('',#4840,#4983,#2322,.T.);
#6177=EDGE_CURVE('',#4770,#4980,#2323,.T.);
#6178=EDGE_CURVE('',#5000,#5001,#2858,.T.);
#6179=EDGE_CURVE('',#5001,#5002,#2859,.T.);
#6180=EDGE_CURVE('',#5002,#5003,#2860,.T.);
#6181=EDGE_CURVE('',#5003,#5000,#2861,.T.);
#6182=EDGE_CURVE('',#5004,#5005,#2862,.T.);
#6183=EDGE_CURVE('',#5005,#5006,#2863,.T.);
#6184=EDGE_CURVE('',#5006,#5007,#2864,.T.);
#6185=EDGE_CURVE('',#5007,#5008,#2865,.T.);
#6186=EDGE_CURVE('',#5008,#5009,#2866,.T.);
#6187=EDGE_CURVE('',#5009,#5004,#2867,.T.);
#6188=EDGE_CURVE('',#5010,#5011,#2868,.T.);
#6189=EDGE_CURVE('',#5011,#5012,#2869,.T.);
#6190=EDGE_CURVE('',#5012,#5013,#2870,.T.);
#6191=EDGE_CURVE('',#5013,#5010,#2324,.T.);
#6192=EDGE_CURVE('',#5014,#5015,#2871,.T.);
#6193=EDGE_CURVE('',#5015,#5016,#2325,.T.);
#6194=EDGE_CURVE('',#5016,#5017,#2872,.T.);
#6195=EDGE_CURVE('',#5017,#5014,#2873,.T.);
#6196=EDGE_CURVE('',#5018,#5019,#2874,.T.);
#6197=EDGE_CURVE('',#5019,#5020,#2875,.T.);
#6198=EDGE_CURVE('',#5020,#5021,#2876,.T.);
#6199=EDGE_CURVE('',#5021,#5018,#2877,.T.);
#6200=EDGE_CURVE('',#5022,#5023,#2878,.T.);
#6201=EDGE_CURVE('',#5023,#5024,#2326,.T.);
#6202=EDGE_CURVE('',#5024,#5022,#2879,.T.);
#6203=EDGE_CURVE('',#5025,#5026,#2880,.T.);
#6204=EDGE_CURVE('',#5026,#5027,#2327,.T.);
#6205=EDGE_CURVE('',#5027,#5025,#2881,.T.);
#6206=EDGE_CURVE('',#5028,#5029,#2882,.T.);
#6207=EDGE_CURVE('',#5029,#5030,#2883,.T.);
#6208=EDGE_CURVE('',#5030,#5031,#2884,.T.);
#6209=EDGE_CURVE('',#5031,#5028,#2885,.T.);
#6210=EDGE_CURVE('',#5032,#5033,#2886,.T.);
#6211=EDGE_CURVE('',#5033,#5034,#2328,.T.);
#6212=EDGE_CURVE('',#5034,#5032,#2887,.T.);
#6213=EDGE_CURVE('',#5035,#5036,#2888,.T.);
#6214=EDGE_CURVE('',#5036,#5037,#2329,.T.);
#6215=EDGE_CURVE('',#5037,#5035,#2889,.T.);
#6216=EDGE_CURVE('',#5038,#5039,#2890,.T.);
#6217=EDGE_CURVE('',#5039,#5040,#2891,.T.);
#6218=EDGE_CURVE('',#5040,#5041,#2892,.T.);
#6219=EDGE_CURVE('',#5041,#5038,#2893,.T.);
#6220=EDGE_CURVE('',#5042,#5043,#2894,.T.);
#6221=EDGE_CURVE('',#5043,#5044,#2895,.T.);
#6222=EDGE_CURVE('',#5044,#5045,#2330,.T.);
#6223=EDGE_CURVE('',#5045,#5042,#2896,.T.);
#6224=EDGE_CURVE('',#5046,#5047,#2897,.T.);
#6225=EDGE_CURVE('',#5047,#5048,#2331,.T.);
#6226=EDGE_CURVE('',#5048,#5049,#2898,.T.);
#6227=EDGE_CURVE('',#5049,#5046,#2899,.T.);
#6228=EDGE_CURVE('',#5050,#5051,#2900,.T.);
#6229=EDGE_CURVE('',#5051,#5052,#2901,.T.);
#6230=EDGE_CURVE('',#5052,#5053,#2902,.T.);
#6231=EDGE_CURVE('',#5053,#5050,#2903,.T.);
#6232=EDGE_CURVE('',#5054,#5055,#2904,.T.);
#6233=EDGE_CURVE('',#5055,#4798,#2332,.T.);
#6234=EDGE_CURVE('',#4798,#5054,#2905,.T.);
#6235=EDGE_CURVE('',#5056,#4794,#2906,.T.);
#6236=EDGE_CURVE('',#4794,#5057,#2333,.T.);
#6237=EDGE_CURVE('',#5057,#5056,#2907,.T.);
#6238=EDGE_CURVE('',#5058,#5059,#2908,.T.);
#6239=EDGE_CURVE('',#5059,#5060,#2909,.T.);
#6240=EDGE_CURVE('',#5060,#5061,#2910,.T.);
#6241=EDGE_CURVE('',#5061,#5058,#2911,.T.);
#6242=EDGE_CURVE('',#5062,#4787,#2912,.T.);
#6243=EDGE_CURVE('',#4787,#5063,#2334,.T.);
#6244=EDGE_CURVE('',#5063,#5062,#2913,.T.);
#6245=EDGE_CURVE('',#5064,#5065,#2914,.T.);
#6246=EDGE_CURVE('',#5065,#4792,#2335,.T.);
#6247=EDGE_CURVE('',#4792,#5064,#2915,.T.);
#6248=EDGE_CURVE('',#5066,#5067,#2916,.T.);
#6249=EDGE_CURVE('',#5067,#5068,#2917,.T.);
#6250=EDGE_CURVE('',#5068,#5069,#2918,.T.);
#6251=EDGE_CURVE('',#5069,#5066,#2919,.T.);
#6252=EDGE_CURVE('',#5070,#5071,#2920,.T.);
#6253=EDGE_CURVE('',#5071,#5072,#2921,.T.);
#6254=EDGE_CURVE('',#5072,#5073,#2922,.T.);
#6255=EDGE_CURVE('',#5073,#5070,#2923,.T.);
#6256=EDGE_CURVE('',#5074,#5075,#2924,.T.);
#6257=EDGE_CURVE('',#5075,#5076,#2925,.T.);
#6258=EDGE_CURVE('',#5076,#5077,#2926,.T.);
#6259=EDGE_CURVE('',#5077,#5074,#2927,.T.);
#6260=EDGE_CURVE('',#5078,#5079,#2928,.T.);
#6261=EDGE_CURVE('',#5079,#5080,#2929,.T.);
#6262=EDGE_CURVE('',#5080,#5081,#2930,.T.);
#6263=EDGE_CURVE('',#5081,#5078,#2931,.T.);
#6264=EDGE_CURVE('',#5054,#4906,#2336,.T.);
#6265=EDGE_CURVE('',#5055,#5053,#2728,.T.);
#6266=EDGE_CURVE('',#5050,#5054,#2337,.T.);
#6267=EDGE_CURVE('',#4872,#5055,#2338,.T.);
#6268=EDGE_CURVE('',#5073,#5040,#2339,.T.);
#6269=EDGE_CURVE('',#4893,#5073,#2340,.T.);
#6270=EDGE_CURVE('',#5040,#4893,#2341,.T.);
#6271=EDGE_CURVE('',#4894,#5071,#2342,.T.);
#6272=EDGE_CURVE('',#5046,#4894,#2343,.T.);
#6273=EDGE_CURVE('',#5071,#5046,#2344,.T.);
#6274=EDGE_CURVE('',#5050,#4905,#2345,.T.);
#6275=EDGE_CURVE('',#4873,#5053,#2346,.T.);
#6276=EDGE_CURVE('',#4907,#4887,#2347,.T.);
#6277=EDGE_CURVE('',#5047,#4907,#2729,.T.);
#6278=EDGE_CURVE('',#5072,#5049,#2348,.T.);
#6279=EDGE_CURVE('',#4888,#5072,#2349,.T.);
#6280=EDGE_CURVE('',#5041,#4892,#2350,.T.);
#6281=EDGE_CURVE('',#5070,#5039,#2351,.T.);
#6282=EDGE_CURVE('',#4895,#5070,#2352,.T.);
#6283=EDGE_CURVE('',#5051,#4904,#2353,.T.);
#6284=EDGE_CURVE('',#5052,#5057,#2730,.T.);
#6285=EDGE_CURVE('',#5056,#5051,#2354,.T.);
#6286=EDGE_CURVE('',#4874,#5052,#2355,.T.);
#6287=EDGE_CURVE('',#5047,#4886,#2356,.T.);
#6288=EDGE_CURVE('',#4888,#5049,#2357,.T.);
#6289=EDGE_CURVE('',#5041,#5068,#2358,.T.);
#6290=EDGE_CURVE('',#5068,#4892,#2359,.T.);
#6291=EDGE_CURVE('',#4895,#5039,#2360,.T.);
#6292=EDGE_CURVE('',#5056,#4903,#2361,.T.);
#6293=EDGE_CURVE('',#4875,#5057,#2362,.T.);
#6294=EDGE_CURVE('',#5048,#4885,#2363,.T.);
#6295=EDGE_CURVE('',#4889,#5048,#2731,.T.);
#6296=EDGE_CURVE('',#5069,#4891,#2364,.T.);
#6297=EDGE_CURVE('',#5038,#5067,#2365,.T.);
#6298=EDGE_CURVE('',#4896,#5038,#2366,.T.);
#6299=EDGE_CURVE('',#4889,#4884,#2367,.T.);
#6300=EDGE_CURVE('',#5069,#5043,#2368,.T.);
#6301=EDGE_CURVE('',#5043,#4891,#2369,.T.);
#6302=EDGE_CURVE('',#4896,#5067,#2370,.T.);
#6303=EDGE_CURVE('',#4890,#4883,#2371,.T.);
#6304=EDGE_CURVE('',#5044,#4890,#2732,.T.);
#6305=EDGE_CURVE('',#5066,#5042,#2372,.T.);
#6306=EDGE_CURVE('',#4897,#5066,#2373,.T.);
#6307=EDGE_CURVE('',#5064,#4902,#2374,.T.);
#6308=EDGE_CURVE('',#5044,#4882,#2375,.T.);
#6309=EDGE_CURVE('',#4897,#5042,#2376,.T.);
#6310=EDGE_CURVE('',#5058,#4901,#2377,.T.);
#6311=EDGE_CURVE('',#5064,#5058,#2378,.T.);
#6312=EDGE_CURVE('',#5045,#4881,#2379,.T.);
#6313=EDGE_CURVE('',#4898,#5045,#2733,.T.);
#6314=EDGE_CURVE('',#5059,#4900,#2380,.T.);
#6315=EDGE_CURVE('',#5065,#5061,#2734,.T.);
#6316=EDGE_CURVE('',#4876,#5065,#2381,.T.);
#6317=EDGE_CURVE('',#4898,#4880,#2382,.T.);
#6318=EDGE_CURVE('',#5062,#4899,#2383,.T.);
#6319=EDGE_CURVE('',#5059,#5062,#2384,.T.);
#6320=EDGE_CURVE('',#4877,#5061,#2385,.T.);
#6321=EDGE_CURVE('',#5060,#5063,#2735,.T.);
#6322=EDGE_CURVE('',#4878,#5060,#2386,.T.);
#6323=EDGE_CURVE('',#4879,#5063,#2387,.T.);
#6324=EDGE_CURVE('',#5079,#5008,#2388,.T.);
#6325=EDGE_CURVE('',#5001,#5079,#2389,.T.);
#6326=EDGE_CURVE('',#5008,#5001,#2390,.T.);
#6327=EDGE_CURVE('',#5078,#4911,#2391,.T.);
#6328=EDGE_CURVE('',#4912,#5081,#2392,.T.);
#6329=EDGE_CURVE('',#5002,#5078,#2393,.T.);
#6330=EDGE_CURVE('',#5009,#5000,#2394,.T.);
#6331=EDGE_CURVE('',#5080,#5007,#2395,.T.);
#6332=EDGE_CURVE('',#5081,#5017,#2396,.T.);
#6333=EDGE_CURVE('',#5014,#5080,#2397,.T.);
#6334=EDGE_CURVE('',#4912,#5017,#2398,.T.);
#6335=EDGE_CURVE('',#5002,#4911,#2399,.T.);
#6336=EDGE_CURVE('',#5009,#5075,#2400,.T.);
#6337=EDGE_CURVE('',#5075,#5000,#2401,.T.);
#6338=EDGE_CURVE('',#5014,#5007,#2402,.T.);
#6339=EDGE_CURVE('',#4785,#5016,#2736,.T.);
#6340=EDGE_CURVE('',#5003,#4910,#2403,.T.);
#6341=EDGE_CURVE('',#5076,#5003,#2404,.T.);
#6342=EDGE_CURVE('',#5004,#5074,#2405,.T.);
#6343=EDGE_CURVE('',#5015,#5006,#2737,.T.);
#6344=EDGE_CURVE('',#4863,#5015,#2406,.T.);
#6345=EDGE_CURVE('',#5016,#4862,#2407,.T.);
#6346=EDGE_CURVE('',#5076,#4910,#2408,.T.);
#6347=EDGE_CURVE('',#5004,#5011,#2409,.T.);
#6348=EDGE_CURVE('',#5011,#5074,#2410,.T.);
#6349=EDGE_CURVE('',#4864,#5006,#2411,.T.);
#6350=EDGE_CURVE('',#5077,#4909,#2412,.T.);
#6351=EDGE_CURVE('',#5012,#5077,#2413,.T.);
#6352=EDGE_CURVE('',#5005,#5010,#2738,.T.);
#6353=EDGE_CURVE('',#4865,#5005,#2414,.T.);
#6354=EDGE_CURVE('',#4783,#5023,#2415,.T.);
#6355=EDGE_CURVE('',#5023,#4784,#2416,.T.);
#6356=EDGE_CURVE('',#5012,#4909,#2417,.T.);
#6357=EDGE_CURVE('',#4866,#5010,#2418,.T.);
#6358=EDGE_CURVE('',#5024,#4861,#2419,.T.);
#6359=EDGE_CURVE('',#5022,#5018,#2420,.T.);
#6360=EDGE_CURVE('',#5019,#5024,#2739,.T.);
#6361=EDGE_CURVE('',#4913,#5022,#2421,.T.);
#6362=EDGE_CURVE('',#5013,#4780,#2740,.T.);
#6363=EDGE_CURVE('',#4867,#5013,#2422,.T.);
#6364=EDGE_CURVE('',#5019,#4860,#2423,.T.);
#6365=EDGE_CURVE('',#4914,#5018,#2424,.T.);
#6366=EDGE_CURVE('',#5020,#4859,#2425,.T.);
#6367=EDGE_CURVE('',#5021,#5025,#2426,.T.);
#6368=EDGE_CURVE('',#5026,#5020,#2741,.T.);
#6369=EDGE_CURVE('',#4915,#5021,#2427,.T.);
#6370=EDGE_CURVE('',#4781,#5034,#2428,.T.);
#6371=EDGE_CURVE('',#5032,#4908,#2429,.T.);
#6372=EDGE_CURVE('',#5026,#4858,#2430,.T.);
#6373=EDGE_CURVE('',#4916,#5025,#2431,.T.);
#6374=EDGE_CURVE('',#5031,#4919,#2432,.T.);
#6375=EDGE_CURVE('',#5032,#5031,#2433,.T.);
#6376=EDGE_CURVE('',#4782,#5034,#2434,.T.);
#6377=EDGE_CURVE('',#5027,#4777,#2435,.T.);
#6378=EDGE_CURVE('',#4776,#5027,#2436,.T.);
#6379=EDGE_CURVE('',#5028,#4918,#2437,.T.);
#6380=EDGE_CURVE('',#5033,#5030,#2742,.T.);
#6381=EDGE_CURVE('',#4868,#5033,#2438,.T.);
#6382=EDGE_CURVE('',#5035,#4917,#2439,.T.);
#6383=EDGE_CURVE('',#5028,#5035,#2440,.T.);
#6384=EDGE_CURVE('',#4869,#5030,#2441,.T.);
#6385=EDGE_CURVE('',#5036,#4774,#2442,.T.);
#6386=EDGE_CURVE('',#5029,#5037,#2743,.T.);
#6387=EDGE_CURVE('',#4870,#5029,#2443,.T.);
#6388=EDGE_CURVE('',#5036,#4775,#2444,.T.);
#6389=EDGE_CURVE('',#4871,#5037,#2445,.T.);
#7528=ORIENTED_EDGE('',*,*,#5832,.F.);
#7529=ORIENTED_EDGE('',*,*,#5833,.F.);
#7530=ORIENTED_EDGE('',*,*,#5834,.F.);
#7531=ORIENTED_EDGE('',*,*,#5835,.F.);
#7532=ORIENTED_EDGE('',*,*,#5836,.F.);
#7533=ORIENTED_EDGE('',*,*,#5837,.T.);
#7534=ORIENTED_EDGE('',*,*,#5838,.F.);
#7535=ORIENTED_EDGE('',*,*,#5837,.F.);
#7536=ORIENTED_EDGE('',*,*,#5839,.F.);
#7537=ORIENTED_EDGE('',*,*,#5840,.F.);
#7538=ORIENTED_EDGE('',*,*,#5841,.T.);
#7539=ORIENTED_EDGE('',*,*,#5842,.F.);
#7540=ORIENTED_EDGE('',*,*,#5843,.T.);
#7541=ORIENTED_EDGE('',*,*,#5844,.T.);
#7542=ORIENTED_EDGE('',*,*,#5845,.F.);
#7543=ORIENTED_EDGE('',*,*,#5846,.F.);
#7544=ORIENTED_EDGE('',*,*,#5847,.F.);
#7545=ORIENTED_EDGE('',*,*,#5848,.F.);
#7546=ORIENTED_EDGE('',*,*,#5849,.F.);
#7547=ORIENTED_EDGE('',*,*,#5850,.T.);
#7548=ORIENTED_EDGE('',*,*,#5851,.F.);
#7549=ORIENTED_EDGE('',*,*,#5852,.F.);
#7550=ORIENTED_EDGE('',*,*,#5853,.T.);
#7551=ORIENTED_EDGE('',*,*,#5854,.T.);
#7552=ORIENTED_EDGE('',*,*,#5855,.T.);
#7553=ORIENTED_EDGE('',*,*,#5856,.T.);
#7554=ORIENTED_EDGE('',*,*,#5857,.F.);
#7555=ORIENTED_EDGE('',*,*,#5858,.T.);
#7556=ORIENTED_EDGE('',*,*,#5859,.T.);
#7557=ORIENTED_EDGE('',*,*,#5860,.F.);
#7558=ORIENTED_EDGE('',*,*,#5861,.F.);
#7559=ORIENTED_EDGE('',*,*,#5862,.T.);
#7560=ORIENTED_EDGE('',*,*,#5863,.T.);
#7561=ORIENTED_EDGE('',*,*,#5864,.F.);
#7562=ORIENTED_EDGE('',*,*,#5865,.T.);
#7563=ORIENTED_EDGE('',*,*,#5866,.F.);
#7564=ORIENTED_EDGE('',*,*,#5867,.F.);
#7565=ORIENTED_EDGE('',*,*,#5865,.F.);
#7566=ORIENTED_EDGE('',*,*,#5868,.F.);
#7567=ORIENTED_EDGE('',*,*,#5869,.F.);
#7568=ORIENTED_EDGE('',*,*,#5870,.T.);
#7569=ORIENTED_EDGE('',*,*,#5871,.F.);
#7570=ORIENTED_EDGE('',*,*,#5870,.F.);
#7571=ORIENTED_EDGE('',*,*,#5872,.F.);
#7572=ORIENTED_EDGE('',*,*,#5873,.T.);
#7573=ORIENTED_EDGE('',*,*,#5874,.T.);
#7574=ORIENTED_EDGE('',*,*,#5873,.F.);
#7575=ORIENTED_EDGE('',*,*,#5875,.F.);
#7576=ORIENTED_EDGE('',*,*,#5876,.T.);
#7577=ORIENTED_EDGE('',*,*,#5872,.T.);
#7578=ORIENTED_EDGE('',*,*,#5876,.F.);
#7579=ORIENTED_EDGE('',*,*,#5877,.F.);
#7580=ORIENTED_EDGE('',*,*,#5878,.T.);
#7581=ORIENTED_EDGE('',*,*,#5879,.T.);
#7582=ORIENTED_EDGE('',*,*,#5878,.F.);
#7583=ORIENTED_EDGE('',*,*,#5880,.F.);
#7584=ORIENTED_EDGE('',*,*,#5881,.T.);
#7585=ORIENTED_EDGE('',*,*,#5877,.T.);
#7586=ORIENTED_EDGE('',*,*,#5881,.F.);
#7587=ORIENTED_EDGE('',*,*,#5882,.F.);
#7588=ORIENTED_EDGE('',*,*,#5883,.T.);
#7589=ORIENTED_EDGE('',*,*,#5884,.T.);
#7590=ORIENTED_EDGE('',*,*,#5883,.F.);
#7591=ORIENTED_EDGE('',*,*,#5885,.F.);
#7592=ORIENTED_EDGE('',*,*,#5886,.T.);
#7593=ORIENTED_EDGE('',*,*,#5882,.T.);
#7594=ORIENTED_EDGE('',*,*,#5886,.F.);
#7595=ORIENTED_EDGE('',*,*,#5887,.F.);
#7596=ORIENTED_EDGE('',*,*,#5888,.T.);
#7597=ORIENTED_EDGE('',*,*,#5889,.T.);
#7598=ORIENTED_EDGE('',*,*,#5888,.F.);
#7599=ORIENTED_EDGE('',*,*,#5890,.F.);
#7600=ORIENTED_EDGE('',*,*,#5891,.T.);
#7601=ORIENTED_EDGE('',*,*,#5887,.T.);
#7602=ORIENTED_EDGE('',*,*,#5891,.F.);
#7603=ORIENTED_EDGE('',*,*,#5892,.F.);
#7604=ORIENTED_EDGE('',*,*,#5893,.T.);
#7605=ORIENTED_EDGE('',*,*,#5894,.T.);
#7606=ORIENTED_EDGE('',*,*,#5893,.F.);
#7607=ORIENTED_EDGE('',*,*,#5895,.F.);
#7608=ORIENTED_EDGE('',*,*,#5896,.T.);
#7609=ORIENTED_EDGE('',*,*,#5892,.T.);
#7610=ORIENTED_EDGE('',*,*,#5896,.F.);
#7611=ORIENTED_EDGE('',*,*,#5897,.F.);
#7612=ORIENTED_EDGE('',*,*,#5898,.T.);
#7613=ORIENTED_EDGE('',*,*,#5899,.T.);
#7614=ORIENTED_EDGE('',*,*,#5898,.F.);
#7615=ORIENTED_EDGE('',*,*,#5900,.F.);
#7616=ORIENTED_EDGE('',*,*,#5901,.T.);
#7617=ORIENTED_EDGE('',*,*,#5897,.T.);
#7618=ORIENTED_EDGE('',*,*,#5901,.F.);
#7619=ORIENTED_EDGE('',*,*,#5868,.T.);
#7620=ORIENTED_EDGE('',*,*,#5869,.T.);
#7621=ORIENTED_EDGE('',*,*,#5902,.T.);
#7622=ORIENTED_EDGE('',*,*,#5866,.T.);
#7623=ORIENTED_EDGE('',*,*,#5867,.T.);
#7624=ORIENTED_EDGE('',*,*,#5902,.F.);
#7625=ORIENTED_EDGE('',*,*,#5903,.F.);
#7626=ORIENTED_EDGE('',*,*,#5904,.T.);
#7627=ORIENTED_EDGE('',*,*,#5905,.F.);
#7628=ORIENTED_EDGE('',*,*,#5904,.F.);
#7629=ORIENTED_EDGE('',*,*,#5906,.F.);
#7630=ORIENTED_EDGE('',*,*,#5907,.F.);
#7631=ORIENTED_EDGE('',*,*,#5908,.T.);
#7632=ORIENTED_EDGE('',*,*,#5909,.F.);
#7633=ORIENTED_EDGE('',*,*,#5908,.F.);
#7634=ORIENTED_EDGE('',*,*,#5906,.T.);
#7635=ORIENTED_EDGE('',*,*,#5907,.T.);
#7636=ORIENTED_EDGE('',*,*,#5910,.T.);
#7637=ORIENTED_EDGE('',*,*,#5903,.T.);
#7638=ORIENTED_EDGE('',*,*,#5910,.F.);
#7639=ORIENTED_EDGE('',*,*,#5911,.F.);
#7640=ORIENTED_EDGE('',*,*,#5912,.T.);
#7641=ORIENTED_EDGE('',*,*,#5913,.T.);
#7642=ORIENTED_EDGE('',*,*,#5912,.F.);
#7643=ORIENTED_EDGE('',*,*,#5914,.F.);
#7644=ORIENTED_EDGE('',*,*,#5915,.T.);
#7645=ORIENTED_EDGE('',*,*,#5916,.T.);
#7646=ORIENTED_EDGE('',*,*,#5915,.F.);
#7647=ORIENTED_EDGE('',*,*,#5917,.T.);
#7648=ORIENTED_EDGE('',*,*,#5918,.T.);
#7649=ORIENTED_EDGE('',*,*,#5919,.T.);
#7650=ORIENTED_EDGE('',*,*,#5918,.F.);
#7651=ORIENTED_EDGE('',*,*,#5920,.T.);
#7652=ORIENTED_EDGE('',*,*,#5921,.T.);
#7653=ORIENTED_EDGE('',*,*,#5922,.T.);
#7654=ORIENTED_EDGE('',*,*,#5921,.F.);
#7655=ORIENTED_EDGE('',*,*,#5923,.T.);
#7656=ORIENTED_EDGE('',*,*,#5924,.T.);
#7657=ORIENTED_EDGE('',*,*,#5925,.F.);
#7658=ORIENTED_EDGE('',*,*,#5926,.T.);
#7659=ORIENTED_EDGE('',*,*,#5832,.T.);
#7660=ORIENTED_EDGE('',*,*,#5927,.F.);
#7661=ORIENTED_EDGE('',*,*,#5928,.F.);
#7662=ORIENTED_EDGE('',*,*,#5926,.F.);
#7663=ORIENTED_EDGE('',*,*,#5929,.F.);
#7664=ORIENTED_EDGE('',*,*,#5930,.F.);
#7665=ORIENTED_EDGE('',*,*,#5931,.F.);
#7666=ORIENTED_EDGE('',*,*,#5932,.F.);
#7667=ORIENTED_EDGE('',*,*,#5933,.T.);
#7668=ORIENTED_EDGE('',*,*,#5932,.T.);
#7669=ORIENTED_EDGE('',*,*,#5934,.T.);
#7670=ORIENTED_EDGE('',*,*,#5935,.F.);
#7671=ORIENTED_EDGE('',*,*,#5936,.F.);
#7672=ORIENTED_EDGE('',*,*,#5937,.F.);
#7673=ORIENTED_EDGE('',*,*,#5938,.T.);
#7674=ORIENTED_EDGE('',*,*,#5939,.T.);
#7675=ORIENTED_EDGE('',*,*,#5940,.F.);
#7676=ORIENTED_EDGE('',*,*,#5835,.T.);
#7677=ORIENTED_EDGE('',*,*,#5836,.T.);
#7678=ORIENTED_EDGE('',*,*,#5941,.T.);
#7679=ORIENTED_EDGE('',*,*,#5942,.F.);
#7680=ORIENTED_EDGE('',*,*,#5943,.T.);
#7681=ORIENTED_EDGE('',*,*,#5944,.F.);
#7682=ORIENTED_EDGE('',*,*,#5943,.F.);
#7683=ORIENTED_EDGE('',*,*,#5945,.T.);
#7684=ORIENTED_EDGE('',*,*,#5946,.T.);
#7685=ORIENTED_EDGE('',*,*,#5947,.T.);
#7686=ORIENTED_EDGE('',*,*,#5937,.T.);
#7687=ORIENTED_EDGE('',*,*,#5948,.T.);
#7688=ORIENTED_EDGE('',*,*,#5949,.T.);
#7689=ORIENTED_EDGE('',*,*,#5950,.T.);
#7690=ORIENTED_EDGE('',*,*,#5941,.F.);
#7691=ORIENTED_EDGE('',*,*,#5951,.T.);
#7692=ORIENTED_EDGE('',*,*,#5952,.T.);
#7693=ORIENTED_EDGE('',*,*,#5953,.T.);
#7694=ORIENTED_EDGE('',*,*,#5954,.T.);
#7695=ORIENTED_EDGE('',*,*,#5955,.T.);
#7696=ORIENTED_EDGE('',*,*,#5851,.T.);
#7697=ORIENTED_EDGE('',*,*,#5956,.F.);
#7698=ORIENTED_EDGE('',*,*,#5957,.T.);
#7699=ORIENTED_EDGE('',*,*,#5958,.T.);
#7700=ORIENTED_EDGE('',*,*,#5959,.T.);
#7701=ORIENTED_EDGE('',*,*,#5960,.T.);
#7702=ORIENTED_EDGE('',*,*,#5961,.T.);
#7703=ORIENTED_EDGE('',*,*,#5962,.F.);
#7704=ORIENTED_EDGE('',*,*,#5847,.T.);
#7705=ORIENTED_EDGE('',*,*,#5963,.T.);
#7706=ORIENTED_EDGE('',*,*,#5964,.T.);
#7707=ORIENTED_EDGE('',*,*,#5965,.T.);
#7708=ORIENTED_EDGE('',*,*,#5966,.T.);
#7709=ORIENTED_EDGE('',*,*,#5967,.T.);
#7710=ORIENTED_EDGE('',*,*,#5842,.T.);
#7711=ORIENTED_EDGE('',*,*,#5968,.T.);
#7712=ORIENTED_EDGE('',*,*,#5969,.T.);
#7713=ORIENTED_EDGE('',*,*,#5970,.T.);
#7714=ORIENTED_EDGE('',*,*,#5971,.T.);
#7715=ORIENTED_EDGE('',*,*,#5972,.T.);
#7716=ORIENTED_EDGE('',*,*,#5973,.T.);
#7717=ORIENTED_EDGE('',*,*,#5974,.T.);
#7718=ORIENTED_EDGE('',*,*,#5975,.T.);
#7719=ORIENTED_EDGE('',*,*,#5976,.T.);
#7720=ORIENTED_EDGE('',*,*,#5977,.T.);
#7721=ORIENTED_EDGE('',*,*,#5978,.T.);
#7722=ORIENTED_EDGE('',*,*,#5979,.T.);
#7723=ORIENTED_EDGE('',*,*,#5980,.F.);
#7724=ORIENTED_EDGE('',*,*,#5981,.T.);
#7725=ORIENTED_EDGE('',*,*,#5982,.T.);
#7726=ORIENTED_EDGE('',*,*,#5983,.T.);
#7727=ORIENTED_EDGE('',*,*,#5984,.T.);
#7728=ORIENTED_EDGE('',*,*,#5985,.T.);
#7729=ORIENTED_EDGE('',*,*,#5986,.F.);
#7730=ORIENTED_EDGE('',*,*,#5987,.T.);
#7731=ORIENTED_EDGE('',*,*,#5988,.T.);
#7732=ORIENTED_EDGE('',*,*,#5989,.T.);
#7733=ORIENTED_EDGE('',*,*,#5990,.T.);
#7734=ORIENTED_EDGE('',*,*,#5991,.T.);
#7735=ORIENTED_EDGE('',*,*,#5992,.T.);
#7736=ORIENTED_EDGE('',*,*,#5993,.T.);
#7737=ORIENTED_EDGE('',*,*,#5913,.F.);
#7738=ORIENTED_EDGE('',*,*,#5916,.F.);
#7739=ORIENTED_EDGE('',*,*,#5994,.T.);
#7740=ORIENTED_EDGE('',*,*,#5995,.T.);
#7741=ORIENTED_EDGE('',*,*,#5996,.T.);
#7742=ORIENTED_EDGE('',*,*,#5997,.T.);
#7743=ORIENTED_EDGE('',*,*,#5998,.T.);
#7744=ORIENTED_EDGE('',*,*,#5999,.T.);
#7745=ORIENTED_EDGE('',*,*,#6000,.F.);
#7746=ORIENTED_EDGE('',*,*,#6001,.T.);
#7747=ORIENTED_EDGE('',*,*,#6002,.F.);
#7748=ORIENTED_EDGE('',*,*,#6003,.T.);
#7749=ORIENTED_EDGE('',*,*,#6004,.T.);
#7750=ORIENTED_EDGE('',*,*,#6005,.T.);
#7751=ORIENTED_EDGE('',*,*,#6006,.F.);
#7752=ORIENTED_EDGE('',*,*,#6007,.T.);
#7753=ORIENTED_EDGE('',*,*,#6008,.F.);
#7754=ORIENTED_EDGE('',*,*,#6009,.T.);
#7755=ORIENTED_EDGE('',*,*,#6010,.T.);
#7756=ORIENTED_EDGE('',*,*,#6011,.T.);
#7757=ORIENTED_EDGE('',*,*,#5911,.T.);
#7758=ORIENTED_EDGE('',*,*,#5914,.T.);
#7759=ORIENTED_EDGE('',*,*,#6012,.T.);
#7760=ORIENTED_EDGE('',*,*,#5845,.T.);
#7761=ORIENTED_EDGE('',*,*,#6013,.T.);
#7762=ORIENTED_EDGE('',*,*,#6014,.T.);
#7763=ORIENTED_EDGE('',*,*,#6015,.T.);
#7764=ORIENTED_EDGE('',*,*,#6016,.T.);
#7765=ORIENTED_EDGE('',*,*,#6017,.T.);
#7766=ORIENTED_EDGE('',*,*,#5849,.T.);
#7767=ORIENTED_EDGE('',*,*,#6018,.T.);
#7768=ORIENTED_EDGE('',*,*,#6019,.F.);
#7769=ORIENTED_EDGE('',*,*,#6020,.T.);
#7770=ORIENTED_EDGE('',*,*,#6021,.F.);
#7771=ORIENTED_EDGE('',*,*,#6022,.T.);
#7772=ORIENTED_EDGE('',*,*,#5840,.T.);
#7773=ORIENTED_EDGE('',*,*,#6023,.T.);
#7774=ORIENTED_EDGE('',*,*,#6024,.F.);
#7775=ORIENTED_EDGE('',*,*,#6025,.T.);
#7776=ORIENTED_EDGE('',*,*,#6026,.F.);
#7777=ORIENTED_EDGE('',*,*,#5917,.F.);
#7778=ORIENTED_EDGE('',*,*,#5920,.F.);
#7779=ORIENTED_EDGE('',*,*,#5838,.T.);
#7780=ORIENTED_EDGE('',*,*,#5905,.T.);
#7781=ORIENTED_EDGE('',*,*,#6027,.T.);
#7782=ORIENTED_EDGE('',*,*,#5940,.T.);
#7783=ORIENTED_EDGE('',*,*,#6028,.T.);
#7784=ORIENTED_EDGE('',*,*,#6029,.T.);
#7785=ORIENTED_EDGE('',*,*,#6030,.T.);
#7786=ORIENTED_EDGE('',*,*,#6031,.T.);
#7787=ORIENTED_EDGE('',*,*,#6032,.T.);
#7788=ORIENTED_EDGE('',*,*,#6033,.T.);
#7789=ORIENTED_EDGE('',*,*,#6034,.T.);
#7790=ORIENTED_EDGE('',*,*,#5942,.T.);
#7791=ORIENTED_EDGE('',*,*,#6035,.T.);
#7792=ORIENTED_EDGE('',*,*,#6036,.T.);
#7793=ORIENTED_EDGE('',*,*,#6037,.F.);
#7794=ORIENTED_EDGE('',*,*,#6038,.T.);
#7795=ORIENTED_EDGE('',*,*,#6039,.T.);
#7796=ORIENTED_EDGE('',*,*,#6040,.T.);
#7797=ORIENTED_EDGE('',*,*,#6041,.T.);
#7798=ORIENTED_EDGE('',*,*,#6042,.T.);
#7799=ORIENTED_EDGE('',*,*,#6043,.T.);
#7800=ORIENTED_EDGE('',*,*,#6044,.T.);
#7801=ORIENTED_EDGE('',*,*,#6045,.T.);
#7802=ORIENTED_EDGE('',*,*,#6046,.T.);
#7803=ORIENTED_EDGE('',*,*,#6047,.T.);
#7804=ORIENTED_EDGE('',*,*,#6048,.T.);
#7805=ORIENTED_EDGE('',*,*,#6049,.T.);
#7806=ORIENTED_EDGE('',*,*,#6050,.T.);
#7807=ORIENTED_EDGE('',*,*,#6051,.T.);
#7808=ORIENTED_EDGE('',*,*,#6052,.T.);
#7809=ORIENTED_EDGE('',*,*,#6053,.F.);
#7810=ORIENTED_EDGE('',*,*,#6054,.F.);
#7811=ORIENTED_EDGE('',*,*,#6055,.F.);
#7812=ORIENTED_EDGE('',*,*,#6056,.F.);
#7813=ORIENTED_EDGE('',*,*,#6057,.F.);
#7814=ORIENTED_EDGE('',*,*,#6058,.F.);
#7815=ORIENTED_EDGE('',*,*,#6059,.F.);
#7816=ORIENTED_EDGE('',*,*,#6060,.F.);
#7817=ORIENTED_EDGE('',*,*,#6037,.T.);
#7818=ORIENTED_EDGE('',*,*,#6061,.T.);
#7819=ORIENTED_EDGE('',*,*,#6062,.T.);
#7820=ORIENTED_EDGE('',*,*,#6051,.F.);
#7821=ORIENTED_EDGE('',*,*,#6063,.T.);
#7822=ORIENTED_EDGE('',*,*,#6064,.T.);
#7823=ORIENTED_EDGE('',*,*,#6065,.T.);
#7824=ORIENTED_EDGE('',*,*,#6066,.T.);
#7825=ORIENTED_EDGE('',*,*,#6067,.T.);
#7826=ORIENTED_EDGE('',*,*,#6068,.T.);
#7827=ORIENTED_EDGE('',*,*,#6049,.F.);
#7828=ORIENTED_EDGE('',*,*,#6069,.T.);
#7829=ORIENTED_EDGE('',*,*,#6070,.T.);
#7830=ORIENTED_EDGE('',*,*,#6071,.T.);
#7831=ORIENTED_EDGE('',*,*,#6045,.F.);
#7832=ORIENTED_EDGE('',*,*,#6072,.T.);
#7833=ORIENTED_EDGE('',*,*,#6047,.F.);
#7834=ORIENTED_EDGE('',*,*,#6073,.T.);
#7835=ORIENTED_EDGE('',*,*,#6074,.T.);
#7836=ORIENTED_EDGE('',*,*,#6075,.T.);
#7837=ORIENTED_EDGE('',*,*,#6067,.F.);
#7838=ORIENTED_EDGE('',*,*,#6076,.T.);
#7839=ORIENTED_EDGE('',*,*,#6033,.F.);
#7840=ORIENTED_EDGE('',*,*,#6077,.T.);
#7841=ORIENTED_EDGE('',*,*,#6078,.T.);
#7842=ORIENTED_EDGE('',*,*,#6079,.T.);
#7843=ORIENTED_EDGE('',*,*,#6080,.T.);
#7844=ORIENTED_EDGE('',*,*,#6029,.F.);
#7845=ORIENTED_EDGE('',*,*,#6081,.T.);
#7846=ORIENTED_EDGE('',*,*,#6082,.T.);
#7847=ORIENTED_EDGE('',*,*,#6083,.T.);
#7848=ORIENTED_EDGE('',*,*,#6074,.F.);
#7849=ORIENTED_EDGE('',*,*,#6084,.T.);
#7850=ORIENTED_EDGE('',*,*,#6044,.F.);
#7851=ORIENTED_EDGE('',*,*,#6085,.T.);
#7852=ORIENTED_EDGE('',*,*,#6069,.F.);
#7853=ORIENTED_EDGE('',*,*,#6086,.T.);
#7854=ORIENTED_EDGE('',*,*,#6087,.T.);
#7855=ORIENTED_EDGE('',*,*,#6046,.F.);
#7856=ORIENTED_EDGE('',*,*,#6071,.F.);
#7857=ORIENTED_EDGE('',*,*,#6088,.F.);
#7858=ORIENTED_EDGE('',*,*,#6073,.F.);
#7859=ORIENTED_EDGE('',*,*,#6088,.T.);
#7860=ORIENTED_EDGE('',*,*,#6070,.F.);
#7861=ORIENTED_EDGE('',*,*,#6089,.F.);
#7862=ORIENTED_EDGE('',*,*,#6084,.F.);
#7863=ORIENTED_EDGE('',*,*,#6089,.T.);
#7864=ORIENTED_EDGE('',*,*,#6085,.F.);
#7865=ORIENTED_EDGE('',*,*,#6090,.F.);
#7866=ORIENTED_EDGE('',*,*,#6079,.F.);
#7867=ORIENTED_EDGE('',*,*,#6090,.T.);
#7868=ORIENTED_EDGE('',*,*,#6043,.F.);
#7869=ORIENTED_EDGE('',*,*,#6091,.F.);
#7870=ORIENTED_EDGE('',*,*,#6080,.F.);
#7871=ORIENTED_EDGE('',*,*,#6042,.F.);
#7872=ORIENTED_EDGE('',*,*,#6092,.T.);
#7873=ORIENTED_EDGE('',*,*,#6027,.F.);
#7874=ORIENTED_EDGE('',*,*,#6091,.T.);
#7875=ORIENTED_EDGE('',*,*,#6048,.F.);
#7876=ORIENTED_EDGE('',*,*,#6075,.F.);
#7877=ORIENTED_EDGE('',*,*,#6093,.F.);
#7878=ORIENTED_EDGE('',*,*,#6065,.F.);
#7879=ORIENTED_EDGE('',*,*,#6093,.T.);
#7880=ORIENTED_EDGE('',*,*,#6083,.F.);
#7881=ORIENTED_EDGE('',*,*,#6094,.F.);
#7882=ORIENTED_EDGE('',*,*,#6066,.F.);
#7883=ORIENTED_EDGE('',*,*,#6094,.T.);
#7884=ORIENTED_EDGE('',*,*,#6082,.F.);
#7885=ORIENTED_EDGE('',*,*,#6095,.F.);
#7886=ORIENTED_EDGE('',*,*,#6076,.F.);
#7887=ORIENTED_EDGE('',*,*,#6095,.T.);
#7888=ORIENTED_EDGE('',*,*,#6081,.F.);
#7889=ORIENTED_EDGE('',*,*,#6096,.F.);
#7890=ORIENTED_EDGE('',*,*,#6034,.F.);
#7891=ORIENTED_EDGE('',*,*,#6028,.F.);
#7892=ORIENTED_EDGE('',*,*,#6097,.T.);
#7893=ORIENTED_EDGE('',*,*,#6030,.F.);
#7894=ORIENTED_EDGE('',*,*,#6096,.T.);
#7895=ORIENTED_EDGE('',*,*,#6052,.F.);
#7896=ORIENTED_EDGE('',*,*,#6062,.F.);
#7897=ORIENTED_EDGE('',*,*,#6098,.F.);
#7898=ORIENTED_EDGE('',*,*,#6072,.F.);
#7899=ORIENTED_EDGE('',*,*,#6098,.T.);
#7900=ORIENTED_EDGE('',*,*,#6061,.F.);
#7901=ORIENTED_EDGE('',*,*,#6099,.F.);
#7902=ORIENTED_EDGE('',*,*,#6086,.F.);
#7903=ORIENTED_EDGE('',*,*,#6099,.T.);
#7904=ORIENTED_EDGE('',*,*,#6036,.F.);
#7905=ORIENTED_EDGE('',*,*,#6100,.F.);
#7906=ORIENTED_EDGE('',*,*,#6087,.F.);
#7907=ORIENTED_EDGE('',*,*,#6035,.F.);
#7908=ORIENTED_EDGE('',*,*,#6101,.T.);
#7909=ORIENTED_EDGE('',*,*,#6040,.F.);
#7910=ORIENTED_EDGE('',*,*,#6100,.T.);
#7911=ORIENTED_EDGE('',*,*,#6050,.F.);
#7912=ORIENTED_EDGE('',*,*,#6068,.F.);
#7913=ORIENTED_EDGE('',*,*,#6102,.F.);
#7914=ORIENTED_EDGE('',*,*,#6063,.F.);
#7915=ORIENTED_EDGE('',*,*,#6102,.T.);
#7916=ORIENTED_EDGE('',*,*,#6078,.F.);
#7917=ORIENTED_EDGE('',*,*,#6103,.F.);
#7918=ORIENTED_EDGE('',*,*,#6064,.F.);
#7919=ORIENTED_EDGE('',*,*,#6103,.T.);
#7920=ORIENTED_EDGE('',*,*,#6077,.F.);
#7921=ORIENTED_EDGE('',*,*,#6104,.F.);
#7922=ORIENTED_EDGE('',*,*,#6038,.F.);
#7923=ORIENTED_EDGE('',*,*,#6032,.F.);
#7924=ORIENTED_EDGE('',*,*,#6105,.T.);
#7925=ORIENTED_EDGE('',*,*,#6039,.F.);
#7926=ORIENTED_EDGE('',*,*,#6104,.T.);
#7927=ORIENTED_EDGE('',*,*,#5945,.F.);
#7928=ORIENTED_EDGE('',*,*,#6105,.F.);
#7929=ORIENTED_EDGE('',*,*,#6106,.F.);
#7930=ORIENTED_EDGE('',*,*,#6106,.T.);
#7931=ORIENTED_EDGE('',*,*,#6031,.F.);
#7932=ORIENTED_EDGE('',*,*,#6107,.F.);
#7933=ORIENTED_EDGE('',*,*,#5946,.F.);
#7934=ORIENTED_EDGE('',*,*,#6107,.T.);
#7935=ORIENTED_EDGE('',*,*,#6097,.F.);
#7936=ORIENTED_EDGE('',*,*,#5939,.F.);
#7937=ORIENTED_EDGE('',*,*,#5938,.F.);
#7938=ORIENTED_EDGE('',*,*,#5947,.F.);
#7939=ORIENTED_EDGE('',*,*,#5936,.T.);
#7940=ORIENTED_EDGE('',*,*,#5935,.T.);
#7941=ORIENTED_EDGE('',*,*,#6092,.F.);
#7942=ORIENTED_EDGE('',*,*,#6108,.F.);
#7943=ORIENTED_EDGE('',*,*,#5948,.F.);
#7944=ORIENTED_EDGE('',*,*,#6108,.T.);
#7945=ORIENTED_EDGE('',*,*,#6041,.F.);
#7946=ORIENTED_EDGE('',*,*,#6109,.F.);
#7947=ORIENTED_EDGE('',*,*,#5949,.F.);
#7948=ORIENTED_EDGE('',*,*,#6109,.T.);
#7949=ORIENTED_EDGE('',*,*,#6101,.F.);
#7950=ORIENTED_EDGE('',*,*,#5950,.F.);
#7951=ORIENTED_EDGE('',*,*,#5927,.T.);
#7952=ORIENTED_EDGE('',*,*,#5834,.T.);
#7953=ORIENTED_EDGE('',*,*,#6110,.F.);
#7954=ORIENTED_EDGE('',*,*,#5909,.T.);
#7955=ORIENTED_EDGE('',*,*,#6111,.F.);
#7956=ORIENTED_EDGE('',*,*,#6112,.F.);
#7957=ORIENTED_EDGE('',*,*,#6113,.F.);
#7958=ORIENTED_EDGE('',*,*,#5924,.F.);
#7959=ORIENTED_EDGE('',*,*,#6114,.F.);
#7960=ORIENTED_EDGE('',*,*,#6115,.F.);
#7961=ORIENTED_EDGE('',*,*,#6116,.F.);
#7962=ORIENTED_EDGE('',*,*,#6117,.F.);
#7963=ORIENTED_EDGE('',*,*,#6118,.F.);
#7964=ORIENTED_EDGE('',*,*,#5934,.F.);
#7965=ORIENTED_EDGE('',*,*,#6119,.F.);
#7966=ORIENTED_EDGE('',*,*,#6120,.F.);
#7967=ORIENTED_EDGE('',*,*,#6121,.T.);
#7968=ORIENTED_EDGE('',*,*,#6122,.F.);
#7969=ORIENTED_EDGE('',*,*,#6123,.F.);
#7970=ORIENTED_EDGE('',*,*,#6124,.F.);
#7971=ORIENTED_EDGE('',*,*,#6125,.F.);
#7972=ORIENTED_EDGE('',*,*,#6126,.F.);
#7973=ORIENTED_EDGE('',*,*,#6127,.F.);
#7974=ORIENTED_EDGE('',*,*,#6128,.F.);
#7975=ORIENTED_EDGE('',*,*,#6121,.F.);
#7976=ORIENTED_EDGE('',*,*,#6129,.F.);
#7977=ORIENTED_EDGE('',*,*,#6130,.F.);
#7978=ORIENTED_EDGE('',*,*,#6055,.T.);
#7979=ORIENTED_EDGE('',*,*,#6131,.F.);
#7980=ORIENTED_EDGE('',*,*,#6132,.F.);
#7981=ORIENTED_EDGE('',*,*,#6133,.F.);
#7982=ORIENTED_EDGE('',*,*,#6057,.T.);
#7983=ORIENTED_EDGE('',*,*,#6134,.F.);
#7984=ORIENTED_EDGE('',*,*,#6135,.F.);
#7985=ORIENTED_EDGE('',*,*,#6136,.F.);
#7986=ORIENTED_EDGE('',*,*,#6137,.F.);
#7987=ORIENTED_EDGE('',*,*,#6138,.F.);
#7988=ORIENTED_EDGE('',*,*,#6053,.T.);
#7989=ORIENTED_EDGE('',*,*,#6139,.F.);
#7990=ORIENTED_EDGE('',*,*,#6140,.F.);
#7991=ORIENTED_EDGE('',*,*,#6059,.T.);
#7992=ORIENTED_EDGE('',*,*,#6141,.F.);
#7993=ORIENTED_EDGE('',*,*,#6142,.F.);
#7994=ORIENTED_EDGE('',*,*,#6143,.F.);
#7995=ORIENTED_EDGE('',*,*,#6135,.T.);
#7996=ORIENTED_EDGE('',*,*,#6144,.F.);
#7997=ORIENTED_EDGE('',*,*,#6145,.F.);
#7998=ORIENTED_EDGE('',*,*,#6116,.T.);
#7999=ORIENTED_EDGE('',*,*,#6146,.F.);
#8000=ORIENTED_EDGE('',*,*,#6147,.F.);
#8001=ORIENTED_EDGE('',*,*,#6148,.F.);
#8002=ORIENTED_EDGE('',*,*,#6142,.T.);
#8003=ORIENTED_EDGE('',*,*,#6149,.F.);
#8004=ORIENTED_EDGE('',*,*,#6150,.F.);
#8005=ORIENTED_EDGE('',*,*,#6151,.F.);
#8006=ORIENTED_EDGE('',*,*,#6112,.T.);
#8007=ORIENTED_EDGE('',*,*,#6152,.F.);
#8008=ORIENTED_EDGE('',*,*,#6125,.T.);
#8009=ORIENTED_EDGE('',*,*,#6153,.F.);
#8010=ORIENTED_EDGE('',*,*,#6154,.F.);
#8011=ORIENTED_EDGE('',*,*,#6137,.T.);
#8012=ORIENTED_EDGE('',*,*,#6155,.F.);
#8013=ORIENTED_EDGE('',*,*,#6060,.T.);
#8014=ORIENTED_EDGE('',*,*,#6143,.T.);
#8015=ORIENTED_EDGE('',*,*,#6156,.T.);
#8016=ORIENTED_EDGE('',*,*,#6139,.T.);
#8017=ORIENTED_EDGE('',*,*,#6156,.F.);
#8018=ORIENTED_EDGE('',*,*,#6148,.T.);
#8019=ORIENTED_EDGE('',*,*,#6157,.T.);
#8020=ORIENTED_EDGE('',*,*,#6140,.T.);
#8021=ORIENTED_EDGE('',*,*,#6157,.F.);
#8022=ORIENTED_EDGE('',*,*,#6147,.T.);
#8023=ORIENTED_EDGE('',*,*,#6158,.T.);
#8024=ORIENTED_EDGE('',*,*,#6155,.T.);
#8025=ORIENTED_EDGE('',*,*,#6158,.F.);
#8026=ORIENTED_EDGE('',*,*,#6152,.T.);
#8027=ORIENTED_EDGE('',*,*,#6159,.T.);
#8028=ORIENTED_EDGE('',*,*,#6126,.T.);
#8029=ORIENTED_EDGE('',*,*,#6127,.T.);
#8030=ORIENTED_EDGE('',*,*,#6159,.F.);
#8031=ORIENTED_EDGE('',*,*,#6111,.T.);
#8032=ORIENTED_EDGE('',*,*,#6160,.F.);
#8033=ORIENTED_EDGE('',*,*,#6058,.T.);
#8034=ORIENTED_EDGE('',*,*,#6133,.T.);
#8035=ORIENTED_EDGE('',*,*,#6161,.T.);
#8036=ORIENTED_EDGE('',*,*,#6141,.T.);
#8037=ORIENTED_EDGE('',*,*,#6161,.F.);
#8038=ORIENTED_EDGE('',*,*,#6136,.T.);
#8039=ORIENTED_EDGE('',*,*,#6162,.T.);
#8040=ORIENTED_EDGE('',*,*,#6149,.T.);
#8041=ORIENTED_EDGE('',*,*,#6162,.F.);
#8042=ORIENTED_EDGE('',*,*,#6146,.T.);
#8043=ORIENTED_EDGE('',*,*,#6163,.T.);
#8044=ORIENTED_EDGE('',*,*,#6150,.T.);
#8045=ORIENTED_EDGE('',*,*,#6163,.F.);
#8046=ORIENTED_EDGE('',*,*,#6115,.T.);
#8047=ORIENTED_EDGE('',*,*,#6164,.T.);
#8048=ORIENTED_EDGE('',*,*,#6151,.T.);
#8049=ORIENTED_EDGE('',*,*,#6113,.T.);
#8050=ORIENTED_EDGE('',*,*,#6164,.F.);
#8051=ORIENTED_EDGE('',*,*,#6114,.T.);
#8052=ORIENTED_EDGE('',*,*,#6165,.F.);
#8053=ORIENTED_EDGE('',*,*,#6054,.T.);
#8054=ORIENTED_EDGE('',*,*,#6138,.T.);
#8055=ORIENTED_EDGE('',*,*,#6166,.T.);
#8056=ORIENTED_EDGE('',*,*,#6131,.T.);
#8057=ORIENTED_EDGE('',*,*,#6166,.F.);
#8058=ORIENTED_EDGE('',*,*,#6154,.T.);
#8059=ORIENTED_EDGE('',*,*,#6167,.T.);
#8060=ORIENTED_EDGE('',*,*,#6132,.T.);
#8061=ORIENTED_EDGE('',*,*,#6167,.F.);
#8062=ORIENTED_EDGE('',*,*,#6153,.T.);
#8063=ORIENTED_EDGE('',*,*,#6168,.T.);
#8064=ORIENTED_EDGE('',*,*,#6122,.T.);
#8065=ORIENTED_EDGE('',*,*,#6123,.T.);
#8066=ORIENTED_EDGE('',*,*,#6168,.F.);
#8067=ORIENTED_EDGE('',*,*,#6124,.T.);
#8068=ORIENTED_EDGE('',*,*,#6169,.F.);
#8069=ORIENTED_EDGE('',*,*,#6056,.T.);
#8070=ORIENTED_EDGE('',*,*,#6130,.T.);
#8071=ORIENTED_EDGE('',*,*,#6170,.T.);
#8072=ORIENTED_EDGE('',*,*,#6134,.T.);
#8073=ORIENTED_EDGE('',*,*,#6170,.F.);
#8074=ORIENTED_EDGE('',*,*,#6129,.T.);
#8075=ORIENTED_EDGE('',*,*,#6171,.T.);
#8076=ORIENTED_EDGE('',*,*,#6144,.T.);
#8077=ORIENTED_EDGE('',*,*,#6171,.F.);
#8078=ORIENTED_EDGE('',*,*,#6120,.T.);
#8079=ORIENTED_EDGE('',*,*,#6172,.T.);
#8080=ORIENTED_EDGE('',*,*,#6145,.T.);
#8081=ORIENTED_EDGE('',*,*,#6117,.T.);
#8082=ORIENTED_EDGE('',*,*,#6172,.F.);
#8083=ORIENTED_EDGE('',*,*,#6119,.T.);
#8084=ORIENTED_EDGE('',*,*,#6173,.F.);
#8085=ORIENTED_EDGE('',*,*,#5931,.T.);
#8086=ORIENTED_EDGE('',*,*,#6174,.T.);
#8087=ORIENTED_EDGE('',*,*,#6173,.T.);
#8088=ORIENTED_EDGE('',*,*,#6174,.F.);
#8089=ORIENTED_EDGE('',*,*,#5930,.T.);
#8090=ORIENTED_EDGE('',*,*,#6175,.T.);
#8091=ORIENTED_EDGE('',*,*,#6118,.T.);
#8092=ORIENTED_EDGE('',*,*,#6175,.F.);
#8093=ORIENTED_EDGE('',*,*,#5929,.T.);
#8094=ORIENTED_EDGE('',*,*,#5925,.T.);
#8095=ORIENTED_EDGE('',*,*,#6165,.T.);
#8096=ORIENTED_EDGE('',*,*,#5923,.F.);
#8097=ORIENTED_EDGE('',*,*,#5928,.T.);
#8098=ORIENTED_EDGE('',*,*,#6176,.T.);
#8099=ORIENTED_EDGE('',*,*,#6160,.T.);
#8100=ORIENTED_EDGE('',*,*,#6176,.F.);
#8101=ORIENTED_EDGE('',*,*,#6110,.T.);
#8102=ORIENTED_EDGE('',*,*,#6177,.T.);
#8103=ORIENTED_EDGE('',*,*,#6128,.T.);
#8104=ORIENTED_EDGE('',*,*,#6177,.F.);
#8105=ORIENTED_EDGE('',*,*,#5833,.T.);
#8106=ORIENTED_EDGE('',*,*,#6169,.T.);
#8107=ORIENTED_EDGE('',*,*,#6178,.T.);
#8108=ORIENTED_EDGE('',*,*,#6179,.T.);
#8109=ORIENTED_EDGE('',*,*,#6180,.T.);
#8110=ORIENTED_EDGE('',*,*,#6181,.T.);
#8111=ORIENTED_EDGE('',*,*,#6182,.T.);
#8112=ORIENTED_EDGE('',*,*,#6183,.T.);
#8113=ORIENTED_EDGE('',*,*,#6184,.T.);
#8114=ORIENTED_EDGE('',*,*,#6185,.T.);
#8115=ORIENTED_EDGE('',*,*,#6186,.T.);
#8116=ORIENTED_EDGE('',*,*,#6187,.T.);
#8117=ORIENTED_EDGE('',*,*,#5919,.F.);
#8118=ORIENTED_EDGE('',*,*,#5922,.F.);
#8119=ORIENTED_EDGE('',*,*,#6188,.T.);
#8120=ORIENTED_EDGE('',*,*,#6189,.T.);
#8121=ORIENTED_EDGE('',*,*,#6190,.T.);
#8122=ORIENTED_EDGE('',*,*,#6191,.T.);
#8123=ORIENTED_EDGE('',*,*,#6192,.T.);
#8124=ORIENTED_EDGE('',*,*,#6193,.T.);
#8125=ORIENTED_EDGE('',*,*,#6194,.T.);
#8126=ORIENTED_EDGE('',*,*,#6195,.T.);
#8127=ORIENTED_EDGE('',*,*,#6196,.T.);
#8128=ORIENTED_EDGE('',*,*,#6197,.T.);
#8129=ORIENTED_EDGE('',*,*,#6198,.T.);
#8130=ORIENTED_EDGE('',*,*,#6199,.T.);
#8131=ORIENTED_EDGE('',*,*,#6200,.T.);
#8132=ORIENTED_EDGE('',*,*,#6201,.T.);
#8133=ORIENTED_EDGE('',*,*,#6202,.T.);
#8134=ORIENTED_EDGE('',*,*,#6203,.T.);
#8135=ORIENTED_EDGE('',*,*,#6204,.T.);
#8136=ORIENTED_EDGE('',*,*,#6205,.T.);
#8137=ORIENTED_EDGE('',*,*,#6206,.T.);
#8138=ORIENTED_EDGE('',*,*,#6207,.T.);
#8139=ORIENTED_EDGE('',*,*,#6208,.T.);
#8140=ORIENTED_EDGE('',*,*,#6209,.T.);
#8141=ORIENTED_EDGE('',*,*,#6210,.T.);
#8142=ORIENTED_EDGE('',*,*,#6211,.T.);
#8143=ORIENTED_EDGE('',*,*,#6212,.T.);
#8144=ORIENTED_EDGE('',*,*,#6213,.T.);
#8145=ORIENTED_EDGE('',*,*,#6214,.T.);
#8146=ORIENTED_EDGE('',*,*,#6215,.T.);
#8147=ORIENTED_EDGE('',*,*,#6216,.T.);
#8148=ORIENTED_EDGE('',*,*,#6217,.T.);
#8149=ORIENTED_EDGE('',*,*,#6218,.T.);
#8150=ORIENTED_EDGE('',*,*,#6219,.T.);
#8151=ORIENTED_EDGE('',*,*,#6220,.T.);
#8152=ORIENTED_EDGE('',*,*,#6221,.T.);
#8153=ORIENTED_EDGE('',*,*,#6222,.T.);
#8154=ORIENTED_EDGE('',*,*,#6223,.T.);
#8155=ORIENTED_EDGE('',*,*,#6224,.T.);
#8156=ORIENTED_EDGE('',*,*,#6225,.T.);
#8157=ORIENTED_EDGE('',*,*,#6226,.T.);
#8158=ORIENTED_EDGE('',*,*,#6227,.T.);
#8159=ORIENTED_EDGE('',*,*,#6228,.T.);
#8160=ORIENTED_EDGE('',*,*,#6229,.T.);
#8161=ORIENTED_EDGE('',*,*,#6230,.T.);
#8162=ORIENTED_EDGE('',*,*,#6231,.T.);
#8163=ORIENTED_EDGE('',*,*,#6232,.T.);
#8164=ORIENTED_EDGE('',*,*,#6233,.T.);
#8165=ORIENTED_EDGE('',*,*,#6234,.T.);
#8166=ORIENTED_EDGE('',*,*,#6235,.T.);
#8167=ORIENTED_EDGE('',*,*,#6236,.T.);
#8168=ORIENTED_EDGE('',*,*,#6237,.T.);
#8169=ORIENTED_EDGE('',*,*,#6238,.T.);
#8170=ORIENTED_EDGE('',*,*,#6239,.T.);
#8171=ORIENTED_EDGE('',*,*,#6240,.T.);
#8172=ORIENTED_EDGE('',*,*,#6241,.T.);
#8173=ORIENTED_EDGE('',*,*,#6242,.T.);
#8174=ORIENTED_EDGE('',*,*,#6243,.T.);
#8175=ORIENTED_EDGE('',*,*,#6244,.T.);
#8176=ORIENTED_EDGE('',*,*,#6245,.T.);
#8177=ORIENTED_EDGE('',*,*,#6246,.T.);
#8178=ORIENTED_EDGE('',*,*,#6247,.T.);
#8179=ORIENTED_EDGE('',*,*,#6248,.T.);
#8180=ORIENTED_EDGE('',*,*,#6249,.T.);
#8181=ORIENTED_EDGE('',*,*,#6250,.T.);
#8182=ORIENTED_EDGE('',*,*,#6251,.T.);
#8183=ORIENTED_EDGE('',*,*,#6252,.T.);
#8184=ORIENTED_EDGE('',*,*,#6253,.T.);
#8185=ORIENTED_EDGE('',*,*,#6254,.T.);
#8186=ORIENTED_EDGE('',*,*,#6255,.T.);
#8187=ORIENTED_EDGE('',*,*,#6256,.T.);
#8188=ORIENTED_EDGE('',*,*,#6257,.T.);
#8189=ORIENTED_EDGE('',*,*,#6258,.T.);
#8190=ORIENTED_EDGE('',*,*,#6259,.T.);
#8191=ORIENTED_EDGE('',*,*,#6260,.T.);
#8192=ORIENTED_EDGE('',*,*,#6261,.T.);
#8193=ORIENTED_EDGE('',*,*,#6262,.T.);
#8194=ORIENTED_EDGE('',*,*,#6263,.T.);
#8195=ORIENTED_EDGE('',*,*,#5871,.T.);
#8196=ORIENTED_EDGE('',*,*,#5944,.T.);
#8197=ORIENTED_EDGE('',*,*,#5900,.T.);
#8198=ORIENTED_EDGE('',*,*,#5895,.T.);
#8199=ORIENTED_EDGE('',*,*,#5890,.T.);
#8200=ORIENTED_EDGE('',*,*,#5885,.T.);
#8201=ORIENTED_EDGE('',*,*,#5880,.T.);
#8202=ORIENTED_EDGE('',*,*,#5875,.T.);
#8203=ORIENTED_EDGE('',*,*,#5864,.T.);
#8204=ORIENTED_EDGE('',*,*,#5874,.F.);
#8205=ORIENTED_EDGE('',*,*,#5879,.F.);
#8206=ORIENTED_EDGE('',*,*,#5884,.F.);
#8207=ORIENTED_EDGE('',*,*,#5889,.F.);
#8208=ORIENTED_EDGE('',*,*,#5894,.F.);
#8209=ORIENTED_EDGE('',*,*,#5899,.F.);
#8210=ORIENTED_EDGE('',*,*,#5933,.F.);
#8211=ORIENTED_EDGE('',*,*,#6264,.F.);
#8212=ORIENTED_EDGE('',*,*,#6234,.F.);
#8213=ORIENTED_EDGE('',*,*,#5862,.F.);
#8214=ORIENTED_EDGE('',*,*,#6009,.F.);
#8215=ORIENTED_EDGE('',*,*,#6265,.F.);
#8216=ORIENTED_EDGE('',*,*,#6232,.F.);
#8217=ORIENTED_EDGE('',*,*,#6266,.F.);
#8218=ORIENTED_EDGE('',*,*,#6231,.F.);
#8219=ORIENTED_EDGE('',*,*,#5863,.F.);
#8220=ORIENTED_EDGE('',*,*,#6233,.F.);
#8221=ORIENTED_EDGE('',*,*,#6267,.F.);
#8222=ORIENTED_EDGE('',*,*,#5968,.F.);
#8223=ORIENTED_EDGE('',*,*,#6268,.F.);
#8224=ORIENTED_EDGE('',*,*,#6269,.F.);
#8225=ORIENTED_EDGE('',*,*,#6270,.F.);
#8226=ORIENTED_EDGE('',*,*,#6271,.F.);
#8227=ORIENTED_EDGE('',*,*,#6272,.F.);
#8228=ORIENTED_EDGE('',*,*,#6273,.F.);
#8229=ORIENTED_EDGE('',*,*,#6264,.T.);
#8230=ORIENTED_EDGE('',*,*,#6008,.T.);
#8231=ORIENTED_EDGE('',*,*,#6274,.F.);
#8232=ORIENTED_EDGE('',*,*,#6266,.T.);
#8233=ORIENTED_EDGE('',*,*,#6267,.T.);
#8234=ORIENTED_EDGE('',*,*,#6265,.T.);
#8235=ORIENTED_EDGE('',*,*,#6275,.F.);
#8236=ORIENTED_EDGE('',*,*,#5969,.F.);
#8237=ORIENTED_EDGE('',*,*,#5861,.T.);
#8238=ORIENTED_EDGE('',*,*,#5987,.F.);
#8239=ORIENTED_EDGE('',*,*,#6276,.F.);
#8240=ORIENTED_EDGE('',*,*,#6010,.F.);
#8241=ORIENTED_EDGE('',*,*,#6272,.T.);
#8242=ORIENTED_EDGE('',*,*,#6011,.F.);
#8243=ORIENTED_EDGE('',*,*,#6277,.F.);
#8244=ORIENTED_EDGE('',*,*,#6224,.F.);
#8245=ORIENTED_EDGE('',*,*,#6273,.T.);
#8246=ORIENTED_EDGE('',*,*,#6227,.F.);
#8247=ORIENTED_EDGE('',*,*,#6278,.F.);
#8248=ORIENTED_EDGE('',*,*,#6253,.F.);
#8249=ORIENTED_EDGE('',*,*,#6269,.T.);
#8250=ORIENTED_EDGE('',*,*,#6254,.F.);
#8251=ORIENTED_EDGE('',*,*,#6279,.F.);
#8252=ORIENTED_EDGE('',*,*,#5993,.F.);
#8253=ORIENTED_EDGE('',*,*,#6270,.T.);
#8254=ORIENTED_EDGE('',*,*,#5992,.F.);
#8255=ORIENTED_EDGE('',*,*,#6280,.F.);
#8256=ORIENTED_EDGE('',*,*,#6218,.F.);
#8257=ORIENTED_EDGE('',*,*,#6268,.T.);
#8258=ORIENTED_EDGE('',*,*,#6217,.F.);
#8259=ORIENTED_EDGE('',*,*,#6281,.F.);
#8260=ORIENTED_EDGE('',*,*,#6255,.F.);
#8261=ORIENTED_EDGE('',*,*,#6271,.T.);
#8262=ORIENTED_EDGE('',*,*,#6252,.F.);
#8263=ORIENTED_EDGE('',*,*,#6282,.F.);
#8264=ORIENTED_EDGE('',*,*,#5994,.F.);
#8265=ORIENTED_EDGE('',*,*,#6274,.T.);
#8266=ORIENTED_EDGE('',*,*,#6007,.F.);
#8267=ORIENTED_EDGE('',*,*,#6283,.F.);
#8268=ORIENTED_EDGE('',*,*,#6228,.F.);
#8269=ORIENTED_EDGE('',*,*,#6284,.F.);
#8270=ORIENTED_EDGE('',*,*,#6229,.F.);
#8271=ORIENTED_EDGE('',*,*,#6285,.F.);
#8272=ORIENTED_EDGE('',*,*,#6237,.F.);
#8273=ORIENTED_EDGE('',*,*,#6275,.T.);
#8274=ORIENTED_EDGE('',*,*,#6230,.F.);
#8275=ORIENTED_EDGE('',*,*,#6286,.F.);
#8276=ORIENTED_EDGE('',*,*,#5970,.F.);
#8277=ORIENTED_EDGE('',*,*,#6276,.T.);
#8278=ORIENTED_EDGE('',*,*,#5986,.T.);
#8279=ORIENTED_EDGE('',*,*,#6287,.F.);
#8280=ORIENTED_EDGE('',*,*,#6277,.T.);
#8281=ORIENTED_EDGE('',*,*,#6279,.T.);
#8282=ORIENTED_EDGE('',*,*,#6278,.T.);
#8283=ORIENTED_EDGE('',*,*,#6288,.F.);
#8284=ORIENTED_EDGE('',*,*,#6289,.F.);
#8285=ORIENTED_EDGE('',*,*,#6280,.T.);
#8286=ORIENTED_EDGE('',*,*,#6290,.F.);
#8287=ORIENTED_EDGE('',*,*,#6282,.T.);
#8288=ORIENTED_EDGE('',*,*,#6281,.T.);
#8289=ORIENTED_EDGE('',*,*,#6291,.F.);
#8290=ORIENTED_EDGE('',*,*,#6283,.T.);
#8291=ORIENTED_EDGE('',*,*,#6006,.T.);
#8292=ORIENTED_EDGE('',*,*,#6292,.F.);
#8293=ORIENTED_EDGE('',*,*,#6285,.T.);
#8294=ORIENTED_EDGE('',*,*,#6286,.T.);
#8295=ORIENTED_EDGE('',*,*,#6284,.T.);
#8296=ORIENTED_EDGE('',*,*,#6293,.F.);
#8297=ORIENTED_EDGE('',*,*,#5971,.F.);
#8298=ORIENTED_EDGE('',*,*,#6287,.T.);
#8299=ORIENTED_EDGE('',*,*,#5985,.F.);
#8300=ORIENTED_EDGE('',*,*,#6294,.F.);
#8301=ORIENTED_EDGE('',*,*,#6225,.F.);
#8302=ORIENTED_EDGE('',*,*,#6288,.T.);
#8303=ORIENTED_EDGE('',*,*,#6226,.F.);
#8304=ORIENTED_EDGE('',*,*,#6295,.F.);
#8305=ORIENTED_EDGE('',*,*,#5988,.F.);
#8306=ORIENTED_EDGE('',*,*,#6290,.T.);
#8307=ORIENTED_EDGE('',*,*,#5991,.F.);
#8308=ORIENTED_EDGE('',*,*,#6296,.F.);
#8309=ORIENTED_EDGE('',*,*,#6250,.F.);
#8310=ORIENTED_EDGE('',*,*,#6289,.T.);
#8311=ORIENTED_EDGE('',*,*,#6249,.F.);
#8312=ORIENTED_EDGE('',*,*,#6297,.F.);
#8313=ORIENTED_EDGE('',*,*,#6219,.F.);
#8314=ORIENTED_EDGE('',*,*,#6291,.T.);
#8315=ORIENTED_EDGE('',*,*,#6216,.F.);
#8316=ORIENTED_EDGE('',*,*,#6298,.F.);
#8317=ORIENTED_EDGE('',*,*,#5995,.F.);
#8318=ORIENTED_EDGE('',*,*,#6292,.T.);
#8319=ORIENTED_EDGE('',*,*,#6005,.F.);
#8320=ORIENTED_EDGE('',*,*,#5859,.F.);
#8321=ORIENTED_EDGE('',*,*,#6235,.F.);
#8322=ORIENTED_EDGE('',*,*,#6293,.T.);
#8323=ORIENTED_EDGE('',*,*,#6236,.F.);
#8324=ORIENTED_EDGE('',*,*,#5858,.F.);
#8325=ORIENTED_EDGE('',*,*,#5972,.F.);
#8326=ORIENTED_EDGE('',*,*,#6294,.T.);
#8327=ORIENTED_EDGE('',*,*,#5984,.F.);
#8328=ORIENTED_EDGE('',*,*,#6299,.F.);
#8329=ORIENTED_EDGE('',*,*,#6295,.T.);
#8330=ORIENTED_EDGE('',*,*,#6300,.F.);
#8331=ORIENTED_EDGE('',*,*,#6296,.T.);
#8332=ORIENTED_EDGE('',*,*,#6301,.F.);
#8333=ORIENTED_EDGE('',*,*,#6298,.T.);
#8334=ORIENTED_EDGE('',*,*,#6297,.T.);
#8335=ORIENTED_EDGE('',*,*,#6302,.F.);
#8336=ORIENTED_EDGE('',*,*,#6299,.T.);
#8337=ORIENTED_EDGE('',*,*,#5983,.F.);
#8338=ORIENTED_EDGE('',*,*,#6303,.F.);
#8339=ORIENTED_EDGE('',*,*,#5989,.F.);
#8340=ORIENTED_EDGE('',*,*,#6301,.T.);
#8341=ORIENTED_EDGE('',*,*,#5990,.F.);
#8342=ORIENTED_EDGE('',*,*,#6304,.F.);
#8343=ORIENTED_EDGE('',*,*,#6221,.F.);
#8344=ORIENTED_EDGE('',*,*,#6300,.T.);
#8345=ORIENTED_EDGE('',*,*,#6220,.F.);
#8346=ORIENTED_EDGE('',*,*,#6305,.F.);
#8347=ORIENTED_EDGE('',*,*,#6251,.F.);
#8348=ORIENTED_EDGE('',*,*,#6302,.T.);
#8349=ORIENTED_EDGE('',*,*,#6248,.F.);
#8350=ORIENTED_EDGE('',*,*,#6306,.F.);
#8351=ORIENTED_EDGE('',*,*,#5996,.F.);
#8352=ORIENTED_EDGE('',*,*,#5856,.F.);
#8353=ORIENTED_EDGE('',*,*,#6003,.F.);
#8354=ORIENTED_EDGE('',*,*,#6307,.F.);
#8355=ORIENTED_EDGE('',*,*,#6247,.F.);
#8356=ORIENTED_EDGE('',*,*,#5860,.T.);
#8357=ORIENTED_EDGE('',*,*,#6004,.F.);
#8358=ORIENTED_EDGE('',*,*,#5855,.F.);
#8359=ORIENTED_EDGE('',*,*,#5973,.F.);
#8360=ORIENTED_EDGE('',*,*,#6303,.T.);
#8361=ORIENTED_EDGE('',*,*,#5982,.F.);
#8362=ORIENTED_EDGE('',*,*,#6308,.F.);
#8363=ORIENTED_EDGE('',*,*,#6304,.T.);
#8364=ORIENTED_EDGE('',*,*,#6306,.T.);
#8365=ORIENTED_EDGE('',*,*,#6305,.T.);
#8366=ORIENTED_EDGE('',*,*,#6309,.F.);
#8367=ORIENTED_EDGE('',*,*,#6307,.T.);
#8368=ORIENTED_EDGE('',*,*,#6002,.T.);
#8369=ORIENTED_EDGE('',*,*,#6310,.F.);
#8370=ORIENTED_EDGE('',*,*,#6311,.F.);
#8371=ORIENTED_EDGE('',*,*,#6308,.T.);
#8372=ORIENTED_EDGE('',*,*,#5981,.F.);
#8373=ORIENTED_EDGE('',*,*,#6312,.F.);
#8374=ORIENTED_EDGE('',*,*,#6222,.F.);
#8375=ORIENTED_EDGE('',*,*,#6309,.T.);
#8376=ORIENTED_EDGE('',*,*,#6223,.F.);
#8377=ORIENTED_EDGE('',*,*,#6313,.F.);
#8378=ORIENTED_EDGE('',*,*,#5997,.F.);
#8379=ORIENTED_EDGE('',*,*,#6310,.T.);
#8380=ORIENTED_EDGE('',*,*,#6001,.F.);
#8381=ORIENTED_EDGE('',*,*,#6314,.F.);
#8382=ORIENTED_EDGE('',*,*,#6238,.F.);
#8383=ORIENTED_EDGE('',*,*,#6311,.T.);
#8384=ORIENTED_EDGE('',*,*,#6241,.F.);
#8385=ORIENTED_EDGE('',*,*,#6315,.F.);
#8386=ORIENTED_EDGE('',*,*,#6245,.F.);
#8387=ORIENTED_EDGE('',*,*,#5857,.T.);
#8388=ORIENTED_EDGE('',*,*,#6246,.F.);
#8389=ORIENTED_EDGE('',*,*,#6316,.F.);
#8390=ORIENTED_EDGE('',*,*,#5974,.F.);
#8391=ORIENTED_EDGE('',*,*,#6312,.T.);
#8392=ORIENTED_EDGE('',*,*,#5980,.T.);
#8393=ORIENTED_EDGE('',*,*,#6317,.F.);
#8394=ORIENTED_EDGE('',*,*,#6313,.T.);
#8395=ORIENTED_EDGE('',*,*,#6314,.T.);
#8396=ORIENTED_EDGE('',*,*,#6000,.T.);
#8397=ORIENTED_EDGE('',*,*,#6318,.F.);
#8398=ORIENTED_EDGE('',*,*,#6319,.F.);
#8399=ORIENTED_EDGE('',*,*,#6316,.T.);
#8400=ORIENTED_EDGE('',*,*,#6315,.T.);
#8401=ORIENTED_EDGE('',*,*,#6320,.F.);
#8402=ORIENTED_EDGE('',*,*,#5975,.F.);
#8403=ORIENTED_EDGE('',*,*,#6317,.T.);
#8404=ORIENTED_EDGE('',*,*,#5979,.F.);
#8405=ORIENTED_EDGE('',*,*,#5854,.F.);
#8406=ORIENTED_EDGE('',*,*,#5998,.F.);
#8407=ORIENTED_EDGE('',*,*,#6318,.T.);
#8408=ORIENTED_EDGE('',*,*,#5999,.F.);
#8409=ORIENTED_EDGE('',*,*,#5853,.F.);
#8410=ORIENTED_EDGE('',*,*,#6242,.F.);
#8411=ORIENTED_EDGE('',*,*,#6319,.T.);
#8412=ORIENTED_EDGE('',*,*,#6244,.F.);
#8413=ORIENTED_EDGE('',*,*,#6321,.F.);
#8414=ORIENTED_EDGE('',*,*,#6239,.F.);
#8415=ORIENTED_EDGE('',*,*,#6320,.T.);
#8416=ORIENTED_EDGE('',*,*,#6240,.F.);
#8417=ORIENTED_EDGE('',*,*,#6322,.F.);
#8418=ORIENTED_EDGE('',*,*,#5976,.F.);
#8419=ORIENTED_EDGE('',*,*,#6322,.T.);
#8420=ORIENTED_EDGE('',*,*,#6321,.T.);
#8421=ORIENTED_EDGE('',*,*,#6323,.F.);
#8422=ORIENTED_EDGE('',*,*,#5977,.F.);
#8423=ORIENTED_EDGE('',*,*,#5852,.T.);
#8424=ORIENTED_EDGE('',*,*,#5978,.F.);
#8425=ORIENTED_EDGE('',*,*,#6323,.T.);
#8426=ORIENTED_EDGE('',*,*,#6243,.F.);
#8427=ORIENTED_EDGE('',*,*,#6324,.F.);
#8428=ORIENTED_EDGE('',*,*,#6325,.F.);
#8429=ORIENTED_EDGE('',*,*,#6326,.F.);
#8430=ORIENTED_EDGE('',*,*,#6327,.F.);
#8431=ORIENTED_EDGE('',*,*,#6263,.F.);
#8432=ORIENTED_EDGE('',*,*,#6328,.F.);
#8433=ORIENTED_EDGE('',*,*,#6016,.F.);
#8434=ORIENTED_EDGE('',*,*,#6325,.T.);
#8435=ORIENTED_EDGE('',*,*,#6260,.F.);
#8436=ORIENTED_EDGE('',*,*,#6329,.F.);
#8437=ORIENTED_EDGE('',*,*,#6179,.F.);
#8438=ORIENTED_EDGE('',*,*,#6326,.T.);
#8439=ORIENTED_EDGE('',*,*,#6178,.F.);
#8440=ORIENTED_EDGE('',*,*,#6330,.F.);
#8441=ORIENTED_EDGE('',*,*,#6186,.F.);
#8442=ORIENTED_EDGE('',*,*,#6324,.T.);
#8443=ORIENTED_EDGE('',*,*,#6185,.F.);
#8444=ORIENTED_EDGE('',*,*,#6331,.F.);
#8445=ORIENTED_EDGE('',*,*,#6261,.F.);
#8446=ORIENTED_EDGE('',*,*,#6332,.F.);
#8447=ORIENTED_EDGE('',*,*,#6262,.F.);
#8448=ORIENTED_EDGE('',*,*,#6333,.F.);
#8449=ORIENTED_EDGE('',*,*,#6195,.F.);
#8450=ORIENTED_EDGE('',*,*,#6328,.T.);
#8451=ORIENTED_EDGE('',*,*,#6332,.T.);
#8452=ORIENTED_EDGE('',*,*,#6334,.F.);
#8453=ORIENTED_EDGE('',*,*,#6329,.T.);
#8454=ORIENTED_EDGE('',*,*,#6327,.T.);
#8455=ORIENTED_EDGE('',*,*,#6335,.F.);
#8456=ORIENTED_EDGE('',*,*,#6336,.F.);
#8457=ORIENTED_EDGE('',*,*,#6330,.T.);
#8458=ORIENTED_EDGE('',*,*,#6337,.F.);
#8459=ORIENTED_EDGE('',*,*,#6333,.T.);
#8460=ORIENTED_EDGE('',*,*,#6331,.T.);
#8461=ORIENTED_EDGE('',*,*,#6338,.F.);
#8462=ORIENTED_EDGE('',*,*,#6334,.T.);
#8463=ORIENTED_EDGE('',*,*,#6194,.F.);
#8464=ORIENTED_EDGE('',*,*,#6339,.F.);
#8465=ORIENTED_EDGE('',*,*,#6017,.F.);
#8466=ORIENTED_EDGE('',*,*,#6335,.T.);
#8467=ORIENTED_EDGE('',*,*,#6015,.F.);
#8468=ORIENTED_EDGE('',*,*,#6340,.F.);
#8469=ORIENTED_EDGE('',*,*,#6180,.F.);
#8470=ORIENTED_EDGE('',*,*,#6337,.T.);
#8471=ORIENTED_EDGE('',*,*,#6181,.F.);
#8472=ORIENTED_EDGE('',*,*,#6341,.F.);
#8473=ORIENTED_EDGE('',*,*,#6257,.F.);
#8474=ORIENTED_EDGE('',*,*,#6336,.T.);
#8475=ORIENTED_EDGE('',*,*,#6256,.F.);
#8476=ORIENTED_EDGE('',*,*,#6342,.F.);
#8477=ORIENTED_EDGE('',*,*,#6187,.F.);
#8478=ORIENTED_EDGE('',*,*,#6338,.T.);
#8479=ORIENTED_EDGE('',*,*,#6184,.F.);
#8480=ORIENTED_EDGE('',*,*,#6343,.F.);
#8481=ORIENTED_EDGE('',*,*,#6192,.F.);
#8482=ORIENTED_EDGE('',*,*,#6344,.F.);
#8483=ORIENTED_EDGE('',*,*,#5957,.F.);
#8484=ORIENTED_EDGE('',*,*,#6345,.F.);
#8485=ORIENTED_EDGE('',*,*,#6193,.F.);
#8486=ORIENTED_EDGE('',*,*,#6345,.T.);
#8487=ORIENTED_EDGE('',*,*,#5956,.T.);
#8488=ORIENTED_EDGE('',*,*,#5850,.F.);
#8489=ORIENTED_EDGE('',*,*,#6339,.T.);
#8490=ORIENTED_EDGE('',*,*,#6341,.T.);
#8491=ORIENTED_EDGE('',*,*,#6340,.T.);
#8492=ORIENTED_EDGE('',*,*,#6346,.F.);
#8493=ORIENTED_EDGE('',*,*,#6347,.F.);
#8494=ORIENTED_EDGE('',*,*,#6342,.T.);
#8495=ORIENTED_EDGE('',*,*,#6348,.F.);
#8496=ORIENTED_EDGE('',*,*,#6344,.T.);
#8497=ORIENTED_EDGE('',*,*,#6343,.T.);
#8498=ORIENTED_EDGE('',*,*,#6349,.F.);
#8499=ORIENTED_EDGE('',*,*,#5958,.F.);
#8500=ORIENTED_EDGE('',*,*,#6346,.T.);
#8501=ORIENTED_EDGE('',*,*,#6014,.F.);
#8502=ORIENTED_EDGE('',*,*,#6350,.F.);
#8503=ORIENTED_EDGE('',*,*,#6258,.F.);
#8504=ORIENTED_EDGE('',*,*,#6348,.T.);
#8505=ORIENTED_EDGE('',*,*,#6259,.F.);
#8506=ORIENTED_EDGE('',*,*,#6351,.F.);
#8507=ORIENTED_EDGE('',*,*,#6189,.F.);
#8508=ORIENTED_EDGE('',*,*,#6347,.T.);
#8509=ORIENTED_EDGE('',*,*,#6188,.F.);
#8510=ORIENTED_EDGE('',*,*,#6352,.F.);
#8511=ORIENTED_EDGE('',*,*,#6182,.F.);
#8512=ORIENTED_EDGE('',*,*,#6349,.T.);
#8513=ORIENTED_EDGE('',*,*,#6183,.F.);
#8514=ORIENTED_EDGE('',*,*,#6353,.F.);
#8515=ORIENTED_EDGE('',*,*,#5959,.F.);
#8516=ORIENTED_EDGE('',*,*,#6354,.F.);
#8517=ORIENTED_EDGE('',*,*,#5848,.T.);
#8518=ORIENTED_EDGE('',*,*,#6355,.F.);
#8519=ORIENTED_EDGE('',*,*,#6351,.T.);
#8520=ORIENTED_EDGE('',*,*,#6350,.T.);
#8521=ORIENTED_EDGE('',*,*,#6356,.F.);
#8522=ORIENTED_EDGE('',*,*,#6353,.T.);
#8523=ORIENTED_EDGE('',*,*,#6352,.T.);
#8524=ORIENTED_EDGE('',*,*,#6357,.F.);
#8525=ORIENTED_EDGE('',*,*,#5960,.F.);
#8526=ORIENTED_EDGE('',*,*,#6355,.T.);
#8527=ORIENTED_EDGE('',*,*,#5955,.F.);
#8528=ORIENTED_EDGE('',*,*,#6358,.F.);
#8529=ORIENTED_EDGE('',*,*,#6201,.F.);
#8530=ORIENTED_EDGE('',*,*,#6359,.F.);
#8531=ORIENTED_EDGE('',*,*,#6202,.F.);
#8532=ORIENTED_EDGE('',*,*,#6360,.F.);
#8533=ORIENTED_EDGE('',*,*,#6196,.F.);
#8534=ORIENTED_EDGE('',*,*,#6354,.T.);
#8535=ORIENTED_EDGE('',*,*,#6200,.F.);
#8536=ORIENTED_EDGE('',*,*,#6361,.F.);
#8537=ORIENTED_EDGE('',*,*,#6018,.F.);
#8538=ORIENTED_EDGE('',*,*,#6356,.T.);
#8539=ORIENTED_EDGE('',*,*,#6013,.F.);
#8540=ORIENTED_EDGE('',*,*,#6362,.F.);
#8541=ORIENTED_EDGE('',*,*,#6190,.F.);
#8542=ORIENTED_EDGE('',*,*,#6357,.T.);
#8543=ORIENTED_EDGE('',*,*,#6191,.F.);
#8544=ORIENTED_EDGE('',*,*,#6363,.F.);
#8545=ORIENTED_EDGE('',*,*,#5961,.F.);
#8546=ORIENTED_EDGE('',*,*,#6358,.T.);
#8547=ORIENTED_EDGE('',*,*,#5954,.F.);
#8548=ORIENTED_EDGE('',*,*,#6364,.F.);
#8549=ORIENTED_EDGE('',*,*,#6360,.T.);
#8550=ORIENTED_EDGE('',*,*,#6361,.T.);
#8551=ORIENTED_EDGE('',*,*,#6359,.T.);
#8552=ORIENTED_EDGE('',*,*,#6365,.F.);
#8553=ORIENTED_EDGE('',*,*,#6019,.T.);
#8554=ORIENTED_EDGE('',*,*,#6363,.T.);
#8555=ORIENTED_EDGE('',*,*,#6362,.T.);
#8556=ORIENTED_EDGE('',*,*,#5844,.F.);
#8557=ORIENTED_EDGE('',*,*,#5843,.F.);
#8558=ORIENTED_EDGE('',*,*,#5962,.T.);
#8559=ORIENTED_EDGE('',*,*,#6364,.T.);
#8560=ORIENTED_EDGE('',*,*,#5953,.F.);
#8561=ORIENTED_EDGE('',*,*,#6366,.F.);
#8562=ORIENTED_EDGE('',*,*,#6197,.F.);
#8563=ORIENTED_EDGE('',*,*,#6367,.F.);
#8564=ORIENTED_EDGE('',*,*,#6198,.F.);
#8565=ORIENTED_EDGE('',*,*,#6368,.F.);
#8566=ORIENTED_EDGE('',*,*,#6203,.F.);
#8567=ORIENTED_EDGE('',*,*,#6365,.T.);
#8568=ORIENTED_EDGE('',*,*,#6199,.F.);
#8569=ORIENTED_EDGE('',*,*,#6369,.F.);
#8570=ORIENTED_EDGE('',*,*,#6020,.F.);
#8571=ORIENTED_EDGE('',*,*,#6370,.F.);
#8572=ORIENTED_EDGE('',*,*,#6012,.F.);
#8573=ORIENTED_EDGE('',*,*,#6371,.F.);
#8574=ORIENTED_EDGE('',*,*,#6212,.F.);
#8575=ORIENTED_EDGE('',*,*,#6366,.T.);
#8576=ORIENTED_EDGE('',*,*,#5952,.F.);
#8577=ORIENTED_EDGE('',*,*,#6372,.F.);
#8578=ORIENTED_EDGE('',*,*,#6368,.T.);
#8579=ORIENTED_EDGE('',*,*,#6369,.T.);
#8580=ORIENTED_EDGE('',*,*,#6367,.T.);
#8581=ORIENTED_EDGE('',*,*,#6373,.F.);
#8582=ORIENTED_EDGE('',*,*,#6021,.T.);
#8583=ORIENTED_EDGE('',*,*,#6371,.T.);
#8584=ORIENTED_EDGE('',*,*,#6026,.T.);
#8585=ORIENTED_EDGE('',*,*,#6374,.F.);
#8586=ORIENTED_EDGE('',*,*,#6375,.F.);
#8587=ORIENTED_EDGE('',*,*,#5846,.T.);
#8588=ORIENTED_EDGE('',*,*,#6370,.T.);
#8589=ORIENTED_EDGE('',*,*,#6376,.F.);
#8590=ORIENTED_EDGE('',*,*,#6372,.T.);
#8591=ORIENTED_EDGE('',*,*,#5951,.F.);
#8592=ORIENTED_EDGE('',*,*,#6377,.F.);
#8593=ORIENTED_EDGE('',*,*,#6204,.F.);
#8594=ORIENTED_EDGE('',*,*,#6373,.T.);
#8595=ORIENTED_EDGE('',*,*,#6205,.F.);
#8596=ORIENTED_EDGE('',*,*,#6378,.F.);
#8597=ORIENTED_EDGE('',*,*,#6022,.F.);
#8598=ORIENTED_EDGE('',*,*,#6374,.T.);
#8599=ORIENTED_EDGE('',*,*,#6025,.F.);
#8600=ORIENTED_EDGE('',*,*,#6379,.F.);
#8601=ORIENTED_EDGE('',*,*,#6209,.F.);
#8602=ORIENTED_EDGE('',*,*,#6375,.T.);
#8603=ORIENTED_EDGE('',*,*,#6208,.F.);
#8604=ORIENTED_EDGE('',*,*,#6380,.F.);
#8605=ORIENTED_EDGE('',*,*,#6210,.F.);
#8606=ORIENTED_EDGE('',*,*,#6376,.T.);
#8607=ORIENTED_EDGE('',*,*,#6211,.F.);
#8608=ORIENTED_EDGE('',*,*,#6381,.F.);
#8609=ORIENTED_EDGE('',*,*,#5963,.F.);
#8610=ORIENTED_EDGE('',*,*,#6378,.T.);
#8611=ORIENTED_EDGE('',*,*,#6377,.T.);
#8612=ORIENTED_EDGE('',*,*,#5841,.F.);
#8613=ORIENTED_EDGE('',*,*,#6379,.T.);
#8614=ORIENTED_EDGE('',*,*,#6024,.T.);
#8615=ORIENTED_EDGE('',*,*,#6382,.F.);
#8616=ORIENTED_EDGE('',*,*,#6383,.F.);
#8617=ORIENTED_EDGE('',*,*,#6381,.T.);
#8618=ORIENTED_EDGE('',*,*,#6380,.T.);
#8619=ORIENTED_EDGE('',*,*,#6384,.F.);
#8620=ORIENTED_EDGE('',*,*,#5964,.F.);
#8621=ORIENTED_EDGE('',*,*,#6382,.T.);
#8622=ORIENTED_EDGE('',*,*,#6023,.F.);
#8623=ORIENTED_EDGE('',*,*,#6385,.F.);
#8624=ORIENTED_EDGE('',*,*,#6213,.F.);
#8625=ORIENTED_EDGE('',*,*,#6383,.T.);
#8626=ORIENTED_EDGE('',*,*,#6215,.F.);
#8627=ORIENTED_EDGE('',*,*,#6386,.F.);
#8628=ORIENTED_EDGE('',*,*,#6206,.F.);
#8629=ORIENTED_EDGE('',*,*,#6384,.T.);
#8630=ORIENTED_EDGE('',*,*,#6207,.F.);
#8631=ORIENTED_EDGE('',*,*,#6387,.F.);
#8632=ORIENTED_EDGE('',*,*,#5965,.F.);
#8633=ORIENTED_EDGE('',*,*,#6385,.T.);
#8634=ORIENTED_EDGE('',*,*,#5839,.T.);
#8635=ORIENTED_EDGE('',*,*,#6388,.F.);
#8636=ORIENTED_EDGE('',*,*,#6387,.T.);
#8637=ORIENTED_EDGE('',*,*,#6386,.T.);
#8638=ORIENTED_EDGE('',*,*,#6389,.F.);
#8639=ORIENTED_EDGE('',*,*,#5966,.F.);
#8640=ORIENTED_EDGE('',*,*,#6388,.T.);
#8641=ORIENTED_EDGE('',*,*,#5967,.F.);
#8642=ORIENTED_EDGE('',*,*,#6389,.T.);
#8643=ORIENTED_EDGE('',*,*,#6214,.F.);
#10920=CYLINDRICAL_SURFACE('',#11897,160.);
#10921=CYLINDRICAL_SURFACE('',#11904,2.5);
#10922=CYLINDRICAL_SURFACE('',#11907,2.5);
#10923=CYLINDRICAL_SURFACE('',#11911,2.5);
#10924=CYLINDRICAL_SURFACE('',#11943,4.49999999999998);
#10925=CYLINDRICAL_SURFACE('',#11948,4.49999999999998);
#10926=CYLINDRICAL_SURFACE('',#11953,4.49999999999998);
#10927=CYLINDRICAL_SURFACE('',#11958,4.49999999999998);
#10928=CYLINDRICAL_SURFACE('',#11963,4.49999999999998);
#10929=CYLINDRICAL_SURFACE('',#11968,4.49999999999998);
#10930=CYLINDRICAL_SURFACE('',#11970,195.);
#10931=CYLINDRICAL_SURFACE('',#11978,35.5);
#10932=CYLINDRICAL_SURFACE('',#11979,4.5);
#10933=CYLINDRICAL_SURFACE('',#11982,4.5);
#10934=CYLINDRICAL_SURFACE('',#11985,4.5);
#10935=CYLINDRICAL_SURFACE('',#11988,4.5);
#10936=CYLINDRICAL_SURFACE('',#11991,25.);
#10937=CYLINDRICAL_SURFACE('',#11994,160.);
#10938=CYLINDRICAL_SURFACE('',#11998,15.);
#10939=CYLINDRICAL_SURFACE('',#12003,170.);
#10940=CYLINDRICAL_SURFACE('',#12031,175.);
#10941=CYLINDRICAL_SURFACE('',#12039,285.);
#10942=CYLINDRICAL_SURFACE('',#12066,100.);
#10943=CYLINDRICAL_SURFACE('',#12069,100.);
#10944=CYLINDRICAL_SURFACE('',#12074,100.);
#10945=CYLINDRICAL_SURFACE('',#12077,35.);
#10946=CYLINDRICAL_SURFACE('',#12084,35.);
#10947=CYLINDRICAL_SURFACE('',#12091,35.);
#10948=CYLINDRICAL_SURFACE('',#12097,35.);
#10949=CYLINDRICAL_SURFACE('',#12111,185.);
#10950=CYLINDRICAL_SURFACE('',#12119,275.);
#10951=CYLINDRICAL_SURFACE('',#12137,110.);
#10952=CYLINDRICAL_SURFACE('',#12140,110.);
#10953=CYLINDRICAL_SURFACE('',#12145,110.);
#10954=CYLINDRICAL_SURFACE('',#12148,25.);
#10955=CYLINDRICAL_SURFACE('',#12155,25.);
#10956=CYLINDRICAL_SURFACE('',#12162,25.);
#10957=CYLINDRICAL_SURFACE('',#12168,25.);
#10958=CYLINDRICAL_SURFACE('',#12217,2.5);
#10959=CYLINDRICAL_SURFACE('',#12219,2.5);
#10960=CYLINDRICAL_SURFACE('',#12234,2.5);
#10961=CYLINDRICAL_SURFACE('',#12236,2.5);
#10962=CYLINDRICAL_SURFACE('',#12237,2.5);
#10963=CYLINDRICAL_SURFACE('',#12239,2.50000000000001);
#10964=CYLINDRICAL_SURFACE('',#12241,2.5);
#10965=CYLINDRICAL_SURFACE('',#12243,2.5);
#10966=CYLINDRICAL_SURFACE('',#12245,2.50000000000001);
#10967=CYLINDRICAL_SURFACE('',#12247,2.5);
#10968=CYLINDRICAL_SURFACE('',#12249,2.5);
#10969=CYLINDRICAL_SURFACE('',#12251,2.5);
#10970=CYLINDRICAL_SURFACE('',#12266,2.5);
#10971=CYLINDRICAL_SURFACE('',#12267,2.5);
#10972=CYLINDRICAL_SURFACE('',#12269,2.5);
#10973=CYLINDRICAL_SURFACE('',#12271,2.5);
#10974=CYLINDRICAL_SURFACE('',#12273,2.5);
#10975=CYLINDRICAL_SURFACE('',#12281,2.5);
#10976=CYLINDRICAL_SURFACE('',#12283,2.5);
#10977=CYLINDRICAL_SURFACE('',#12284,2.5);
#10978=CYLINDRICAL_SURFACE('',#12286,2.5);
#10979=CYLINDRICAL_SURFACE('',#12288,2.5);
#10980=CYLINDRICAL_SURFACE('',#12290,2.5);
#10981=CYLINDRICAL_SURFACE('',#12299,2.5);
#10982=CYLINDRICAL_SURFACE('',#12300,2.5);
#10983=CYLINDRICAL_SURFACE('',#12302,2.5);
#10984=CYLINDRICAL_SURFACE('',#12310,2.5);
#10985=CYLINDRICAL_SURFACE('',#12311,2.5);
#10986=CYLINDRICAL_SURFACE('',#12312,2.5);
#10987=CYLINDRICAL_SURFACE('',#12313,2.5);
#10988=CYLINDRICAL_SURFACE('',#12321,2.50000000000001);
#10989=CYLINDRICAL_SURFACE('',#12324,2.5);
#10990=CYLINDRICAL_SURFACE('',#12326,2.5);
#10991=CYLINDRICAL_SURFACE('',#12328,2.50000000000001);
#10992=CYLINDRICAL_SURFACE('',#12330,2.5);
#10993=CYLINDRICAL_SURFACE('',#12342,2.5);
#10994=CYLINDRICAL_SURFACE('',#12343,2.5);
#10995=CYLINDRICAL_SURFACE('',#12345,2.5);
#10996=CYLINDRICAL_SURFACE('',#12347,2.5);
#10997=CYLINDRICAL_SURFACE('',#12349,2.5);
#10998=CYLINDRICAL_SURFACE('',#12359,2.5);
#10999=CYLINDRICAL_SURFACE('',#12361,2.5);
#11000=CYLINDRICAL_SURFACE('',#12363,2.5);
#11001=CYLINDRICAL_SURFACE('',#12364,2.5);
#11002=CYLINDRICAL_SURFACE('',#12374,2.5);
#11003=CYLINDRICAL_SURFACE('',#12376,2.5);
#11004=CYLINDRICAL_SURFACE('',#12378,2.5);
#11005=CYLINDRICAL_SURFACE('',#12384,2.5);
#11006=CYLINDRICAL_SURFACE('',#12386,2.5);
#11007=CYLINDRICAL_SURFACE('',#12388,2.5);
#11008=CYLINDRICAL_SURFACE('',#12390,2.5);
#11009=CYLINDRICAL_SURFACE('',#12403,2.5);
#11010=CYLINDRICAL_SURFACE('',#12405,2.5);
#11011=CYLINDRICAL_SURFACE('',#12407,2.5);
#11012=CYLINDRICAL_SURFACE('',#12415,2.5);
#11013=CYLINDRICAL_SURFACE('',#12417,2.5);
#11014=CYLINDRICAL_SURFACE('',#12418,2.5);
#11142=ADVANCED_FACE('',(#703),#10920,.F.);
#11143=ADVANCED_FACE('',(#704),#658,.T.);
#11144=ADVANCED_FACE('',(#705),#10921,.F.);
#11145=ADVANCED_FACE('',(#706),#10922,.F.);
#11146=ADVANCED_FACE('',(#707),#10923,.F.);
#11147=ADVANCED_FACE('',(#708),#634,.F.);
#11148=ADVANCED_FACE('',(#709),#635,.F.);
#11149=ADVANCED_FACE('',(#710),#636,.F.);
#11150=ADVANCED_FACE('',(#711),#637,.F.);
#11151=ADVANCED_FACE('',(#712),#659,.T.);
#11152=ADVANCED_FACE('',(#713),#660,.T.);
#11153=ADVANCED_FACE('',(#714),#617,.F.);
#11154=ADVANCED_FACE('',(#715),#10924,.F.);
#11155=ADVANCED_FACE('',(#716),#618,.F.);
#11156=ADVANCED_FACE('',(#717),#10925,.F.);
#11157=ADVANCED_FACE('',(#718),#619,.F.);
#11158=ADVANCED_FACE('',(#719),#10926,.F.);
#11159=ADVANCED_FACE('',(#720),#620,.F.);
#11160=ADVANCED_FACE('',(#721),#10927,.F.);
#11161=ADVANCED_FACE('',(#722),#621,.F.);
#11162=ADVANCED_FACE('',(#723),#10928,.F.);
#11163=ADVANCED_FACE('',(#724),#622,.F.);
#11164=ADVANCED_FACE('',(#725),#10929,.F.);
#11165=ADVANCED_FACE('',(#726),#10930,.T.);
#11166=ADVANCED_FACE('',(#727),#623,.F.);
#11167=ADVANCED_FACE('',(#728),#624,.F.);
#11168=ADVANCED_FACE('',(#729),#10931,.F.);
#11169=ADVANCED_FACE('',(#730),#10932,.F.);
#11170=ADVANCED_FACE('',(#731),#10933,.F.);
#11171=ADVANCED_FACE('',(#732),#10934,.F.);
#11172=ADVANCED_FACE('',(#733),#10935,.F.);
#11173=ADVANCED_FACE('',(#734),#10936,.T.);
#11174=ADVANCED_FACE('',(#735),#10937,.F.);
#11175=ADVANCED_FACE('',(#736),#10938,.F.);
#11176=ADVANCED_FACE('',(#737,#542,#543),#10939,.T.);
#11177=ADVANCED_FACE('',(#738,#544,#545),#205,.F.);
#11178=ADVANCED_FACE('',(#739,#546,#547),#206,.F.);
#11179=ADVANCED_FACE('',(#740,#548,#549),#207,.T.);
#11180=ADVANCED_FACE('',(#741,#550),#208,.F.);
#11181=ADVANCED_FACE('',(#742),#10940,.F.);
#11182=ADVANCED_FACE('',(#743),#209,.F.);
#11183=ADVANCED_FACE('',(#744),#10941,.T.);
#11184=ADVANCED_FACE('',(#745),#210,.F.);
#11185=ADVANCED_FACE('',(#746,#551),#211,.T.);
#11186=ADVANCED_FACE('',(#747),#212,.F.);
#11187=ADVANCED_FACE('',(#748),#213,.F.);
#11188=ADVANCED_FACE('',(#749),#214,.F.);
#11189=ADVANCED_FACE('',(#750),#215,.F.);
#11190=ADVANCED_FACE('',(#751),#10942,.F.);
#11191=ADVANCED_FACE('',(#752),#10943,.F.);
#11192=ADVANCED_FACE('',(#753),#10944,.F.);
#11193=ADVANCED_FACE('',(#754),#10945,.T.);
#11194=ADVANCED_FACE('',(#755),#89,.T.);
#11195=ADVANCED_FACE('',(#756),#90,.T.);
#11196=ADVANCED_FACE('',(#757),#661,.T.);
#11197=ADVANCED_FACE('',(#758),#662,.T.);
#11198=ADVANCED_FACE('',(#759),#10946,.T.);
#11199=ADVANCED_FACE('',(#760),#91,.T.);
#11200=ADVANCED_FACE('',(#761),#92,.T.);
#11201=ADVANCED_FACE('',(#762),#663,.T.);
#11202=ADVANCED_FACE('',(#763),#664,.T.);
#11203=ADVANCED_FACE('',(#764),#10947,.T.);
#11204=ADVANCED_FACE('',(#765),#665,.T.);
#11205=ADVANCED_FACE('',(#766),#93,.T.);
#11206=ADVANCED_FACE('',(#767),#666,.T.);
#11207=ADVANCED_FACE('',(#768),#10948,.T.);
#11208=ADVANCED_FACE('',(#769),#667,.T.);
#11209=ADVANCED_FACE('',(#770),#94,.T.);
#11210=ADVANCED_FACE('',(#771),#668,.T.);
#11211=ADVANCED_FACE('',(#772),#95,.F.);
#11212=ADVANCED_FACE('',(#773),#669,.F.);
#11213=ADVANCED_FACE('',(#774),#96,.F.);
#11214=ADVANCED_FACE('',(#775),#97,.F.);
#11215=ADVANCED_FACE('',(#776),#670,.F.);
#11216=ADVANCED_FACE('',(#777),#98,.F.);
#11217=ADVANCED_FACE('',(#778,#552),#216,.T.);
#11218=ADVANCED_FACE('',(#779),#10949,.T.);
#11219=ADVANCED_FACE('',(#780),#217,.T.);
#11220=ADVANCED_FACE('',(#781),#10950,.F.);
#11221=ADVANCED_FACE('',(#782),#218,.T.);
#11222=ADVANCED_FACE('',(#783),#219,.T.);
#11223=ADVANCED_FACE('',(#784),#220,.T.);
#11224=ADVANCED_FACE('',(#785),#221,.T.);
#11225=ADVANCED_FACE('',(#786),#222,.T.);
#11226=ADVANCED_FACE('',(#787),#10951,.T.);
#11227=ADVANCED_FACE('',(#788),#10952,.T.);
#11228=ADVANCED_FACE('',(#789),#10953,.T.);
#11229=ADVANCED_FACE('',(#790),#10954,.F.);
#11230=ADVANCED_FACE('',(#791),#99,.F.);
#11231=ADVANCED_FACE('',(#792),#100,.F.);
#11232=ADVANCED_FACE('',(#793),#671,.F.);
#11233=ADVANCED_FACE('',(#794),#672,.F.);
#11234=ADVANCED_FACE('',(#795),#10955,.F.);
#11235=ADVANCED_FACE('',(#796),#101,.F.);
#11236=ADVANCED_FACE('',(#797),#102,.F.);
#11237=ADVANCED_FACE('',(#798),#673,.F.);
#11238=ADVANCED_FACE('',(#799),#674,.F.);
#11239=ADVANCED_FACE('',(#800),#10956,.F.);
#11240=ADVANCED_FACE('',(#801),#675,.F.);
#11241=ADVANCED_FACE('',(#802),#103,.F.);
#11242=ADVANCED_FACE('',(#803),#676,.F.);
#11243=ADVANCED_FACE('',(#804),#10957,.F.);
#11244=ADVANCED_FACE('',(#805),#677,.F.);
#11245=ADVANCED_FACE('',(#806),#104,.F.);
#11246=ADVANCED_FACE('',(#807),#678,.F.);
#11247=ADVANCED_FACE('',(#808),#105,.T.);
#11248=ADVANCED_FACE('',(#809),#679,.T.);
#11249=ADVANCED_FACE('',(#810),#106,.T.);
#11250=ADVANCED_FACE('',(#811),#107,.T.);
#11251=ADVANCED_FACE('',(#812),#680,.T.);
#11252=ADVANCED_FACE('',(#813),#108,.T.);
#11253=ADVANCED_FACE('',(#814),#223,.T.);
#11254=ADVANCED_FACE('',(#815,#553,#554),#224,.T.);
#11255=ADVANCED_FACE('',(#816),#225,.T.);
#11256=ADVANCED_FACE('',(#817),#226,.F.);
#11257=ADVANCED_FACE('',(#818),#227,.F.);
#11258=ADVANCED_FACE('',(#819),#228,.F.);
#11259=ADVANCED_FACE('',(#820),#229,.T.);
#11260=ADVANCED_FACE('',(#821),#230,.T.);
#11261=ADVANCED_FACE('',(#822),#231,.F.);
#11262=ADVANCED_FACE('',(#823),#232,.T.);
#11263=ADVANCED_FACE('',(#824),#233,.F.);
#11264=ADVANCED_FACE('',(#825),#234,.T.);
#11265=ADVANCED_FACE('',(#826),#235,.F.);
#11266=ADVANCED_FACE('',(#827),#236,.T.);
#11267=ADVANCED_FACE('',(#828),#237,.F.);
#11268=ADVANCED_FACE('',(#829),#238,.T.);
#11269=ADVANCED_FACE('',(#830),#239,.F.);
#11270=ADVANCED_FACE('',(#831),#240,.F.);
#11271=ADVANCED_FACE('',(#832),#241,.T.);
#11272=ADVANCED_FACE('',(#833),#242,.T.);
#11273=ADVANCED_FACE('',(#834),#243,.F.);
#11274=ADVANCED_FACE('',(#835),#244,.F.);
#11275=ADVANCED_FACE('',(#836),#245,.T.);
#11276=ADVANCED_FACE('',(#837,#555,#556,#557,#558,#559,#560,#561),#246,
 .F.);
#11277=ADVANCED_FACE('',(#838,#562,#563,#564,#565,#566,#567,#568),#247,
 .T.);
#11278=ADVANCED_FACE('',(#839),#10958,.F.);
#11279=ADVANCED_FACE('',(#840),#10959,.T.);
#11280=ADVANCED_FACE('',(#841),#681,.F.);
#11281=ADVANCED_FACE('',(#842),#638,.T.);
#11282=ADVANCED_FACE('',(#843),#639,.T.);
#11283=ADVANCED_FACE('',(#844),#682,.F.);
#11284=ADVANCED_FACE('',(#845),#109,.F.);
#11285=ADVANCED_FACE('',(#846),#10960,.F.);
#11286=ADVANCED_FACE('',(#847),#10961,.T.);
#11287=ADVANCED_FACE('',(#848),#10962,.T.);
#11288=ADVANCED_FACE('',(#849),#10963,.T.);
#11289=ADVANCED_FACE('',(#850),#10964,.T.);
#11290=ADVANCED_FACE('',(#851),#10965,.T.);
#11291=ADVANCED_FACE('',(#852),#10966,.T.);
#11292=ADVANCED_FACE('',(#853),#10967,.F.);
#11293=ADVANCED_FACE('',(#854),#10968,.T.);
#11294=ADVANCED_FACE('',(#855),#10969,.F.);
#11295=ADVANCED_FACE('',(#856),#110,.F.);
#11296=ADVANCED_FACE('',(#857),#640,.T.);
#11297=ADVANCED_FACE('',(#858),#641,.T.);
#11298=ADVANCED_FACE('',(#859),#642,.T.);
#11299=ADVANCED_FACE('',(#860),#683,.F.);
#11300=ADVANCED_FACE('',(#861),#111,.F.);
#11301=ADVANCED_FACE('',(#862),#684,.F.);
#11302=ADVANCED_FACE('',(#863),#10970,.T.);
#11303=ADVANCED_FACE('',(#864),#10971,.T.);
#11304=ADVANCED_FACE('',(#865),#10972,.T.);
#11305=ADVANCED_FACE('',(#866),#10973,.T.);
#11306=ADVANCED_FACE('',(#867),#10974,.F.);
#11307=ADVANCED_FACE('',(#868),#685,.F.);
#11308=ADVANCED_FACE('',(#869),#112,.F.);
#11309=ADVANCED_FACE('',(#870),#643,.T.);
#11310=ADVANCED_FACE('',(#871),#644,.T.);
#11311=ADVANCED_FACE('',(#872),#10975,.F.);
#11312=ADVANCED_FACE('',(#873),#10976,.T.);
#11313=ADVANCED_FACE('',(#874),#10977,.T.);
#11314=ADVANCED_FACE('',(#875),#10978,.T.);
#11315=ADVANCED_FACE('',(#876),#10979,.F.);
#11316=ADVANCED_FACE('',(#877),#10980,.F.);
#11317=ADVANCED_FACE('',(#878),#113,.F.);
#11318=ADVANCED_FACE('',(#879),#645,.T.);
#11319=ADVANCED_FACE('',(#880),#686,.F.);
#11320=ADVANCED_FACE('',(#881),#687,.F.);
#11321=ADVANCED_FACE('',(#882),#10981,.T.);
#11322=ADVANCED_FACE('',(#883),#10982,.F.);
#11323=ADVANCED_FACE('',(#884),#10983,.T.);
#11324=ADVANCED_FACE('',(#885),#688,.F.);
#11325=ADVANCED_FACE('',(#886),#114,.F.);
#11326=ADVANCED_FACE('',(#887),#689,.F.);
#11327=ADVANCED_FACE('',(#888),#115,.F.);
#11328=ADVANCED_FACE('',(#889),#10984,.F.);
#11329=ADVANCED_FACE('',(#890),#10985,.F.);
#11330=ADVANCED_FACE('',(#891),#10986,.T.);
#11331=ADVANCED_FACE('',(#892),#10987,.F.);
#11332=ADVANCED_FACE('',(#893),#116,.F.);
#11333=ADVANCED_FACE('',(#894),#690,.F.);
#11334=ADVANCED_FACE('',(#895),#646,.T.);
#11335=ADVANCED_FACE('',(#896),#10988,.T.);
#11336=ADVANCED_FACE('',(#897),#10989,.T.);
#11337=ADVANCED_FACE('',(#898),#10990,.T.);
#11338=ADVANCED_FACE('',(#899),#10991,.T.);
#11339=ADVANCED_FACE('',(#900),#10992,.T.);
#11340=ADVANCED_FACE('',(#901),#647,.T.);
#11341=ADVANCED_FACE('',(#902),#648,.T.);
#11342=ADVANCED_FACE('',(#903),#649,.T.);
#11343=ADVANCED_FACE('',(#904),#650,.T.);
#11344=ADVANCED_FACE('',(#905),#10993,.T.);
#11345=ADVANCED_FACE('',(#906),#10994,.T.);
#11346=ADVANCED_FACE('',(#907),#10995,.T.);
#11347=ADVANCED_FACE('',(#908),#10996,.T.);
#11348=ADVANCED_FACE('',(#909),#10997,.T.);
#11349=ADVANCED_FACE('',(#910),#691,.F.);
#11350=ADVANCED_FACE('',(#911),#117,.F.);
#11351=ADVANCED_FACE('',(#912),#651,.T.);
#11352=ADVANCED_FACE('',(#913),#652,.T.);
#11353=ADVANCED_FACE('',(#914),#118,.F.);
#11354=ADVANCED_FACE('',(#915),#10998,.T.);
#11355=ADVANCED_FACE('',(#916),#10999,.T.);
#11356=ADVANCED_FACE('',(#917),#11000,.T.);
#11357=ADVANCED_FACE('',(#918),#11001,.F.);
#11358=ADVANCED_FACE('',(#919),#653,.F.);
#11359=ADVANCED_FACE('',(#920),#654,.T.);
#11360=ADVANCED_FACE('',(#921),#119,.F.);
#11361=ADVANCED_FACE('',(#922),#692,.F.);
#11362=ADVANCED_FACE('',(#923),#11002,.T.);
#11363=ADVANCED_FACE('',(#924),#11003,.F.);
#11364=ADVANCED_FACE('',(#925),#11004,.T.);
#11365=ADVANCED_FACE('',(#926),#693,.F.);
#11366=ADVANCED_FACE('',(#927),#120,.F.);
#11367=ADVANCED_FACE('',(#928),#694,.F.);
#11368=ADVANCED_FACE('',(#929),#121,.F.);
#11369=ADVANCED_FACE('',(#930),#11005,.F.);
#11370=ADVANCED_FACE('',(#931),#11006,.T.);
#11371=ADVANCED_FACE('',(#932),#11007,.F.);
#11372=ADVANCED_FACE('',(#933),#11008,.F.);
#11373=ADVANCED_FACE('',(#934),#122,.F.);
#11374=ADVANCED_FACE('',(#935),#695,.F.);
#11375=ADVANCED_FACE('',(#936),#696,.F.);
#11376=ADVANCED_FACE('',(#937),#655,.F.);
#11377=ADVANCED_FACE('',(#938),#697,.F.);
#11378=ADVANCED_FACE('',(#939),#11009,.F.);
#11379=ADVANCED_FACE('',(#940),#11010,.F.);
#11380=ADVANCED_FACE('',(#941),#11011,.T.);
#11381=ADVANCED_FACE('',(#942),#698,.F.);
#11382=ADVANCED_FACE('',(#943),#656,.F.);
#11383=ADVANCED_FACE('',(#944),#699,.F.);
#11384=ADVANCED_FACE('',(#945),#123,.F.);
#11385=ADVANCED_FACE('',(#946),#11012,.F.);
#11386=ADVANCED_FACE('',(#947),#11013,.T.);
#11387=ADVANCED_FACE('',(#948),#11014,.F.);
#11388=ADVANCED_FACE('',(#949),#657,.F.);
#11389=ADVANCED_FACE('',(#950),#124,.F.);
#11390=ADVANCED_FACE('',(#951),#700,.F.);
#11823=CLOSED_SHELL('',(#11142,#11143,#11144,#11145,#11146,#11147,#11148,
#11149,#11150,#11151,#11152,#11153,#11154,#11155,#11156,#11157,#11158,#11159,
#11160,#11161,#11162,#11163,#11164,#11165,#11166,#11167,#11168,#11169,#11170,
#11171,#11172,#11173,#11174,#11175,#11176,#11177,#11178,#11179,#11180,#11181,
#11182,#11183,#11184,#11185,#11186,#11187,#11188,#11189,#11190,#11191,#11192,
#11193,#11194,#11195,#11196,#11197,#11198,#11199,#11200,#11201,#11202,#11203,
#11204,#11205,#11206,#11207,#11208,#11209,#11210,#11211,#11212,#11213,#11214,
#11215,#11216,#11217,#11218,#11219,#11220,#11221,#11222,#11223,#11224,#11225,
#11226,#11227,#11228,#11229,#11230,#11231,#11232,#11233,#11234,#11235,#11236,
#11237,#11238,#11239,#11240,#11241,#11242,#11243,#11244,#11245,#11246,#11247,
#11248,#11249,#11250,#11251,#11252,#11253,#11254,#11255,#11256,#11257,#11258,
#11259,#11260,#11261,#11262,#11263,#11264,#11265,#11266,#11267,#11268,#11269,
#11270,#11271,#11272,#11273,#11274,#11275,#11276,#11277,#11278,#11279,#11280,
#11281,#11282,#11283,#11284,#11285,#11286,#11287,#11288,#11289,#11290,#11291,
#11292,#11293,#11294,#11295,#11296,#11297,#11298,#11299,#11300,#11301,#11302,
#11303,#11304,#11305,#11306,#11307,#11308,#11309,#11310,#11311,#11312,#11313,
#11314,#11315,#11316,#11317,#11318,#11319,#11320,#11321,#11322,#11323,#11324,
#11325,#11326,#11327,#11328,#11329,#11330,#11331,#11332,#11333,#11334,#11335,
#11336,#11337,#11338,#11339,#11340,#11341,#11342,#11343,#11344,#11345,#11346,
#11347,#11348,#11349,#11350,#11351,#11352,#11353,#11354,#11355,#11356,#11357,
#11358,#11359,#11360,#11361,#11362,#11363,#11364,#11365,#11366,#11367,#11368,
#11369,#11370,#11371,#11372,#11373,#11374,#11375,#11376,#11377,#11378,#11379,
#11380,#11381,#11382,#11383,#11384,#11385,#11386,#11387,#11388,#11389,#11390));
#11896=AXIS2_PLACEMENT_3D('',#16754,#13179,#13180);
#11897=AXIS2_PLACEMENT_3D('',#16755,#13181,#13182);
#11898=AXIS2_PLACEMENT_3D('',#16806,#13184,#13185);
#11899=AXIS2_PLACEMENT_3D('',#16807,#13186,#13187);
#11900=AXIS2_PLACEMENT_3D('',#16810,#13188,#13189);
#11901=AXIS2_PLACEMENT_3D('',#16811,#13190,#13191);
#11902=AXIS2_PLACEMENT_3D('',#16813,#13192,#13193);
#11903=AXIS2_PLACEMENT_3D('',#16814,#13194,#13195);
#11904=AXIS2_PLACEMENT_3D('',#16815,#13196,#13197);
#11905=AXIS2_PLACEMENT_3D('',#16818,#13198,#13199);
#11906=AXIS2_PLACEMENT_3D('',#16822,#13201,#13202);
#11907=AXIS2_PLACEMENT_3D('',#16824,#13204,#13205);
#11908=AXIS2_PLACEMENT_3D('',#16827,#13206,#13207);
#11909=AXIS2_PLACEMENT_3D('',#16829,#13208,#13209);
#11910=AXIS2_PLACEMENT_3D('',#16833,#13211,#13212);
#11911=AXIS2_PLACEMENT_3D('',#16835,#13214,#13215);
#11912=AXIS2_PLACEMENT_3D('',#16838,#13216,#13217);
#11913=AXIS2_PLACEMENT_3D('',#16842,#13219,#13220);
#11914=AXIS2_PLACEMENT_3D('',#16844,#13222,#13223);
#11915=AXIS2_PLACEMENT_3D('',#16847,#13224,#13225);
#11916=AXIS2_PLACEMENT_3D('',#16849,#13226,#13227);
#11917=AXIS2_PLACEMENT_3D('',#16850,#13228,#13229);
#11918=AXIS2_PLACEMENT_3D('',#16851,#13230,#13231);
#11919=AXIS2_PLACEMENT_3D('',#16854,#13232,#13233);
#11920=AXIS2_PLACEMENT_3D('',#16856,#13234,#13235);
#11921=AXIS2_PLACEMENT_3D('',#16857,#13236,#13237);
#11922=AXIS2_PLACEMENT_3D('',#16858,#13238,#13239);
#11923=AXIS2_PLACEMENT_3D('',#16861,#13240,#13241);
#11924=AXIS2_PLACEMENT_3D('',#16863,#13242,#13243);
#11925=AXIS2_PLACEMENT_3D('',#16864,#13244,#13245);
#11926=AXIS2_PLACEMENT_3D('',#16865,#13246,#13247);
#11927=AXIS2_PLACEMENT_3D('',#16868,#13248,#13249);
#11928=AXIS2_PLACEMENT_3D('',#16870,#13250,#13251);
#11929=AXIS2_PLACEMENT_3D('',#16871,#13252,#13253);
#11930=AXIS2_PLACEMENT_3D('',#16872,#13254,#13255);
#11931=AXIS2_PLACEMENT_3D('',#16874,#13256,#13257);
#11932=AXIS2_PLACEMENT_3D('',#16876,#13258,#13259);
#11933=AXIS2_PLACEMENT_3D('',#16878,#13260,#13261);
#11934=AXIS2_PLACEMENT_3D('',#16879,#13262,#13263);
#11935=AXIS2_PLACEMENT_3D('',#16880,#13264,#13265);
#11936=AXIS2_PLACEMENT_3D('',#16883,#13266,#13267);
#11937=AXIS2_PLACEMENT_3D('',#16884,#13268,#13269);
#11938=AXIS2_PLACEMENT_3D('',#16886,#13270,#13271);
#11939=AXIS2_PLACEMENT_3D('',#16887,#13272,#13273);
#11940=AXIS2_PLACEMENT_3D('',#16888,#13274,#13275);
#11941=AXIS2_PLACEMENT_3D('',#16890,#13276,#13277);
#11942=AXIS2_PLACEMENT_3D('',#16893,#13279,#13280);
#11943=AXIS2_PLACEMENT_3D('',#16894,#13281,#13282);
#11944=AXIS2_PLACEMENT_3D('',#16896,#13283,#13284);
#11945=AXIS2_PLACEMENT_3D('',#16898,#13286,#13287);
#11946=AXIS2_PLACEMENT_3D('',#16900,#13288,#13289);
#11947=AXIS2_PLACEMENT_3D('',#16903,#13291,#13292);
#11948=AXIS2_PLACEMENT_3D('',#16904,#13293,#13294);
#11949=AXIS2_PLACEMENT_3D('',#16906,#13295,#13296);
#11950=AXIS2_PLACEMENT_3D('',#16908,#13298,#13299);
#11951=AXIS2_PLACEMENT_3D('',#16910,#13300,#13301);
#11952=AXIS2_PLACEMENT_3D('',#16913,#13303,#13304);
#11953=AXIS2_PLACEMENT_3D('',#16914,#13305,#13306);
#11954=AXIS2_PLACEMENT_3D('',#16916,#13307,#13308);
#11955=AXIS2_PLACEMENT_3D('',#16918,#13310,#13311);
#11956=AXIS2_PLACEMENT_3D('',#16920,#13312,#13313);
#11957=AXIS2_PLACEMENT_3D('',#16923,#13315,#13316);
#11958=AXIS2_PLACEMENT_3D('',#16924,#13317,#13318);
#11959=AXIS2_PLACEMENT_3D('',#16926,#13319,#13320);
#11960=AXIS2_PLACEMENT_3D('',#16928,#13322,#13323);
#11961=AXIS2_PLACEMENT_3D('',#16930,#13324,#13325);
#11962=AXIS2_PLACEMENT_3D('',#16933,#13327,#13328);
#11963=AXIS2_PLACEMENT_3D('',#16934,#13329,#13330);
#11964=AXIS2_PLACEMENT_3D('',#16936,#13331,#13332);
#11965=AXIS2_PLACEMENT_3D('',#16938,#13334,#13335);
#11966=AXIS2_PLACEMENT_3D('',#16940,#13336,#13337);
#11967=AXIS2_PLACEMENT_3D('',#16943,#13339,#13340);
#11968=AXIS2_PLACEMENT_3D('',#16944,#13341,#13342);
#11969=AXIS2_PLACEMENT_3D('',#16946,#13343,#13344);
#11970=AXIS2_PLACEMENT_3D('',#16948,#13346,#13347);
#11971=AXIS2_PLACEMENT_3D('',#16950,#13349,#13350);
#11972=AXIS2_PLACEMENT_3D('',#16952,#13351,#13352);
#11973=AXIS2_PLACEMENT_3D('',#16955,#13354,#13355);
#11974=AXIS2_PLACEMENT_3D('',#16956,#13356,#13357);
#11975=AXIS2_PLACEMENT_3D('',#16959,#13358,#13359);
#11976=AXIS2_PLACEMENT_3D('',#16960,#13360,#13361);
#11977=AXIS2_PLACEMENT_3D('',#16963,#13363,#13364);
#11978=AXIS2_PLACEMENT_3D('',#16964,#13365,#13366);
#11979=AXIS2_PLACEMENT_3D('',#16966,#13368,#13369);
#11980=AXIS2_PLACEMENT_3D('',#16968,#13370,#13371);
#11981=AXIS2_PLACEMENT_3D('',#16971,#13373,#13374);
#11982=AXIS2_PLACEMENT_3D('',#16972,#13375,#13376);
#11983=AXIS2_PLACEMENT_3D('',#16974,#13377,#13378);
#11984=AXIS2_PLACEMENT_3D('',#16977,#13380,#13381);
#11985=AXIS2_PLACEMENT_3D('',#16978,#13382,#13383);
#11986=AXIS2_PLACEMENT_3D('',#16980,#13384,#13385);
#11987=AXIS2_PLACEMENT_3D('',#16983,#13387,#13388);
#11988=AXIS2_PLACEMENT_3D('',#16984,#13389,#13390);
#11989=AXIS2_PLACEMENT_3D('',#16986,#13391,#13392);
#11990=AXIS2_PLACEMENT_3D('',#16989,#13394,#13395);
#11991=AXIS2_PLACEMENT_3D('',#16990,#13396,#13397);
#11992=AXIS2_PLACEMENT_3D('',#16993,#13398,#13399);
#11993=AXIS2_PLACEMENT_3D('',#16997,#13401,#13402);
#11994=AXIS2_PLACEMENT_3D('',#16999,#13404,#13405);
#11995=AXIS2_PLACEMENT_3D('',#17001,#13406,#13407);
#11996=AXIS2_PLACEMENT_3D('',#17303,#13408,#13409);
#11997=AXIS2_PLACEMENT_3D('',#17353,#13411,#13412);
#11998=AXIS2_PLACEMENT_3D('',#17355,#13414,#13415);
#11999=AXIS2_PLACEMENT_3D('',#17358,#13416,#13417);
#12000=AXIS2_PLACEMENT_3D('',#17360,#13418,#13419);
#12001=AXIS2_PLACEMENT_3D('',#17364,#13421,#13422);
#12002=AXIS2_PLACEMENT_3D('',#17366,#13423,#13424);
#12003=AXIS2_PLACEMENT_3D('',#17368,#13426,#13427);
#12004=AXIS2_PLACEMENT_3D('',#17375,#13431,#13432);
#12005=AXIS2_PLACEMENT_3D('',#17424,#13433,#13434);
#12006=AXIS2_PLACEMENT_3D('',#17741,#13435,#13436);
#12007=AXIS2_PLACEMENT_3D('',#17789,#13437,#13438);
#12008=AXIS2_PLACEMENT_3D('',#17958,#13440,#13441);
#12009=AXIS2_PLACEMENT_3D('',#18046,#13442,#13443);
#12010=AXIS2_PLACEMENT_3D('',#18207,#13445,#13446);
#12011=AXIS2_PLACEMENT_3D('',#18291,#13447,#13448);
#12012=AXIS2_PLACEMENT_3D('',#18460,#13450,#13451);
#12013=AXIS2_PLACEMENT_3D('',#18462,#13452,#13453);
#12014=AXIS2_PLACEMENT_3D('',#18631,#13455,#13456);
#12015=AXIS2_PLACEMENT_3D('',#18634,#13458,#13459);
#12016=AXIS2_PLACEMENT_3D('',#18803,#13461,#13462);
#12017=AXIS2_PLACEMENT_3D('',#18893,#13464,#13465);
#12018=AXIS2_PLACEMENT_3D('',#19054,#13467,#13468);
#12019=AXIS2_PLACEMENT_3D('',#19139,#13470,#13471);
#12020=AXIS2_PLACEMENT_3D('',#19152,#13478,#13479);
#12021=AXIS2_PLACEMENT_3D('',#19166,#13486,#13487);
#12022=AXIS2_PLACEMENT_3D('',#19170,#13489,#13490);
#12023=AXIS2_PLACEMENT_3D('',#19176,#13494,#13495);
#12024=AXIS2_PLACEMENT_3D('',#19180,#13497,#13498);
#12025=AXIS2_PLACEMENT_3D('',#19185,#13502,#13503);
#12026=AXIS2_PLACEMENT_3D('',#19200,#13511,#13512);
#12027=AXIS2_PLACEMENT_3D('',#19204,#13514,#13515);
#12028=AXIS2_PLACEMENT_3D('',#19209,#13518,#13519);
#12029=AXIS2_PLACEMENT_3D('',#19212,#13521,#13522);
#12030=AXIS2_PLACEMENT_3D('',#19213,#13523,#13524);
#12031=AXIS2_PLACEMENT_3D('',#19214,#13525,#13526);
#12032=AXIS2_PLACEMENT_3D('',#19216,#13527,#13528);
#12033=AXIS2_PLACEMENT_3D('',#19218,#13529,#13530);
#12034=AXIS2_PLACEMENT_3D('',#19220,#13532,#13533);
#12035=AXIS2_PLACEMENT_3D('',#19223,#13534,#13535);
#12036=AXIS2_PLACEMENT_3D('',#19225,#13536,#13537);
#12037=AXIS2_PLACEMENT_3D('',#19227,#13538,#13539);
#12038=AXIS2_PLACEMENT_3D('',#19230,#13541,#13542);
#12039=AXIS2_PLACEMENT_3D('',#19231,#13543,#13544);
#12040=AXIS2_PLACEMENT_3D('',#19233,#13545,#13546);
#12041=AXIS2_PLACEMENT_3D('',#19235,#13547,#13548);
#12042=AXIS2_PLACEMENT_3D('',#19239,#13550,#13551);
#12043=AXIS2_PLACEMENT_3D('',#19240,#13552,#13553);
#12044=AXIS2_PLACEMENT_3D('',#19241,#13554,#13555);
#12045=AXIS2_PLACEMENT_3D('',#19244,#13556,#13557);
#12046=AXIS2_PLACEMENT_3D('',#19246,#13558,#13559);
#12047=AXIS2_PLACEMENT_3D('',#19248,#13560,#13561);
#12048=AXIS2_PLACEMENT_3D('',#19250,#13562,#13563);
#12049=AXIS2_PLACEMENT_3D('',#19252,#13565,#13566);
#12050=AXIS2_PLACEMENT_3D('',#19257,#13568,#13569);
#12051=AXIS2_PLACEMENT_3D('',#19261,#13571,#13572);
#12052=AXIS2_PLACEMENT_3D('',#19265,#13574,#13575);
#12053=AXIS2_PLACEMENT_3D('',#19268,#13577,#13578);
#12054=AXIS2_PLACEMENT_3D('',#19273,#13580,#13581);
#12055=AXIS2_PLACEMENT_3D('',#19277,#13583,#13584);
#12056=AXIS2_PLACEMENT_3D('',#19281,#13586,#13587);
#12057=AXIS2_PLACEMENT_3D('',#19284,#13589,#13590);
#12058=AXIS2_PLACEMENT_3D('',#19285,#13591,#13592);
#12059=AXIS2_PLACEMENT_3D('',#19287,#13593,#13594);
#12060=AXIS2_PLACEMENT_3D('',#19291,#13597,#13598);
#12061=AXIS2_PLACEMENT_3D('',#19292,#13599,#13600);
#12062=AXIS2_PLACEMENT_3D('',#19296,#13602,#13603);
#12063=AXIS2_PLACEMENT_3D('',#19300,#13606,#13607);
#12064=AXIS2_PLACEMENT_3D('',#19305,#13609,#13610);
#12065=AXIS2_PLACEMENT_3D('',#19308,#13613,#13614);
#12066=AXIS2_PLACEMENT_3D('',#19314,#13618,#13619);
#12067=AXIS2_PLACEMENT_3D('',#19329,#13620,#13621);
#12068=AXIS2_PLACEMENT_3D('',#19330,#13622,#13623);
#12069=AXIS2_PLACEMENT_3D('',#19331,#13624,#13625);
#12070=AXIS2_PLACEMENT_3D('',#19347,#13626,#13627);
#12071=AXIS2_PLACEMENT_3D('',#19349,#13628,#13629);
#12072=AXIS2_PLACEMENT_3D('',#19364,#13630,#13631);
#12073=AXIS2_PLACEMENT_3D('',#19365,#13632,#13633);
#12074=AXIS2_PLACEMENT_3D('',#19366,#13634,#13635);
#12075=AXIS2_PLACEMENT_3D('',#19381,#13636,#13637);
#12076=AXIS2_PLACEMENT_3D('',#19382,#13638,#13639);
#12077=AXIS2_PLACEMENT_3D('',#19383,#13640,#13641);
#12078=AXIS2_PLACEMENT_3D('',#19384,#13642,#13643);
#12079=AXIS2_PLACEMENT_3D('',#19397,#13644,#13645);
#12080=AXIS2_PLACEMENT_3D('',#19416,#13646,#13647);
#12081=AXIS2_PLACEMENT_3D('',#19417,#13648,#13649);
#12082=AXIS2_PLACEMENT_3D('',#19418,#13650,#13651);
#12083=AXIS2_PLACEMENT_3D('',#19419,#13652,#13653);
#12084=AXIS2_PLACEMENT_3D('',#19607,#13654,#13655);
#12085=AXIS2_PLACEMENT_3D('',#19608,#13656,#13657);
#12086=AXIS2_PLACEMENT_3D('',#19621,#13658,#13659);
#12087=AXIS2_PLACEMENT_3D('',#19640,#13660,#13661);
#12088=AXIS2_PLACEMENT_3D('',#19641,#13662,#13663);
#12089=AXIS2_PLACEMENT_3D('',#19642,#13664,#13665);
#12090=AXIS2_PLACEMENT_3D('',#19643,#13666,#13667);
#12091=AXIS2_PLACEMENT_3D('',#19831,#13668,#13669);
#12092=AXIS2_PLACEMENT_3D('',#19832,#13670,#13671);
#12093=AXIS2_PLACEMENT_3D('',#19833,#13672,#13673);
#12094=AXIS2_PLACEMENT_3D('',#19834,#13674,#13675);
#12095=AXIS2_PLACEMENT_3D('',#19847,#13676,#13677);
#12096=AXIS2_PLACEMENT_3D('',#19848,#13678,#13679);
#12097=AXIS2_PLACEMENT_3D('',#20009,#13680,#13681);
#12098=AXIS2_PLACEMENT_3D('',#20010,#13682,#13683);
#12099=AXIS2_PLACEMENT_3D('',#20011,#13684,#13685);
#12100=AXIS2_PLACEMENT_3D('',#20012,#13686,#13687);
#12101=AXIS2_PLACEMENT_3D('',#20025,#13688,#13689);
#12102=AXIS2_PLACEMENT_3D('',#20026,#13690,#13691);
#12103=AXIS2_PLACEMENT_3D('',#20322,#13692,#13693);
#12104=AXIS2_PLACEMENT_3D('',#20323,#13694,#13695);
#12105=AXIS2_PLACEMENT_3D('',#20324,#13696,#13697);
#12106=AXIS2_PLACEMENT_3D('',#20595,#13698,#13699);
#12107=AXIS2_PLACEMENT_3D('',#20596,#13700,#13701);
#12108=AXIS2_PLACEMENT_3D('',#20597,#13702,#13703);
#12109=AXIS2_PLACEMENT_3D('',#20724,#13704,#13705);
#12110=AXIS2_PLACEMENT_3D('',#20725,#13706,#13707);
#12111=AXIS2_PLACEMENT_3D('',#20726,#13708,#13709);
#12112=AXIS2_PLACEMENT_3D('',#20728,#13710,#13711);
#12113=AXIS2_PLACEMENT_3D('',#20731,#13713,#13714);
#12114=AXIS2_PLACEMENT_3D('',#20732,#13715,#13716);
#12115=AXIS2_PLACEMENT_3D('',#20735,#13717,#13718);
#12116=AXIS2_PLACEMENT_3D('',#20737,#13719,#13720);
#12117=AXIS2_PLACEMENT_3D('',#20741,#13722,#13723);
#12118=AXIS2_PLACEMENT_3D('',#20742,#13724,#13725);
#12119=AXIS2_PLACEMENT_3D('',#20743,#13726,#13727);
#12120=AXIS2_PLACEMENT_3D('',#20745,#13728,#13729);
#12121=AXIS2_PLACEMENT_3D('',#20747,#13730,#13731);
#12122=AXIS2_PLACEMENT_3D('',#20751,#13733,#13734);
#12123=AXIS2_PLACEMENT_3D('',#20752,#13735,#13736);
#12124=AXIS2_PLACEMENT_3D('',#20753,#13737,#13738);
#12125=AXIS2_PLACEMENT_3D('',#20756,#13739,#13740);
#12126=AXIS2_PLACEMENT_3D('',#20760,#13742,#13743);
#12127=AXIS2_PLACEMENT_3D('',#20762,#13744,#13745);
#12128=AXIS2_PLACEMENT_3D('',#20763,#13746,#13747);
#12129=AXIS2_PLACEMENT_3D('',#20764,#13748,#13749);
#12130=AXIS2_PLACEMENT_3D('',#20766,#13750,#13751);
#12131=AXIS2_PLACEMENT_3D('',#20770,#13754,#13755);
#12132=AXIS2_PLACEMENT_3D('',#20771,#13756,#13757);
#12133=AXIS2_PLACEMENT_3D('',#20778,#13761,#13762);
#12134=AXIS2_PLACEMENT_3D('',#20779,#13763,#13764);
#12135=AXIS2_PLACEMENT_3D('',#20786,#13768,#13769);
#12136=AXIS2_PLACEMENT_3D('',#20787,#13770,#13771);
#12137=AXIS2_PLACEMENT_3D('',#20793,#13775,#13776);
#12138=AXIS2_PLACEMENT_3D('',#20795,#13777,#13778);
#12139=AXIS2_PLACEMENT_3D('',#20796,#13779,#13780);
#12140=AXIS2_PLACEMENT_3D('',#20807,#13781,#13782);
#12141=AXIS2_PLACEMENT_3D('',#20820,#13783,#13784);
#12142=AXIS2_PLACEMENT_3D('',#20822,#13785,#13786);
#12143=AXIS2_PLACEMENT_3D('',#20834,#13787,#13788);
#12144=AXIS2_PLACEMENT_3D('',#20835,#13789,#13790);
#12145=AXIS2_PLACEMENT_3D('',#20836,#13791,#13792);
#12146=AXIS2_PLACEMENT_3D('',#20838,#13793,#13794);
#12147=AXIS2_PLACEMENT_3D('',#20839,#13795,#13796);
#12148=AXIS2_PLACEMENT_3D('',#20850,#13797,#13798);
#12149=AXIS2_PLACEMENT_3D('',#20851,#13799,#13800);
#12150=AXIS2_PLACEMENT_3D('',#20864,#13801,#13802);
#12151=AXIS2_PLACEMENT_3D('',#20883,#13803,#13804);
#12152=AXIS2_PLACEMENT_3D('',#20884,#13805,#13806);
#12153=AXIS2_PLACEMENT_3D('',#20885,#13807,#13808);
#12154=AXIS2_PLACEMENT_3D('',#20886,#13809,#13810);
#12155=AXIS2_PLACEMENT_3D('',#21101,#13811,#13812);
#12156=AXIS2_PLACEMENT_3D('',#21102,#13813,#13814);
#12157=AXIS2_PLACEMENT_3D('',#21115,#13815,#13816);
#12158=AXIS2_PLACEMENT_3D('',#21134,#13817,#13818);
#12159=AXIS2_PLACEMENT_3D('',#21135,#13819,#13820);
#12160=AXIS2_PLACEMENT_3D('',#21136,#13821,#13822);
#12161=AXIS2_PLACEMENT_3D('',#21137,#13823,#13824);
#12162=AXIS2_PLACEMENT_3D('',#21358,#13825,#13826);
#12163=AXIS2_PLACEMENT_3D('',#21359,#13827,#13828);
#12164=AXIS2_PLACEMENT_3D('',#21360,#13829,#13830);
#12165=AXIS2_PLACEMENT_3D('',#21361,#13831,#13832);
#12166=AXIS2_PLACEMENT_3D('',#21374,#13833,#13834);
#12167=AXIS2_PLACEMENT_3D('',#21375,#13835,#13836);
#12168=AXIS2_PLACEMENT_3D('',#21536,#13837,#13838);
#12169=AXIS2_PLACEMENT_3D('',#21537,#13839,#13840);
#12170=AXIS2_PLACEMENT_3D('',#21538,#13841,#13842);
#12171=AXIS2_PLACEMENT_3D('',#21539,#13843,#13844);
#12172=AXIS2_PLACEMENT_3D('',#21552,#13845,#13846);
#12173=AXIS2_PLACEMENT_3D('',#21553,#13847,#13848);
#12174=AXIS2_PLACEMENT_3D('',#21837,#13849,#13850);
#12175=AXIS2_PLACEMENT_3D('',#21838,#13851,#13852);
#12176=AXIS2_PLACEMENT_3D('',#21839,#13853,#13854);
#12177=AXIS2_PLACEMENT_3D('',#22122,#13855,#13856);
#12178=AXIS2_PLACEMENT_3D('',#22123,#13857,#13858);
#12179=AXIS2_PLACEMENT_3D('',#22124,#13859,#13860);
#12180=AXIS2_PLACEMENT_3D('',#22251,#13861,#13862);
#12181=AXIS2_PLACEMENT_3D('',#22260,#13867,#13868);
#12182=AXIS2_PLACEMENT_3D('',#22273,#13875,#13876);
#12183=AXIS2_PLACEMENT_3D('',#22281,#13880,#13881);
#12184=AXIS2_PLACEMENT_3D('',#22282,#13882,#13883);
#12185=AXIS2_PLACEMENT_3D('',#22287,#13885,#13886);
#12186=AXIS2_PLACEMENT_3D('',#22291,#13889,#13890);
#12187=AXIS2_PLACEMENT_3D('',#22300,#13895,#13896);
#12188=AXIS2_PLACEMENT_3D('',#22305,#13898,#13899);
#12189=AXIS2_PLACEMENT_3D('',#22307,#13901,#13902);
#12190=AXIS2_PLACEMENT_3D('',#22312,#13904,#13905);
#12191=AXIS2_PLACEMENT_3D('',#22314,#13907,#13908);
#12192=AXIS2_PLACEMENT_3D('',#22323,#13913,#13914);
#12193=AXIS2_PLACEMENT_3D('',#22328,#13916,#13917);
#12194=AXIS2_PLACEMENT_3D('',#22330,#13919,#13920);
#12195=AXIS2_PLACEMENT_3D('',#22335,#13922,#13923);
#12196=AXIS2_PLACEMENT_3D('',#22337,#13925,#13926);
#12197=AXIS2_PLACEMENT_3D('',#22346,#13931,#13932);
#12198=AXIS2_PLACEMENT_3D('',#22353,#13935,#13936);
#12199=AXIS2_PLACEMENT_3D('',#22355,#13938,#13939);
#12200=AXIS2_PLACEMENT_3D('',#22360,#13941,#13942);
#12201=AXIS2_PLACEMENT_3D('',#22364,#13945,#13946);
#12202=AXIS2_PLACEMENT_3D('',#22373,#13951,#13952);
#12203=AXIS2_PLACEMENT_3D('',#22377,#13954,#13955);
#12204=AXIS2_PLACEMENT_3D('',#22379,#13957,#13958);
#12205=AXIS2_PLACEMENT_3D('',#22383,#13960,#13961);
#12206=AXIS2_PLACEMENT_3D('',#22385,#13963,#13964);
#12207=AXIS2_PLACEMENT_3D('',#22394,#13969,#13970);
#12208=AXIS2_PLACEMENT_3D('',#22398,#13972,#13973);
#12209=AXIS2_PLACEMENT_3D('',#22400,#13975,#13976);
#12210=AXIS2_PLACEMENT_3D('',#22404,#13978,#13979);
#12211=AXIS2_PLACEMENT_3D('',#22406,#13981,#13982);
#12212=AXIS2_PLACEMENT_3D('',#22415,#13987,#13988);
#12213=AXIS2_PLACEMENT_3D('',#22424,#13993,#13994);
#12214=AXIS2_PLACEMENT_3D('',#22433,#13999,#14000);
#12215=AXIS2_PLACEMENT_3D('',#22442,#14005,#14006);
#12216=AXIS2_PLACEMENT_3D('',#22443,#14007,#14008);
#12217=AXIS2_PLACEMENT_3D('',#22444,#14009,#14010);
#12218=AXIS2_PLACEMENT_3D('',#22445,#14011,#14012);
#12219=AXIS2_PLACEMENT_3D('',#22446,#14013,#14014);
#12220=AXIS2_PLACEMENT_3D('',#22553,#14015,#14016);
#12221=AXIS2_PLACEMENT_3D('',#22554,#14017,#14018);
#12222=AXIS2_PLACEMENT_3D('',#22555,#14019,#14020);
#12223=AXIS2_PLACEMENT_3D('',#22556,#14021,#14022);
#12224=AXIS2_PLACEMENT_3D('',#22557,#14023,#14024);
#12225=AXIS2_PLACEMENT_3D('',#22558,#14025,#14026);
#12226=AXIS2_PLACEMENT_3D('',#22559,#14027,#14028);
#12227=AXIS2_PLACEMENT_3D('',#22560,#14029,#14030);
#12228=AXIS2_PLACEMENT_3D('',#22561,#14031,#14032);
#12229=AXIS2_PLACEMENT_3D('',#22562,#14033,#14034);
#12230=AXIS2_PLACEMENT_3D('',#22563,#14035,#14036);
#12231=AXIS2_PLACEMENT_3D('',#22564,#14037,#14038);
#12232=AXIS2_PLACEMENT_3D('',#22565,#14039,#14040);
#12233=AXIS2_PLACEMENT_3D('',#22626,#14041,#14042);
#12234=AXIS2_PLACEMENT_3D('',#22627,#14043,#14044);
#12235=AXIS2_PLACEMENT_3D('',#22628,#14045,#14046);
#12236=AXIS2_PLACEMENT_3D('',#22629,#14047,#14048);
#12237=AXIS2_PLACEMENT_3D('',#22733,#14049,#14050);
#12238=AXIS2_PLACEMENT_3D('',#22734,#14051,#14052);
#12239=AXIS2_PLACEMENT_3D('',#22735,#14053,#14054);
#12240=AXIS2_PLACEMENT_3D('',#22736,#14055,#14056);
#12241=AXIS2_PLACEMENT_3D('',#22737,#14057,#14058);
#12242=AXIS2_PLACEMENT_3D('',#22738,#14059,#14060);
#12243=AXIS2_PLACEMENT_3D('',#22739,#14061,#14062);
#12244=AXIS2_PLACEMENT_3D('',#22740,#14063,#14064);
#12245=AXIS2_PLACEMENT_3D('',#22741,#14065,#14066);
#12246=AXIS2_PLACEMENT_3D('',#22742,#14067,#14068);
#12247=AXIS2_PLACEMENT_3D('',#22743,#14069,#14070);
#12248=AXIS2_PLACEMENT_3D('',#22744,#14071,#14072);
#12249=AXIS2_PLACEMENT_3D('',#22745,#14073,#14074);
#12250=AXIS2_PLACEMENT_3D('',#22861,#14075,#14076);
#12251=AXIS2_PLACEMENT_3D('',#22862,#14077,#14078);
#12252=AXIS2_PLACEMENT_3D('',#22863,#14079,#14080);
#12253=AXIS2_PLACEMENT_3D('',#22930,#14081,#14082);
#12254=AXIS2_PLACEMENT_3D('',#22931,#14083,#14084);
#12255=AXIS2_PLACEMENT_3D('',#22932,#14085,#14086);
#12256=AXIS2_PLACEMENT_3D('',#22933,#14087,#14088);
#12257=AXIS2_PLACEMENT_3D('',#22934,#14089,#14090);
#12258=AXIS2_PLACEMENT_3D('',#22935,#14091,#14092);
#12259=AXIS2_PLACEMENT_3D('',#22936,#14093,#14094);
#12260=AXIS2_PLACEMENT_3D('',#22937,#14095,#14096);
#12261=AXIS2_PLACEMENT_3D('',#22938,#14097,#14098);
#12262=AXIS2_PLACEMENT_3D('',#22939,#14099,#14100);
#12263=AXIS2_PLACEMENT_3D('',#23006,#14101,#14102);
#12264=AXIS2_PLACEMENT_3D('',#23007,#14103,#14104);
#12265=AXIS2_PLACEMENT_3D('',#23008,#14105,#14106);
#12266=AXIS2_PLACEMENT_3D('',#23009,#14107,#14108);
#12267=AXIS2_PLACEMENT_3D('',#23028,#14109,#14110);
#12268=AXIS2_PLACEMENT_3D('',#23029,#14111,#14112);
#12269=AXIS2_PLACEMENT_3D('',#23030,#14113,#14114);
#12270=AXIS2_PLACEMENT_3D('',#23031,#14115,#14116);
#12271=AXIS2_PLACEMENT_3D('',#23032,#14117,#14118);
#12272=AXIS2_PLACEMENT_3D('',#23033,#14119,#14120);
#12273=AXIS2_PLACEMENT_3D('',#23034,#14121,#14122);
#12274=AXIS2_PLACEMENT_3D('',#23035,#14123,#14124);
#12275=AXIS2_PLACEMENT_3D('',#23096,#14125,#14126);
#12276=AXIS2_PLACEMENT_3D('',#23097,#14127,#14128);
#12277=AXIS2_PLACEMENT_3D('',#23098,#14129,#14130);
#12278=AXIS2_PLACEMENT_3D('',#23099,#14131,#14132);
#12279=AXIS2_PLACEMENT_3D('',#23100,#14133,#14134);
#12280=AXIS2_PLACEMENT_3D('',#23101,#14135,#14136);
#12281=AXIS2_PLACEMENT_3D('',#23102,#14137,#14138);
#12282=AXIS2_PLACEMENT_3D('',#23103,#14139,#14140);
#12283=AXIS2_PLACEMENT_3D('',#23104,#14141,#14142);
#12284=AXIS2_PLACEMENT_3D('',#23211,#14143,#14144);
#12285=AXIS2_PLACEMENT_3D('',#23212,#14145,#14146);
#12286=AXIS2_PLACEMENT_3D('',#23213,#14147,#14148);
#12287=AXIS2_PLACEMENT_3D('',#23214,#14149,#14150);
#12288=AXIS2_PLACEMENT_3D('',#23215,#14151,#14152);
#12289=AXIS2_PLACEMENT_3D('',#23216,#14153,#14154);
#12290=AXIS2_PLACEMENT_3D('',#23217,#14155,#14156);
#12291=AXIS2_PLACEMENT_3D('',#23278,#14157,#14158);
#12292=AXIS2_PLACEMENT_3D('',#23279,#14159,#14160);
#12293=AXIS2_PLACEMENT_3D('',#23280,#14161,#14162);
#12294=AXIS2_PLACEMENT_3D('',#23281,#14163,#14164);
#12295=AXIS2_PLACEMENT_3D('',#23282,#14165,#14166);
#12296=AXIS2_PLACEMENT_3D('',#23283,#14167,#14168);
#12297=AXIS2_PLACEMENT_3D('',#23284,#14169,#14170);
#12298=AXIS2_PLACEMENT_3D('',#23285,#14171,#14172);
#12299=AXIS2_PLACEMENT_3D('',#23286,#14173,#14174);
#12300=AXIS2_PLACEMENT_3D('',#23384,#14175,#14176);
#12301=AXIS2_PLACEMENT_3D('',#23385,#14177,#14178);
#12302=AXIS2_PLACEMENT_3D('',#23386,#14179,#14180);
#12303=AXIS2_PLACEMENT_3D('',#23493,#14181,#14182);
#12304=AXIS2_PLACEMENT_3D('',#23494,#14183,#14184);
#12305=AXIS2_PLACEMENT_3D('',#23567,#14185,#14186);
#12306=AXIS2_PLACEMENT_3D('',#23568,#14187,#14188);
#12307=AXIS2_PLACEMENT_3D('',#23569,#14189,#14190);
#12308=AXIS2_PLACEMENT_3D('',#23570,#14191,#14192);
#12309=AXIS2_PLACEMENT_3D('',#23631,#14193,#14194);
#12310=AXIS2_PLACEMENT_3D('',#23632,#14195,#14196);
#12311=AXIS2_PLACEMENT_3D('',#23633,#14197,#14198);
#12312=AXIS2_PLACEMENT_3D('',#23634,#14199,#14200);
#12313=AXIS2_PLACEMENT_3D('',#23750,#14201,#14202);
#12314=AXIS2_PLACEMENT_3D('',#23751,#14203,#14204);
#12315=AXIS2_PLACEMENT_3D('',#23818,#14205,#14206);
#12316=AXIS2_PLACEMENT_3D('',#23819,#14207,#14208);
#12317=AXIS2_PLACEMENT_3D('',#23820,#14209,#14210);
#12318=AXIS2_PLACEMENT_3D('',#23821,#14211,#14212);
#12319=AXIS2_PLACEMENT_3D('',#23822,#14213,#14214);
#12320=AXIS2_PLACEMENT_3D('',#23823,#14215,#14216);
#12321=AXIS2_PLACEMENT_3D('',#23824,#14217,#14218);
#12322=AXIS2_PLACEMENT_3D('',#23825,#14219,#14220);
#12323=AXIS2_PLACEMENT_3D('',#23826,#14221,#14222);
#12324=AXIS2_PLACEMENT_3D('',#23827,#14223,#14224);
#12325=AXIS2_PLACEMENT_3D('',#23828,#14225,#14226);
#12326=AXIS2_PLACEMENT_3D('',#23829,#14227,#14228);
#12327=AXIS2_PLACEMENT_3D('',#23830,#14229,#14230);
#12328=AXIS2_PLACEMENT_3D('',#23831,#14231,#14232);
#12329=AXIS2_PLACEMENT_3D('',#23832,#14233,#14234);
#12330=AXIS2_PLACEMENT_3D('',#23833,#14235,#14236);
#12331=AXIS2_PLACEMENT_3D('',#23834,#14237,#14238);
#12332=AXIS2_PLACEMENT_3D('',#23835,#14239,#14240);
#12333=AXIS2_PLACEMENT_3D('',#23836,#14241,#14242);
#12334=AXIS2_PLACEMENT_3D('',#23837,#14243,#14244);
#12335=AXIS2_PLACEMENT_3D('',#23838,#14245,#14246);
#12336=AXIS2_PLACEMENT_3D('',#23839,#14247,#14248);
#12337=AXIS2_PLACEMENT_3D('',#23840,#14249,#14250);
#12338=AXIS2_PLACEMENT_3D('',#23841,#14251,#14252);
#12339=AXIS2_PLACEMENT_3D('',#23842,#14253,#14254);
#12340=AXIS2_PLACEMENT_3D('',#23843,#14255,#14256);
#12341=AXIS2_PLACEMENT_3D('',#23844,#14257,#14258);
#12342=AXIS2_PLACEMENT_3D('',#23845,#14259,#14260);
#12343=AXIS2_PLACEMENT_3D('',#23943,#14261,#14262);
#12344=AXIS2_PLACEMENT_3D('',#23944,#14263,#14264);
#12345=AXIS2_PLACEMENT_3D('',#23945,#14265,#14266);
#12346=AXIS2_PLACEMENT_3D('',#23946,#14267,#14268);
#12347=AXIS2_PLACEMENT_3D('',#23947,#14269,#14270);
#12348=AXIS2_PLACEMENT_3D('',#23948,#14271,#14272);
#12349=AXIS2_PLACEMENT_3D('',#23949,#14273,#14274);
#12350=AXIS2_PLACEMENT_3D('',#24056,#14275,#14276);
#12351=AXIS2_PLACEMENT_3D('',#24057,#14277,#14278);
#12352=AXIS2_PLACEMENT_3D('',#24058,#14279,#14280);
#12353=AXIS2_PLACEMENT_3D('',#24131,#14281,#14282);
#12354=AXIS2_PLACEMENT_3D('',#24132,#14283,#14284);
#12355=AXIS2_PLACEMENT_3D('',#24133,#14285,#14286);
#12356=AXIS2_PLACEMENT_3D('',#24134,#14287,#14288);
#12357=AXIS2_PLACEMENT_3D('',#24135,#14289,#14290);
#12358=AXIS2_PLACEMENT_3D('',#24196,#14291,#14292);
#12359=AXIS2_PLACEMENT_3D('',#24197,#14293,#14294);
#12360=AXIS2_PLACEMENT_3D('',#24198,#14295,#14296);
#12361=AXIS2_PLACEMENT_3D('',#24199,#14297,#14298);
#12362=AXIS2_PLACEMENT_3D('',#24200,#14299,#14300);
#12363=AXIS2_PLACEMENT_3D('',#24201,#14301,#14302);
#12364=AXIS2_PLACEMENT_3D('',#24220,#14303,#14304);
#12365=AXIS2_PLACEMENT_3D('',#24221,#14305,#14306);
#12366=AXIS2_PLACEMENT_3D('',#24222,#14307,#14308);
#12367=AXIS2_PLACEMENT_3D('',#24223,#14309,#14310);
#12368=AXIS2_PLACEMENT_3D('',#24224,#14311,#14312);
#12369=AXIS2_PLACEMENT_3D('',#24225,#14313,#14314);
#12370=AXIS2_PLACEMENT_3D('',#24226,#14315,#14316);
#12371=AXIS2_PLACEMENT_3D('',#24287,#14317,#14318);
#12372=AXIS2_PLACEMENT_3D('',#24288,#14319,#14320);
#12373=AXIS2_PLACEMENT_3D('',#24289,#14321,#14322);
#12374=AXIS2_PLACEMENT_3D('',#24290,#14323,#14324);
#12375=AXIS2_PLACEMENT_3D('',#24291,#14325,#14326);
#12376=AXIS2_PLACEMENT_3D('',#24407,#14327,#14328);
#12377=AXIS2_PLACEMENT_3D('',#24408,#14329,#14330);
#12378=AXIS2_PLACEMENT_3D('',#24409,#14331,#14332);
#12379=AXIS2_PLACEMENT_3D('',#24513,#14333,#14334);
#12380=AXIS2_PLACEMENT_3D('',#24514,#14335,#14336);
#12381=AXIS2_PLACEMENT_3D('',#24581,#14337,#14338);
#12382=AXIS2_PLACEMENT_3D('',#24582,#14339,#14340);
#12383=AXIS2_PLACEMENT_3D('',#24583,#14341,#14342);
#12384=AXIS2_PLACEMENT_3D('',#24650,#14343,#14344);
#12385=AXIS2_PLACEMENT_3D('',#24651,#14345,#14346);
#12386=AXIS2_PLACEMENT_3D('',#24652,#14347,#14348);
#12387=AXIS2_PLACEMENT_3D('',#24653,#14349,#14350);
#12388=AXIS2_PLACEMENT_3D('',#24760,#14351,#14352);
#12389=AXIS2_PLACEMENT_3D('',#24761,#14353,#14354);
#12390=AXIS2_PLACEMENT_3D('',#24762,#14355,#14356);
#12391=AXIS2_PLACEMENT_3D('',#24763,#14357,#14358);
#12392=AXIS2_PLACEMENT_3D('',#24764,#14359,#14360);
#12393=AXIS2_PLACEMENT_3D('',#24825,#14361,#14362);
#12394=AXIS2_PLACEMENT_3D('',#24826,#14363,#14364);
#12395=AXIS2_PLACEMENT_3D('',#24827,#14365,#14366);
#12396=AXIS2_PLACEMENT_3D('',#24828,#14367,#14368);
#12397=AXIS2_PLACEMENT_3D('',#24829,#14369,#14370);
#12398=AXIS2_PLACEMENT_3D('',#24830,#14371,#14372);
#12399=AXIS2_PLACEMENT_3D('',#24831,#14373,#14374);
#12400=AXIS2_PLACEMENT_3D('',#24832,#14375,#14376);
#12401=AXIS2_PLACEMENT_3D('',#24833,#14377,#14378);
#12402=AXIS2_PLACEMENT_3D('',#24834,#14379,#14380);
#12403=AXIS2_PLACEMENT_3D('',#24835,#14381,#14382);
#12404=AXIS2_PLACEMENT_3D('',#24836,#14383,#14384);
#12405=AXIS2_PLACEMENT_3D('',#24837,#14385,#14386);
#12406=AXIS2_PLACEMENT_3D('',#24838,#14387,#14388);
#12407=AXIS2_PLACEMENT_3D('',#24839,#14389,#14390);
#12408=AXIS2_PLACEMENT_3D('',#24946,#14391,#14392);
#12409=AXIS2_PLACEMENT_3D('',#24947,#14393,#14394);
#12410=AXIS2_PLACEMENT_3D('',#24948,#14395,#14396);
#12411=AXIS2_PLACEMENT_3D('',#24949,#14397,#14398);
#12412=AXIS2_PLACEMENT_3D('',#24950,#14399,#14400);
#12413=AXIS2_PLACEMENT_3D('',#24951,#14401,#14402);
#12414=AXIS2_PLACEMENT_3D('',#25012,#14403,#14404);
#12415=AXIS2_PLACEMENT_3D('',#25013,#14405,#14406);
#12416=AXIS2_PLACEMENT_3D('',#25014,#14407,#14408);
#12417=AXIS2_PLACEMENT_3D('',#25015,#14409,#14410);
#12418=AXIS2_PLACEMENT_3D('',#25131,#14411,#14412);
#12419=AXIS2_PLACEMENT_3D('',#25132,#14413,#14414);
#12420=AXIS2_PLACEMENT_3D('',#25133,#14415,#14416);
#12421=AXIS2_PLACEMENT_3D('',#25134,#14417,#14418);
#12422=AXIS2_PLACEMENT_3D('',#25201,#14419,#14420);
#12423=AXIS2_PLACEMENT_3D('',#25202,#14421,#14422);
#13179=DIRECTION('axis',(0.,0.,1.));
#13180=DIRECTION('refdir',(1.,0.,0.));
#13181=DIRECTION('center_axis',(0.,0.,-1.));
#13182=DIRECTION('ref_axis',(-1.,0.,0.));
#13183=DIRECTION('',(0.,0.,-1.));
#13184=DIRECTION('center_axis',(0.,0.,1.));
#13185=DIRECTION('ref_axis',(1.,0.,0.));
#13186=DIRECTION('center_axis',(0.,0.,1.));
#13187=DIRECTION('ref_axis',(1.,0.,0.));
#13188=DIRECTION('center_axis',(0.,0.,1.));
#13189=DIRECTION('ref_axis',(1.,0.,0.));
#13190=DIRECTION('center_axis',(0.,0.,1.));
#13191=DIRECTION('ref_axis',(1.,0.,0.));
#13192=DIRECTION('center_axis',(1.22464679914735E-16,-1.,0.));
#13193=DIRECTION('ref_axis',(-1.,-1.22464679914735E-16,0.));
#13194=DIRECTION('center_axis',(0.,0.,-1.));
#13195=DIRECTION('ref_axis',(1.,0.,0.));
#13196=DIRECTION('center_axis',(0.,0.,-1.));
#13197=DIRECTION('ref_axis',(-1.,0.,0.));
#13198=DIRECTION('center_axis',(0.,0.,-1.));
#13199=DIRECTION('ref_axis',(-1.,0.,0.));
#13200=DIRECTION('',(0.,0.,1.));
#13201=DIRECTION('center_axis',(-5.59912692738561E-15,-5.55111512312578E-15,
-1.));
#13202=DIRECTION('ref_axis',(1.,-2.66519052715287E-31,-5.59912692738561E-15));
#13203=DIRECTION('',(0.,0.,-1.));
#13204=DIRECTION('center_axis',(0.,0.,-1.));
#13205=DIRECTION('ref_axis',(-1.,0.,0.));
#13206=DIRECTION('center_axis',(0.,0.,1.));
#13207=DIRECTION('ref_axis',(-1.,0.,0.));
#13208=DIRECTION('center_axis',(0.,0.,1.));
#13209=DIRECTION('ref_axis',(-1.,0.,0.));
#13210=DIRECTION('',(0.,0.,1.));
#13211=DIRECTION('center_axis',(0.,0.,1.));
#13212=DIRECTION('ref_axis',(1.,0.,0.));
#13213=DIRECTION('',(0.,0.,-1.));
#13214=DIRECTION('center_axis',(0.,0.,-1.));
#13215=DIRECTION('ref_axis',(-1.,0.,0.));
#13216=DIRECTION('center_axis',(0.,0.,-1.));
#13217=DIRECTION('ref_axis',(-1.,0.,0.));
#13218=DIRECTION('',(0.,0.,1.));
#13219=DIRECTION('center_axis',(0.,0.,-1.));
#13220=DIRECTION('ref_axis',(1.,0.,0.));
#13221=DIRECTION('',(0.,0.,-1.));
#13222=DIRECTION('center_axis',(0.,1.,0.));
#13223=DIRECTION('ref_axis',(1.,0.,0.));
#13224=DIRECTION('center_axis',(0.710144927536232,-0.704055524724123,-3.94209624685744E-15));
#13225=DIRECTION('ref_axis',(-0.704055524724123,-0.710144927536232,-5.14874778252965E-31));
#13226=DIRECTION('center_axis',(-1.,-5.55111512312578E-15,0.));
#13227=DIRECTION('ref_axis',(5.55111512312578E-15,-1.,0.));
#13228=DIRECTION('center_axis',(0.,0.,1.));
#13229=DIRECTION('ref_axis',(1.,0.,0.));
#13230=DIRECTION('center_axis',(0.,1.,0.));
#13231=DIRECTION('ref_axis',(1.,0.,0.));
#13232=DIRECTION('center_axis',(0.,0.,-1.));
#13233=DIRECTION('ref_axis',(-1.,0.,0.));
#13234=DIRECTION('center_axis',(-1.,0.,-5.55111512312578E-15));
#13235=DIRECTION('ref_axis',(-5.55111512312578E-15,0.,1.));
#13236=DIRECTION('center_axis',(0.710144927536229,-0.704055524724125,0.));
#13237=DIRECTION('ref_axis',(-0.704055524724125,-0.710144927536229,0.));
#13238=DIRECTION('center_axis',(0.,1.,0.));
#13239=DIRECTION('ref_axis',(1.,0.,0.));
#13240=DIRECTION('center_axis',(-0.710144927536232,0.704055524724123,3.94209624685746E-15));
#13241=DIRECTION('ref_axis',(-0.704055524724123,-0.710144927536232,2.54343028847643E-31));
#13242=DIRECTION('center_axis',(-1.,-5.55111512312578E-15,0.));
#13243=DIRECTION('ref_axis',(5.55111512312578E-15,-1.,0.));
#13244=DIRECTION('center_axis',(-7.88448485693075E-15,0.,-1.));
#13245=DIRECTION('ref_axis',(1.,0.,-7.88448485693075E-15));
#13246=DIRECTION('center_axis',(0.,1.,0.));
#13247=DIRECTION('ref_axis',(1.,0.,0.));
#13248=DIRECTION('center_axis',(0.,0.,1.));
#13249=DIRECTION('ref_axis',(-1.,0.,0.));
#13250=DIRECTION('center_axis',(-1.,0.,-5.55111512312578E-15));
#13251=DIRECTION('ref_axis',(-5.55111512312578E-15,0.,1.));
#13252=DIRECTION('center_axis',(-0.710144927536229,0.704055524724125,0.));
#13253=DIRECTION('ref_axis',(-0.704055524724125,-0.710144927536229,0.));
#13254=DIRECTION('center_axis',(0.,0.,1.));
#13255=DIRECTION('ref_axis',(1.,0.,0.));
#13256=DIRECTION('center_axis',(0.,0.,1.));
#13257=DIRECTION('ref_axis',(1.,0.,0.));
#13258=DIRECTION('center_axis',(1.22464679914735E-16,-1.,0.));
#13259=DIRECTION('ref_axis',(-1.,-1.22464679914735E-16,0.));
#13260=DIRECTION('center_axis',(0.,0.,-1.));
#13261=DIRECTION('ref_axis',(1.,0.,0.));
#13262=DIRECTION('center_axis',(0.,0.,-1.));
#13263=DIRECTION('ref_axis',(1.,0.,0.));
#13264=DIRECTION('center_axis',(0.,0.,1.));
#13265=DIRECTION('ref_axis',(1.,0.,0.));
#13266=DIRECTION('center_axis',(0.,0.,1.));
#13267=DIRECTION('ref_axis',(1.,0.,0.));
#13268=DIRECTION('center_axis',(0.,0.,1.));
#13269=DIRECTION('ref_axis',(1.,0.,0.));
#13270=DIRECTION('center_axis',(1.22464679914735E-16,-1.,0.));
#13271=DIRECTION('ref_axis',(-1.,-1.22464679914735E-16,0.));
#13272=DIRECTION('center_axis',(0.,0.,-1.));
#13273=DIRECTION('ref_axis',(1.,0.,0.));
#13274=DIRECTION('center_axis',(0.,0.,1.));
#13275=DIRECTION('ref_axis',(1.,0.,0.));
#13276=DIRECTION('center_axis',(0.,0.,1.));
#13277=DIRECTION('ref_axis',(1.,0.,0.));
#13278=DIRECTION('',(-0.707106781186566,-8.65956056235516E-17,0.707106781186529));
#13279=DIRECTION('center_axis',(0.,0.,1.));
#13280=DIRECTION('ref_axis',(1.,0.,0.));
#13281=DIRECTION('center_axis',(0.,0.,1.));
#13282=DIRECTION('ref_axis',(1.,0.,0.));
#13283=DIRECTION('center_axis',(0.,0.,1.));
#13284=DIRECTION('ref_axis',(1.,0.,0.));
#13285=DIRECTION('',(0.,0.,1.));
#13286=DIRECTION('center_axis',(0.,0.,1.));
#13287=DIRECTION('ref_axis',(1.,0.,0.));
#13288=DIRECTION('center_axis',(0.,0.,1.));
#13289=DIRECTION('ref_axis',(1.,0.,0.));
#13290=DIRECTION('',(-0.707106781186566,-8.65956056235516E-17,0.707106781186529));
#13291=DIRECTION('center_axis',(0.,0.,1.));
#13292=DIRECTION('ref_axis',(1.,0.,0.));
#13293=DIRECTION('center_axis',(0.,0.,1.));
#13294=DIRECTION('ref_axis',(1.,0.,0.));
#13295=DIRECTION('center_axis',(0.,0.,1.));
#13296=DIRECTION('ref_axis',(1.,0.,0.));
#13297=DIRECTION('',(0.,0.,1.));
#13298=DIRECTION('center_axis',(0.,0.,1.));
#13299=DIRECTION('ref_axis',(1.,0.,0.));
#13300=DIRECTION('center_axis',(0.,0.,1.));
#13301=DIRECTION('ref_axis',(1.,0.,0.));
#13302=DIRECTION('',(-0.707106781186558,-8.65956056235506E-17,0.707106781186537));
#13303=DIRECTION('center_axis',(0.,0.,1.));
#13304=DIRECTION('ref_axis',(1.,0.,0.));
#13305=DIRECTION('center_axis',(0.,0.,1.));
#13306=DIRECTION('ref_axis',(1.,0.,0.));
#13307=DIRECTION('center_axis',(0.,0.,1.));
#13308=DIRECTION('ref_axis',(1.,0.,0.));
#13309=DIRECTION('',(0.,0.,1.));
#13310=DIRECTION('center_axis',(0.,0.,1.));
#13311=DIRECTION('ref_axis',(1.,0.,0.));
#13312=DIRECTION('center_axis',(0.,0.,1.));
#13313=DIRECTION('ref_axis',(1.,0.,0.));
#13314=DIRECTION('',(-0.707106781186566,-8.65956056235516E-17,0.707106781186529));
#13315=DIRECTION('center_axis',(0.,0.,1.));
#13316=DIRECTION('ref_axis',(1.,0.,0.));
#13317=DIRECTION('center_axis',(0.,0.,1.));
#13318=DIRECTION('ref_axis',(1.,0.,0.));
#13319=DIRECTION('center_axis',(0.,0.,1.));
#13320=DIRECTION('ref_axis',(1.,0.,0.));
#13321=DIRECTION('',(0.,0.,1.));
#13322=DIRECTION('center_axis',(0.,0.,1.));
#13323=DIRECTION('ref_axis',(1.,0.,0.));
#13324=DIRECTION('center_axis',(0.,0.,1.));
#13325=DIRECTION('ref_axis',(1.,0.,0.));
#13326=DIRECTION('',(-0.707106781186566,-8.65956056235516E-17,0.707106781186529));
#13327=DIRECTION('center_axis',(0.,0.,1.));
#13328=DIRECTION('ref_axis',(1.,0.,0.));
#13329=DIRECTION('center_axis',(0.,0.,1.));
#13330=DIRECTION('ref_axis',(1.,0.,0.));
#13331=DIRECTION('center_axis',(0.,0.,1.));
#13332=DIRECTION('ref_axis',(1.,0.,0.));
#13333=DIRECTION('',(0.,0.,1.));
#13334=DIRECTION('center_axis',(0.,0.,1.));
#13335=DIRECTION('ref_axis',(1.,0.,0.));
#13336=DIRECTION('center_axis',(0.,0.,1.));
#13337=DIRECTION('ref_axis',(1.,0.,0.));
#13338=DIRECTION('',(-0.707106781186558,-8.65956056235506E-17,0.707106781186537));
#13339=DIRECTION('center_axis',(0.,0.,1.));
#13340=DIRECTION('ref_axis',(1.,0.,0.));
#13341=DIRECTION('center_axis',(0.,0.,1.));
#13342=DIRECTION('ref_axis',(1.,0.,0.));
#13343=DIRECTION('center_axis',(0.,0.,1.));
#13344=DIRECTION('ref_axis',(1.,0.,0.));
#13345=DIRECTION('',(0.,0.,1.));
#13346=DIRECTION('center_axis',(0.,0.,-1.));
#13347=DIRECTION('ref_axis',(-1.,0.,0.));
#13348=DIRECTION('',(0.,0.,1.));
#13349=DIRECTION('center_axis',(0.,0.,-1.));
#13350=DIRECTION('ref_axis',(-1.,0.,0.));
#13351=DIRECTION('center_axis',(0.,0.,-1.));
#13352=DIRECTION('ref_axis',(1.,0.,0.));
#13353=DIRECTION('',(0.707106781186562,-8.65956056235511E-17,-0.707106781186533));
#13354=DIRECTION('center_axis',(0.,0.,1.));
#13355=DIRECTION('ref_axis',(1.,0.,0.));
#13356=DIRECTION('center_axis',(0.,0.,1.));
#13357=DIRECTION('ref_axis',(1.,0.,0.));
#13358=DIRECTION('center_axis',(0.,0.,1.));
#13359=DIRECTION('ref_axis',(1.,0.,0.));
#13360=DIRECTION('center_axis',(0.,0.,1.));
#13361=DIRECTION('ref_axis',(1.,0.,0.));
#13362=DIRECTION('',(-0.707106781186562,-8.65956056235511E-17,0.707106781186533));
#13363=DIRECTION('center_axis',(0.,0.,-1.));
#13364=DIRECTION('ref_axis',(1.,0.,0.));
#13365=DIRECTION('center_axis',(0.,0.,-1.));
#13366=DIRECTION('ref_axis',(-1.,0.,0.));
#13367=DIRECTION('',(0.,0.,-1.));
#13368=DIRECTION('center_axis',(0.,-1.,0.));
#13369=DIRECTION('ref_axis',(0.,0.,-1.));
#13370=DIRECTION('center_axis',(0.,-1.,0.));
#13371=DIRECTION('ref_axis',(0.,0.,-1.));
#13372=DIRECTION('',(0.,-1.,0.));
#13373=DIRECTION('center_axis',(0.,-1.,0.));
#13374=DIRECTION('ref_axis',(0.,0.,-1.));
#13375=DIRECTION('center_axis',(0.,-1.,0.));
#13376=DIRECTION('ref_axis',(0.,0.,-1.));
#13377=DIRECTION('center_axis',(0.,-1.,0.));
#13378=DIRECTION('ref_axis',(0.,0.,-1.));
#13379=DIRECTION('',(0.,-1.,0.));
#13380=DIRECTION('center_axis',(0.,-1.,0.));
#13381=DIRECTION('ref_axis',(0.,0.,-1.));
#13382=DIRECTION('center_axis',(0.,-1.,0.));
#13383=DIRECTION('ref_axis',(0.,0.,-1.));
#13384=DIRECTION('center_axis',(0.,1.,0.));
#13385=DIRECTION('ref_axis',(0.,0.,1.));
#13386=DIRECTION('',(0.,-1.,0.));
#13387=DIRECTION('center_axis',(0.,-1.,0.));
#13388=DIRECTION('ref_axis',(0.,0.,-1.));
#13389=DIRECTION('center_axis',(0.,-1.,0.));
#13390=DIRECTION('ref_axis',(0.,0.,-1.));
#13391=DIRECTION('center_axis',(0.,1.,0.));
#13392=DIRECTION('ref_axis',(0.,0.,1.));
#13393=DIRECTION('',(0.,-1.,0.));
#13394=DIRECTION('center_axis',(0.,-1.,0.));
#13395=DIRECTION('ref_axis',(0.,0.,-1.));
#13396=DIRECTION('center_axis',(2.52323414687536E-16,0.,1.));
#13397=DIRECTION('ref_axis',(1.,0.,-2.52323414687536E-16));
#13398=DIRECTION('center_axis',(-8.7764665978268E-18,-5.25222157317359E-18,
1.));
#13399=DIRECTION('ref_axis',(1.,-4.60959472013434E-35,8.7764665978268E-18));
#13400=DIRECTION('',(2.52323414687536E-16,0.,1.));
#13401=DIRECTION('center_axis',(2.52323414687536E-16,0.,1.));
#13402=DIRECTION('ref_axis',(1.,0.,-2.52323414687536E-16));
#13403=DIRECTION('',(0.,0.,-1.));
#13404=DIRECTION('center_axis',(0.,0.,-1.));
#13405=DIRECTION('ref_axis',(-1.,0.,0.));
#13406=DIRECTION('center_axis',(0.,0.,1.));
#13407=DIRECTION('ref_axis',(1.,0.,0.));
#13408=DIRECTION('center_axis',(0.,0.,1.));
#13409=DIRECTION('ref_axis',(-1.,-4.44089209850063E-15,0.));
#13410=DIRECTION('',(0.,0.,-1.));
#13411=DIRECTION('center_axis',(0.,0.,1.));
#13412=DIRECTION('ref_axis',(1.,0.,0.));
#13413=DIRECTION('',(-2.52323414687536E-16,0.,-1.));
#13414=DIRECTION('center_axis',(2.52323414687536E-16,0.,1.));
#13415=DIRECTION('ref_axis',(1.,0.,-2.52323414687536E-16));
#13416=DIRECTION('center_axis',(0.,0.,1.));
#13417=DIRECTION('ref_axis',(1.,0.,0.));
#13418=DIRECTION('center_axis',(0.,0.,1.));
#13419=DIRECTION('ref_axis',(1.,0.,0.));
#13420=DIRECTION('',(0.,0.,-1.));
#13421=DIRECTION('center_axis',(0.,0.,1.));
#13422=DIRECTION('ref_axis',(1.,0.,0.));
#13423=DIRECTION('center_axis',(0.,0.,1.));
#13424=DIRECTION('ref_axis',(1.,0.,0.));
#13425=DIRECTION('',(2.52323414687536E-16,0.,1.));
#13426=DIRECTION('center_axis',(0.,0.,-1.));
#13427=DIRECTION('ref_axis',(-1.,0.,0.));
#13428=DIRECTION('',(0.,0.,1.));
#13429=DIRECTION('',(0.,0.,-1.));
#13430=DIRECTION('',(0.,0.,1.));
#13431=DIRECTION('center_axis',(0.,0.,1.));
#13432=DIRECTION('ref_axis',(1.,0.,0.));
#13433=DIRECTION('center_axis',(2.52323414687536E-16,0.,1.));
#13434=DIRECTION('ref_axis',(-1.,-4.44089209850063E-15,2.52323414687536E-16));
#13435=DIRECTION('center_axis',(-2.52323414687536E-16,0.,-1.));
#13436=DIRECTION('ref_axis',(1.,-4.44089209850063E-15,-2.52323414687536E-16));
#13437=DIRECTION('center_axis',(0.,0.,1.));
#13438=DIRECTION('ref_axis',(1.,0.,0.));
#13439=DIRECTION('',(0.,0.,-1.));
#13440=DIRECTION('center_axis',(0.,0.,-1.));
#13441=DIRECTION('ref_axis',(1.,0.,0.));
#13442=DIRECTION('center_axis',(0.,0.,-1.));
#13443=DIRECTION('ref_axis',(1.,0.,0.));
#13444=DIRECTION('',(0.,0.,1.));
#13445=DIRECTION('center_axis',(0.,0.,1.));
#13446=DIRECTION('ref_axis',(1.,0.,0.));
#13447=DIRECTION('center_axis',(0.,0.,1.));
#13448=DIRECTION('ref_axis',(-1.,0.,0.));
#13449=DIRECTION('',(0.,0.,-1.));
#13450=DIRECTION('center_axis',(0.,0.,-1.));
#13451=DIRECTION('ref_axis',(-1.,0.,0.));
#13452=DIRECTION('center_axis',(0.,0.,-1.));
#13453=DIRECTION('ref_axis',(1.,0.,0.));
#13454=DIRECTION('',(0.,0.,1.));
#13455=DIRECTION('center_axis',(0.,0.,1.));
#13456=DIRECTION('ref_axis',(1.,0.,0.));
#13457=DIRECTION('',(0.,0.,1.));
#13458=DIRECTION('center_axis',(0.,0.,-1.));
#13459=DIRECTION('ref_axis',(-1.,0.,0.));
#13460=DIRECTION('',(0.,0.,1.));
#13461=DIRECTION('center_axis',(0.,0.,1.));
#13462=DIRECTION('ref_axis',(-1.,0.,0.));
#13463=DIRECTION('',(0.,0.,1.));
#13464=DIRECTION('center_axis',(0.,0.,1.));
#13465=DIRECTION('ref_axis',(1.,0.,0.));
#13466=DIRECTION('',(0.,0.,-1.));
#13467=DIRECTION('center_axis',(0.,0.,-1.));
#13468=DIRECTION('ref_axis',(1.,1.06581410364015E-14,0.));
#13469=DIRECTION('',(0.,0.,1.));
#13470=DIRECTION('center_axis',(0.,1.,0.));
#13471=DIRECTION('ref_axis',(0.,0.,1.));
#13472=DIRECTION('',(1.,0.,0.));
#13473=DIRECTION('',(0.,0.,1.));
#13474=DIRECTION('',(-1.,0.,0.));
#13475=DIRECTION('',(-0.707106781186547,0.,-0.707106781186547));
#13476=DIRECTION('',(0.,0.,-1.));
#13477=DIRECTION('',(0.707106781186547,0.,-0.707106781186547));
#13478=DIRECTION('center_axis',(0.,-1.,0.));
#13479=DIRECTION('ref_axis',(0.,0.,-1.));
#13480=DIRECTION('',(-0.707106781186547,0.,0.707106781186547));
#13481=DIRECTION('',(0.,0.,1.));
#13482=DIRECTION('',(0.707106781186547,0.,0.707106781186547));
#13483=DIRECTION('',(1.,0.,0.));
#13484=DIRECTION('',(0.,0.,-1.));
#13485=DIRECTION('',(-1.,0.,0.));
#13486=DIRECTION('center_axis',(0.,1.,0.));
#13487=DIRECTION('ref_axis',(0.,0.,-1.));
#13488=DIRECTION('',(0.,0.,-1.));
#13489=DIRECTION('center_axis',(0.,1.,0.));
#13490=DIRECTION('ref_axis',(0.,0.,-1.));
#13491=DIRECTION('',(1.,0.,0.));
#13492=DIRECTION('',(0.,0.,-1.));
#13493=DIRECTION('',(-1.,0.,0.));
#13494=DIRECTION('center_axis',(0.,1.,0.));
#13495=DIRECTION('ref_axis',(0.,0.,-1.));
#13496=DIRECTION('',(0.,0.,-1.));
#13497=DIRECTION('center_axis',(0.,1.,0.));
#13498=DIRECTION('ref_axis',(0.,0.,-1.));
#13499=DIRECTION('',(1.,0.,0.));
#13500=DIRECTION('',(0.,0.,-1.));
#13501=DIRECTION('',(-1.,0.,0.));
#13502=DIRECTION('center_axis',(0.,1.,0.));
#13503=DIRECTION('ref_axis',(0.,0.,1.));
#13504=DIRECTION('',(-1.,0.,0.));
#13505=DIRECTION('',(1.,0.,0.));
#13506=DIRECTION('',(0.707106781186548,0.,-0.707106781186548));
#13507=DIRECTION('',(0.,0.,-1.));
#13508=DIRECTION('',(-0.707106781186547,0.,-0.707106781186547));
#13509=DIRECTION('',(-1.,0.,0.));
#13510=DIRECTION('',(1.,0.,0.));
#13511=DIRECTION('center_axis',(0.,1.,0.));
#13512=DIRECTION('ref_axis',(0.,0.,1.));
#13513=DIRECTION('',(0.,0.,1.));
#13514=DIRECTION('center_axis',(0.,1.,0.));
#13515=DIRECTION('ref_axis',(0.,0.,1.));
#13516=DIRECTION('',(-1.,0.,0.));
#13517=DIRECTION('',(1.,0.,0.));
#13518=DIRECTION('center_axis',(0.,1.,0.));
#13519=DIRECTION('ref_axis',(0.,0.,1.));
#13520=DIRECTION('',(0.,0.,1.));
#13521=DIRECTION('center_axis',(0.,1.,0.));
#13522=DIRECTION('ref_axis',(0.,0.,1.));
#13523=DIRECTION('center_axis',(0.,0.,1.));
#13524=DIRECTION('ref_axis',(1.,0.,0.));
#13525=DIRECTION('center_axis',(-2.52323414687536E-16,0.,-1.));
#13526=DIRECTION('ref_axis',(-1.,0.,2.52323414687536E-16));
#13527=DIRECTION('center_axis',(-2.52323414687536E-16,0.,-1.));
#13528=DIRECTION('ref_axis',(1.,5.15143483426073E-14,-2.52323414687536E-16));
#13529=DIRECTION('center_axis',(2.52323414687536E-16,0.,1.));
#13530=DIRECTION('ref_axis',(-1.,4.9737991503207E-14,2.52323414687536E-16));
#13531=DIRECTION('',(-2.52323414687536E-16,0.,-1.));
#13532=DIRECTION('center_axis',(-2.52323414687536E-16,0.,-1.));
#13533=DIRECTION('ref_axis',(-1.,0.,2.52323414687536E-16));
#13534=DIRECTION('center_axis',(-2.52323414687536E-16,0.,-1.));
#13535=DIRECTION('ref_axis',(-1.,0.,2.52323414687536E-16));
#13536=DIRECTION('center_axis',(-2.52323414687536E-16,0.,-1.));
#13537=DIRECTION('ref_axis',(-1.,0.,2.52323414687536E-16));
#13538=DIRECTION('center_axis',(2.52323414687536E-16,0.,1.));
#13539=DIRECTION('ref_axis',(-1.,1.77635683940025E-15,2.52323414687536E-16));
#13540=DIRECTION('',(3.46944695195362E-15,-1.,-8.754227019942E-31));
#13541=DIRECTION('center_axis',(-2.52323414687536E-16,0.,-1.));
#13542=DIRECTION('ref_axis',(-1.,0.,2.52323414687536E-16));
#13543=DIRECTION('center_axis',(-2.52323414687536E-16,0.,-1.));
#13544=DIRECTION('ref_axis',(-1.,0.,2.52323414687536E-16));
#13545=DIRECTION('center_axis',(2.52323414687536E-16,0.,1.));
#13546=DIRECTION('ref_axis',(1.,0.,-2.52323414687536E-16));
#13547=DIRECTION('center_axis',(-0.0237269141195627,-0.851557493622926,
0.523724038593803));
#13548=DIRECTION('ref_axis',(-0.0385579135341051,0.524261227788714,0.85068410843354));
#13549=DIRECTION('',(-3.04630100940178E-45,8.57457505675013E-31,-1.));
#13550=DIRECTION('center_axis',(-0.0237269141195507,-0.851557493623381,
-0.523724038593063));
#13551=DIRECTION('ref_axis',(0.0146007549783791,0.523520473997797,-0.851887980464089));
#13552=DIRECTION('center_axis',(-2.52323414687536E-16,0.,-1.));
#13553=DIRECTION('ref_axis',(-1.,0.,2.52323414687536E-16));
#13554=DIRECTION('center_axis',(2.52323414687536E-16,0.,1.));
#13555=DIRECTION('ref_axis',(1.,0.,-2.52323414687536E-16));
#13556=DIRECTION('center_axis',(-2.52323414687536E-16,0.,-1.));
#13557=DIRECTION('ref_axis',(1.,-8.88178419700125E-16,-2.52323414687536E-16));
#13558=DIRECTION('center_axis',(2.52323414687536E-16,0.,1.));
#13559=DIRECTION('ref_axis',(1.,0.,-2.52323414687536E-16));
#13560=DIRECTION('center_axis',(2.52323414687536E-16,0.,1.));
#13561=DIRECTION('ref_axis',(1.,0.,-2.52323414687536E-16));
#13562=DIRECTION('center_axis',(2.52323414687536E-16,0.,1.));
#13563=DIRECTION('ref_axis',(1.,0.,-2.52323414687536E-16));
#13564=DIRECTION('',(-3.46944695195361E-15,1.,8.75422701994197E-31));
#13565=DIRECTION('center_axis',(-1.,-3.46944695195361E-15,2.41352831440251E-16));
#13566=DIRECTION('ref_axis',(3.46944695195361E-15,-1.,-4.87884146037003E-48));
#13567=DIRECTION('',(3.46944695195361E-15,-1.,0.));
#13568=DIRECTION('center_axis',(-1.,-5.52038264252701E-15,6.2479767589266E-16));
#13569=DIRECTION('ref_axis',(-4.16417573426786E-15,0.819231920519141,0.573462344363185));
#13570=DIRECTION('',(2.41352831440251E-16,0.,1.));
#13571=DIRECTION('center_axis',(-1.,-1.42770121134483E-15,3.50862385444968E-15));
#13572=DIRECTION('ref_axis',(-3.18168206635957E-15,0.819231920518936,-0.573462344363477));
#13573=DIRECTION('',(-3.46944695195361E-15,1.,0.));
#13574=DIRECTION('center_axis',(-1.,-8.96139251667977E-15,-8.32782443095335E-16));
#13575=DIRECTION('ref_axis',(8.32782443102262E-16,-7.72993066836482E-13,
-1.));
#13576=DIRECTION('',(-2.41352831440251E-16,0.,-1.));
#13577=DIRECTION('center_axis',(-1.,0.,0.));
#13578=DIRECTION('ref_axis',(0.,-5.23876817808574E-13,-1.));
#13579=DIRECTION('',(3.46944695195361E-15,-1.,1.91404262256119E-33));
#13580=DIRECTION('center_axis',(-1.,-1.17134969274264E-14,8.78564447069424E-15));
#13581=DIRECTION('ref_axis',(-8.78564447074124E-15,4.012053825336E-12,-1.));
#13582=DIRECTION('',(-2.41352831440251E-16,0.,-1.));
#13583=DIRECTION('center_axis',(-1.,-4.85188929015585E-15,-1.99030797820559E-15));
#13584=DIRECTION('ref_axis',(1.99030797821407E-15,-1.7484297207494E-12,
-1.));
#13585=DIRECTION('',(-3.46944695195361E-15,1.,0.));
#13586=DIRECTION('center_axis',(-1.,-6.86244039359303E-15,6.93075172121948E-15));
#13587=DIRECTION('ref_axis',(-9.59645535334076E-15,0.819231920519237,-0.573462344363048));
#13588=DIRECTION('',(2.41352831440251E-16,-1.24480026177148E-32,1.));
#13589=DIRECTION('center_axis',(-1.,6.86244039359302E-15,6.93075172121946E-15));
#13590=DIRECTION('ref_axis',(9.5964553533418E-15,0.819231920518884,0.573462344363551));
#13591=DIRECTION('center_axis',(3.5527136788005E-15,-1.,-8.57457505675013E-31));
#13592=DIRECTION('ref_axis',(1.,3.5527136788005E-15,0.));
#13593=DIRECTION('center_axis',(3.5527136788005E-15,-1.,-8.57457505675013E-31));
#13594=DIRECTION('ref_axis',(1.,3.5527136788005E-15,-1.26929208725074E-46));
#13595=DIRECTION('',(-0.99034174667433,-3.51840067009707E-15,-0.138647844534406));
#13596=DIRECTION('',(0.99034174667433,3.51840067009707E-15,-0.138647844534406));
#13597=DIRECTION('center_axis',(3.5527136788005E-15,-1.,-8.57457505675013E-31));
#13598=DIRECTION('ref_axis',(1.,3.5527136788005E-15,-1.26929208725074E-46));
#13599=DIRECTION('center_axis',(-0.138647844534406,-4.81031341614835E-16,
-0.99034174667433));
#13600=DIRECTION('ref_axis',(-0.99034174667433,3.0510584428262E-33,0.138647844534406));
#13601=DIRECTION('',(0.9714691757235,0.194293835144703,-0.13600568460129));
#13602=DIRECTION('center_axis',(-0.138647844534404,-4.3608853103437E-15,
-0.990341746674331));
#13603=DIRECTION('ref_axis',(-0.142395756615647,0.989609027893549,0.0199354059261866));
#13604=DIRECTION('',(-3.46944695195362E-15,1.,8.93770063475844E-31));
#13605=DIRECTION('',(-0.99034174667433,-3.51840067009707E-15,0.138647844534406));
#13606=DIRECTION('center_axis',(-0.138647844534406,-4.81031341614834E-16,
0.99034174667433));
#13607=DIRECTION('ref_axis',(0.99034174667433,1.28749462997746E-32,0.138647844534406));
#13608=DIRECTION('',(3.46944695195361E-15,-1.,-8.93770063475844E-31));
#13609=DIRECTION('center_axis',(-0.138647844534388,-1.15563460846761E-13,
0.990341746674333));
#13610=DIRECTION('ref_axis',(-0.192413756189552,0.980944083309055,-0.0269379258664217));
#13611=DIRECTION('',(-0.9714691757235,-0.194293835144703,-0.13600568460129));
#13612=DIRECTION('',(0.99034174667433,3.51840067009707E-15,0.138647844534406));
#13613=DIRECTION('center_axis',(-0.196116135138187,0.98058067569092,4.73331845067205E-17));
#13614=DIRECTION('ref_axis',(-0.980580675690919,-0.196116135138187,9.12179048335121E-36));
#13615=DIRECTION('',(0.9714691757235,0.194293835144703,0.13600568460129));
#13616=DIRECTION('',(2.51901469178025E-16,2.10972754755468E-18,1.));
#13617=DIRECTION('',(-0.9714691757235,-0.194293835144703,0.13600568460129));
#13618=DIRECTION('center_axis',(3.46944695195362E-15,-1.,-8.754227019942E-31));
#13619=DIRECTION('ref_axis',(1.,3.46944695195362E-15,0.));
#13620=DIRECTION('center_axis',(0.0303922984798993,0.807916267226531,0.588513052823688));
#13621=DIRECTION('ref_axis',(-0.0416915731841444,0.589297297589034,-0.806839827834306));
#13622=DIRECTION('center_axis',(-3.5527136788005E-15,1.,8.57457505675013E-31));
#13623=DIRECTION('ref_axis',(1.,3.5527136788005E-15,1.90393813087611E-46));
#13624=DIRECTION('center_axis',(-2.52323414687536E-16,0.,-1.));
#13625=DIRECTION('ref_axis',(-1.,0.,2.52323414687536E-16));
#13626=DIRECTION('center_axis',(-2.52323414687536E-16,0.,-1.));
#13627=DIRECTION('ref_axis',(1.,0.,-2.52323414687536E-16));
#13628=DIRECTION('center_axis',(2.52323414687536E-16,0.,1.));
#13629=DIRECTION('ref_axis',(-1.,-1.85962356624714E-14,2.52323414687536E-16));
#13630=DIRECTION('center_axis',(0.185712190755878,-2.42469285118642E-13,
0.982604183893317));
#13631=DIRECTION('ref_axis',(-0.189474179318918,0.981232457104028,0.0358106198915277));
#13632=DIRECTION('center_axis',(0.185712190755882,-2.44440580120635E-13,
-0.982604183893317));
#13633=DIRECTION('ref_axis',(-0.140198967511934,0.98976872371543,-0.0264976048600095));
#13634=DIRECTION('center_axis',(-3.46944695195361E-15,1.,8.75422701994197E-31));
#13635=DIRECTION('ref_axis',(-1.,-3.46944695195361E-15,6.22301527786114E-61));
#13636=DIRECTION('center_axis',(-3.5527136788005E-15,1.,8.57457505675013E-31));
#13637=DIRECTION('ref_axis',(1.,3.5527136788005E-15,1.90393813087611E-46));
#13638=DIRECTION('center_axis',(0.0303922984798813,0.807916267226852,-0.588513052823249));
#13639=DIRECTION('ref_axis',(0.0221372134653148,0.588096554362881,0.808487715754852));
#13640=DIRECTION('center_axis',(-0.9714691757235,-0.194293835144704,-0.13600568460129));
#13641=DIRECTION('ref_axis',(0.196116135138187,-0.98058067569092,-3.92731709847666E-18));
#13642=DIRECTION('center_axis',(0.9714691757235,0.194293835144703,0.136005684601291));
#13643=DIRECTION('ref_axis',(-0.196116135138187,0.98058067569092,3.24008523737298E-18));
#13644=DIRECTION('center_axis',(0.980051041638971,0.143785099769423,0.137207145829456));
#13645=DIRECTION('ref_axis',(-0.145157949036735,0.989408494925856,2.07268495050659E-17));
#13646=DIRECTION('center_axis',(0.999978809045156,0.00651010450232906,-3.96499820692563E-16));
#13647=DIRECTION('ref_axis',(-0.00651010450232906,0.999978809045156,6.00796001774974E-35));
#13648=DIRECTION('center_axis',(2.52323414687536E-16,0.,1.));
#13649=DIRECTION('ref_axis',(1.,0.,-2.507797890918E-16));
#13650=DIRECTION('center_axis',(0.994514519537326,-0.104598615810349,-3.94333184969416E-16));
#13651=DIRECTION('ref_axis',(0.104598615810349,0.994514519537326,5.49398292351409E-33));
#13652=DIRECTION('center_axis',(2.52323414687536E-16,0.,1.));
#13653=DIRECTION('ref_axis',(1.,0.,-2.3201395453391E-16));
#13654=DIRECTION('center_axis',(-0.9714691757235,-0.194293835144704,0.13600568460129));
#13655=DIRECTION('ref_axis',(0.196116135138187,-0.98058067569092,7.05725267053878E-18));
#13656=DIRECTION('center_axis',(0.9714691757235,0.194293835144703,-0.13600568460129));
#13657=DIRECTION('ref_axis',(-0.196116135138187,0.98058067569092,-4.37148606784657E-18));
#13658=DIRECTION('center_axis',(0.980051041638971,0.143785099769423,-0.137207145829457));
#13659=DIRECTION('ref_axis',(-0.145157949036735,0.989408494925857,5.49111790108275E-17));
#13660=DIRECTION('center_axis',(0.999978809045156,0.00651010450232827,-3.96499820692563E-16));
#13661=DIRECTION('ref_axis',(-0.00651010450232827,0.999978809045156,2.30522657691445E-35));
#13662=DIRECTION('center_axis',(-2.52323414687536E-16,0.,-1.));
#13663=DIRECTION('ref_axis',(-1.,0.,2.507797890918E-16));
#13664=DIRECTION('center_axis',(0.994514519537326,-0.104598615810349,-3.94333184969416E-16));
#13665=DIRECTION('ref_axis',(0.104598615810349,0.994514519537326,5.49398292351409E-33));
#13666=DIRECTION('center_axis',(-2.52323414687536E-16,0.,-1.));
#13667=DIRECTION('ref_axis',(-1.,0.,2.3201395453391E-16));
#13668=DIRECTION('center_axis',(-0.99034174667433,-3.51840067009707E-15,
-0.138647844534406));
#13669=DIRECTION('ref_axis',(-0.138647844534406,-3.36051524361832E-32,0.99034174667433));
#13670=DIRECTION('center_axis',(0.99034174667433,3.14142916972953E-15,0.138647844534406));
#13671=DIRECTION('ref_axis',(0.138647844534406,-8.69074855760808E-32,-0.99034174667433));
#13672=DIRECTION('center_axis',(3.5527136788005E-15,-1.,-8.57457505675013E-31));
#13673=DIRECTION('ref_axis',(1.,3.5109170472852E-15,0.));
#13674=DIRECTION('center_axis',(0.998667820387802,2.79231993889397E-15,
0.0516002376145364));
#13675=DIRECTION('ref_axis',(0.0516002376145364,-2.37256198805332E-32,-0.998667820387802));
#13676=DIRECTION('center_axis',(0.999611719795952,-0.0278641283118466,-3.96354266786649E-16));
#13677=DIRECTION('ref_axis',(0.0278641283118466,0.999611719795952,-1.9098216440265E-32));
#13678=DIRECTION('center_axis',(2.52323414687536E-16,0.,1.));
#13679=DIRECTION('ref_axis',(1.,0.,-2.49313240617579E-16));
#13680=DIRECTION('center_axis',(-0.99034174667433,-3.51840067009707E-15,
0.138647844534406));
#13681=DIRECTION('ref_axis',(0.138647844534406,-3.67558502487976E-34,0.99034174667433));
#13682=DIRECTION('center_axis',(0.99034174667433,3.14142916972953E-15,-0.138647844534406));
#13683=DIRECTION('ref_axis',(-0.138647844534406,-1.13235899567505E-30,-0.99034174667433));
#13684=DIRECTION('center_axis',(3.5527136788005E-15,-1.,-8.57457505675013E-31));
#13685=DIRECTION('ref_axis',(1.,3.5109170472852E-15,0.));
#13686=DIRECTION('center_axis',(0.998667820387802,3.56382002618601E-15,
-0.0516002376145376));
#13687=DIRECTION('ref_axis',(-0.0516002376145376,-4.64884186281675E-32,
-0.998667820387802));
#13688=DIRECTION('center_axis',(0.999611719795952,-0.0278641283118465,-3.74257554777419E-16));
#13689=DIRECTION('ref_axis',(0.0278641283118465,0.999611719795952,-1.41173314945589E-33));
#13690=DIRECTION('center_axis',(-2.52323414687536E-16,0.,-1.));
#13691=DIRECTION('ref_axis',(-1.,0.,2.49313240617579E-16));
#13692=DIRECTION('center_axis',(0.935358342755929,-0.353701527614572,-8.65380307002384E-16));
#13693=DIRECTION('ref_axis',(0.353701527614572,0.935358342755929,3.79648143258003E-33));
#13694=DIRECTION('center_axis',(-2.52323414687536E-16,0.,-1.));
#13695=DIRECTION('ref_axis',(-1.,0.,2.1316282072803E-16));
#13696=DIRECTION('center_axis',(0.996895904609183,0.0787309048178608,-4.61156994354849E-16));
#13697=DIRECTION('ref_axis',(-0.0787309048178608,0.996895904609183,8.19223082641905E-33));
#13698=DIRECTION('center_axis',(-0.996895904609183,-0.0787309048178614,
1.15289248588712E-16));
#13699=DIRECTION('ref_axis',(0.0787309048178614,-0.996895904609183,1.91107223648995E-33));
#13700=DIRECTION('center_axis',(2.52323414687536E-16,0.,1.));
#13701=DIRECTION('ref_axis',(1.,0.,-2.1316282072803E-16));
#13702=DIRECTION('center_axis',(-0.93535834275593,0.353701527614571,8.65380307002384E-16));
#13703=DIRECTION('ref_axis',(-0.353701527614571,-0.93535834275593,3.5407744807615E-31));
#13704=DIRECTION('center_axis',(0.,0.,1.));
#13705=DIRECTION('ref_axis',(1.,0.,0.));
#13706=DIRECTION('center_axis',(0.,0.,-1.));
#13707=DIRECTION('ref_axis',(-1.,0.,0.));
#13708=DIRECTION('center_axis',(-2.52323414687536E-16,0.,-1.));
#13709=DIRECTION('ref_axis',(-1.,0.,2.52323414687536E-16));
#13710=DIRECTION('center_axis',(-2.52323414687536E-16,0.,-1.));
#13711=DIRECTION('ref_axis',(-1.,0.,2.52323414687536E-16));
#13712=DIRECTION('',(-2.52323414687536E-16,0.,-1.));
#13713=DIRECTION('center_axis',(2.52323414687536E-16,0.,1.));
#13714=DIRECTION('ref_axis',(-1.,4.9737991503207E-14,2.52323414687536E-16));
#13715=DIRECTION('center_axis',(-2.52323414687536E-16,0.,-1.));
#13716=DIRECTION('ref_axis',(-1.,0.,2.52323414687536E-16));
#13717=DIRECTION('center_axis',(-2.52323414687536E-16,0.,-1.));
#13718=DIRECTION('ref_axis',(-1.,0.,2.52323414687536E-16));
#13719=DIRECTION('center_axis',(-2.52323414687536E-16,0.,-1.));
#13720=DIRECTION('ref_axis',(-1.,0.,2.52323414687536E-16));
#13721=DIRECTION('',(0.,-1.,0.));
#13722=DIRECTION('center_axis',(2.52323414687536E-16,0.,1.));
#13723=DIRECTION('ref_axis',(-1.,1.77635683940025E-15,2.52323414687536E-16));
#13724=DIRECTION('center_axis',(-2.52323414687536E-16,0.,-1.));
#13725=DIRECTION('ref_axis',(-1.,0.,2.52323414687536E-16));
#13726=DIRECTION('center_axis',(-2.52323414687536E-16,0.,-1.));
#13727=DIRECTION('ref_axis',(-1.,0.,2.52323414687536E-16));
#13728=DIRECTION('center_axis',(-2.52323414687536E-16,0.,-1.));
#13729=DIRECTION('ref_axis',(-1.,0.,2.52323414687536E-16));
#13730=DIRECTION('center_axis',(-0.0239544909236863,-0.859725218195524,
-0.510194797663838));
#13731=DIRECTION('ref_axis',(0.0142235277005771,0.509996493084021,-0.860058874904359));
#13732=DIRECTION('',(-3.04630100940178E-45,8.57457505675013E-31,-1.));
#13733=DIRECTION('center_axis',(-0.023954490923717,-0.859725218194695,0.510194797665234));
#13734=DIRECTION('ref_axis',(-0.0403411650264477,0.510756839498867,0.858778225917168));
#13735=DIRECTION('center_axis',(2.52323414687536E-16,0.,1.));
#13736=DIRECTION('ref_axis',(-1.,8.88178419700125E-16,2.52323414687536E-16));
#13737=DIRECTION('center_axis',(2.52323414687536E-16,0.,1.));
#13738=DIRECTION('ref_axis',(1.,0.,-2.52323414687536E-16));
#13739=DIRECTION('center_axis',(-2.52323414687536E-16,0.,-1.));
#13740=DIRECTION('ref_axis',(1.,-8.88178419700125E-16,-2.52323414687536E-16));
#13741=DIRECTION('',(0.,1.,0.));
#13742=DIRECTION('center_axis',(2.52323414687536E-16,0.,1.));
#13743=DIRECTION('ref_axis',(1.,0.,-2.52323414687536E-16));
#13744=DIRECTION('center_axis',(2.52323414687536E-16,0.,1.));
#13745=DIRECTION('ref_axis',(1.,0.,-2.52323414687536E-16));
#13746=DIRECTION('center_axis',(2.52323414687536E-16,0.,1.));
#13747=DIRECTION('ref_axis',(1.,0.,-2.52323414687536E-16));
#13748=DIRECTION('center_axis',(3.5527136788005E-15,-1.,-8.57457505675013E-31));
#13749=DIRECTION('ref_axis',(1.,3.5527136788005E-15,0.));
#13750=DIRECTION('center_axis',(3.5527136788005E-15,-1.,-8.57457505675013E-31));
#13751=DIRECTION('ref_axis',(1.,3.5527136788005E-15,-1.26929208725075E-46));
#13752=DIRECTION('',(0.99034174667433,3.51840067009707E-15,-0.138647844534406));
#13753=DIRECTION('',(-0.99034174667433,-3.51840067009707E-15,-0.138647844534406));
#13754=DIRECTION('center_axis',(3.5527136788005E-15,-1.,-8.57457505675013E-31));
#13755=DIRECTION('ref_axis',(1.,3.5527136788005E-15,-1.26929208725075E-46));
#13756=DIRECTION('center_axis',(-0.138647844534406,-4.81031341614835E-16,
-0.99034174667433));
#13757=DIRECTION('ref_axis',(-0.99034174667433,3.0510584428262E-33,0.138647844534406));
#13758=DIRECTION('',(0.9714691757235,0.194293835144703,-0.13600568460129));
#13759=DIRECTION('',(-0.99034174667433,0.,0.138647844534406));
#13760=DIRECTION('',(-6.66939586683906E-17,1.,-4.76385419059932E-16));
#13761=DIRECTION('center_axis',(-0.138647844534408,1.96239838967726E-14,
-0.99034174667433));
#13762=DIRECTION('ref_axis',(-0.142395756615911,0.98960902789351,0.019935405926249));
#13763=DIRECTION('center_axis',(-0.138647844534406,-4.81031341614834E-16,
0.99034174667433));
#13764=DIRECTION('ref_axis',(0.99034174667433,1.28749462997746E-32,0.138647844534406));
#13765=DIRECTION('',(6.66939586683902E-17,-1.,-4.76385419059931E-16));
#13766=DIRECTION('',(0.99034174667433,0.,0.138647844534406));
#13767=DIRECTION('',(-0.9714691757235,-0.194293835144704,-0.13600568460129));
#13768=DIRECTION('center_axis',(-0.138647844534407,4.36088531502231E-15,
0.99034174667433));
#13769=DIRECTION('ref_axis',(-0.192413756189259,0.980944083309111,-0.0269379258665006));
#13770=DIRECTION('center_axis',(-0.196116135138187,0.98058067569092,4.73331845067205E-17));
#13771=DIRECTION('ref_axis',(-0.980580675690919,-0.196116135138187,9.12179048335121E-36));
#13772=DIRECTION('',(-0.9714691757235,-0.194293835144703,0.13600568460129));
#13773=DIRECTION('',(9.28280120924076E-18,-4.6414006046203E-17,1.));
#13774=DIRECTION('',(0.9714691757235,0.194293835144704,0.13600568460129));
#13775=DIRECTION('center_axis',(3.46944695195362E-15,-1.,-8.754227019942E-31));
#13776=DIRECTION('ref_axis',(1.,3.46944695195362E-15,0.));
#13777=DIRECTION('center_axis',(-3.46944695195362E-15,1.,8.754227019942E-31));
#13778=DIRECTION('ref_axis',(1.,3.46944695195362E-15,-5.52224113655355E-47));
#13779=DIRECTION('center_axis',(0.0285016084921434,0.833421796752127,0.551901954165607));
#13780=DIRECTION('ref_axis',(-0.0430076714350775,0.552637411426228,-0.832311379046238));
#13781=DIRECTION('center_axis',(-2.52323414687536E-16,0.,-1.));
#13782=DIRECTION('ref_axis',(-1.,0.,2.52323414687536E-16));
#13783=DIRECTION('center_axis',(0.169336824475723,-4.83683914468181E-13,
-0.985558237688914));
#13784=DIRECTION('ref_axis',(-0.141035172496763,0.989707972370685,-0.0242324069113047));
#13785=DIRECTION('center_axis',(0.169336824475649,-5.71923547513346E-14,
0.985558237688927));
#13786=DIRECTION('ref_axis',(-0.190594454957618,0.981122494345506,0.0327475927155013));
#13787=DIRECTION('center_axis',(2.52323414687536E-16,0.,1.));
#13788=DIRECTION('ref_axis',(-1.,9.71445146547012E-15,2.52323414687536E-16));
#13789=DIRECTION('center_axis',(-2.52323414687536E-16,0.,-1.));
#13790=DIRECTION('ref_axis',(-1.,0.,2.52323414687536E-16));
#13791=DIRECTION('center_axis',(-3.46944695195361E-15,1.,8.75422701994197E-31));
#13792=DIRECTION('ref_axis',(-1.,-3.46944695195361E-15,6.22301527786114E-61));
#13793=DIRECTION('center_axis',(0.0285016084921437,0.833421796752069,-0.551901954165695));
#13794=DIRECTION('ref_axis',(0.0188743829595763,0.551579119228361,0.83390900756567));
#13795=DIRECTION('center_axis',(-3.46944695195361E-15,1.,8.75422701994197E-31));
#13796=DIRECTION('ref_axis',(-1.,-3.46944695195361E-15,5.52224113655467E-47));
#13797=DIRECTION('center_axis',(-0.9714691757235,-0.194293835144704,-0.13600568460129));
#13798=DIRECTION('ref_axis',(0.196116135138187,-0.980580675690919,1.08828652437483E-18));
#13799=DIRECTION('center_axis',(0.971469175723501,0.194293835144703,0.13600568460129));
#13800=DIRECTION('ref_axis',(-0.196116135138187,0.98058067569092,-1.50980502241592E-17));
#13801=DIRECTION('center_axis',(0.980051041638971,0.143785099769423,0.137207145829456));
#13802=DIRECTION('ref_axis',(-0.145157949036735,0.989408494925856,-5.6122374695011E-17));
#13803=DIRECTION('center_axis',(0.999978809045156,0.00651010450232907,-2.52318067713449E-16));
#13804=DIRECTION('ref_axis',(-0.00651010450232907,0.999978809045156,-1.80918359374754E-32));
#13805=DIRECTION('center_axis',(2.52323414687536E-16,0.,1.));
#13806=DIRECTION('ref_axis',(1.,0.,-2.66453525910038E-16));
#13807=DIRECTION('center_axis',(0.994514519537326,-0.104598615810349,-2.50939299525992E-16));
#13808=DIRECTION('ref_axis',(0.104598615810349,0.994514519537326,-1.52162986309358E-32));
#13809=DIRECTION('center_axis',(2.52323414687536E-16,0.,1.));
#13810=DIRECTION('ref_axis',(1.,0.,-2.41886888769396E-16));
#13811=DIRECTION('center_axis',(-0.9714691757235,-0.194293835144704,0.13600568460129));
#13812=DIRECTION('ref_axis',(0.196116135138187,-0.980580675690919,-3.35108818532205E-18));
#13813=DIRECTION('center_axis',(0.9714691757235,0.194293835144703,-0.13600568460129));
#13814=DIRECTION('ref_axis',(0.196116135138188,-0.980580675690919,3.62636123721662E-15));
#13815=DIRECTION('center_axis',(0.980051041638971,0.143785099769423,-0.137207145829457));
#13816=DIRECTION('ref_axis',(-0.145157949036735,0.989408494925857,2.8694747315233E-18));
#13817=DIRECTION('center_axis',(0.999978809045156,0.00651010450232831,-2.52318067713449E-16));
#13818=DIRECTION('ref_axis',(0.0065101045023283,-0.999978809045156,7.13181002470613E-32));
#13819=DIRECTION('center_axis',(-2.52323414687536E-16,0.,-1.));
#13820=DIRECTION('ref_axis',(-1.,0.,2.66453525910038E-16));
#13821=DIRECTION('center_axis',(0.994514519537326,-0.104598615810349,-2.50939299525992E-16));
#13822=DIRECTION('ref_axis',(-0.104598615810349,-0.994514519537326,4.29233327314378E-32));
#13823=DIRECTION('center_axis',(-2.52323414687536E-16,0.,-1.));
#13824=DIRECTION('ref_axis',(-1.,0.,2.41886888769396E-16));
#13825=DIRECTION('center_axis',(-0.99034174667433,-3.51840067009707E-15,
-0.138647844534406));
#13826=DIRECTION('ref_axis',(-0.138647844534406,-3.26527751285154E-32,0.99034174667433));
#13827=DIRECTION('center_axis',(0.99034174667433,3.51840067009707E-15,0.138647844534406));
#13828=DIRECTION('ref_axis',(0.138647844534406,8.65196281794793E-31,-0.99034174667433));
#13829=DIRECTION('center_axis',(3.5527136788005E-15,-1.,-8.57457505675013E-31));
#13830=DIRECTION('ref_axis',(1.,3.5527136788005E-15,0.));
#13831=DIRECTION('center_axis',(0.998667820387802,3.38652769649194E-15,
0.0516002376145362));
#13832=DIRECTION('ref_axis',(0.0516002376145362,-4.34329619623291E-31,-0.998667820387802));
#13833=DIRECTION('center_axis',(0.999611719795952,-0.0278641283118464,-2.52225442500595E-16));
#13834=DIRECTION('ref_axis',(0.0278641283118464,0.999611719795952,-7.27443156916003E-33));
#13835=DIRECTION('center_axis',(2.52323414687536E-16,0.,1.));
#13836=DIRECTION('ref_axis',(1.,0.,-2.58379176640036E-16));
#13837=DIRECTION('center_axis',(-0.99034174667433,-3.51840067009707E-15,
0.138647844534406));
#13838=DIRECTION('ref_axis',(0.138647844534406,1.9494291318743E-31,0.99034174667433));
#13839=DIRECTION('center_axis',(0.99034174667433,3.51840067009707E-15,-0.138647844534406));
#13840=DIRECTION('ref_axis',(0.138647844534406,2.22044604925031E-15,0.99034174667433));
#13841=DIRECTION('center_axis',(3.5527136788005E-15,-1.,-8.57457505675013E-31));
#13842=DIRECTION('ref_axis',(1.,3.5527136788005E-15,0.));
#13843=DIRECTION('center_axis',(0.998667820387802,3.42216846262747E-15,
-0.0516002376145377));
#13844=DIRECTION('ref_axis',(0.0516002376145376,8.88178419700125E-15,0.998667820387802));
#13845=DIRECTION('center_axis',(0.999611719795952,-0.0278641283118467,-2.52225442500595E-16));
#13846=DIRECTION('ref_axis',(-0.0278641283118467,-0.999611719795952,-6.03275671091393E-32));
#13847=DIRECTION('center_axis',(-2.52323414687536E-16,0.,-1.));
#13848=DIRECTION('ref_axis',(-1.,0.,2.58379176640036E-16));
#13849=DIRECTION('center_axis',(0.935358342755929,-0.353701527614572,-2.3601281100065E-16));
#13850=DIRECTION('ref_axis',(-0.353701527614572,-0.935358342755929,-4.5752724171616E-32));
#13851=DIRECTION('center_axis',(-2.52323414687536E-16,0.,-1.));
#13852=DIRECTION('ref_axis',(-1.,0.,2.03012210217171E-16));
#13853=DIRECTION('center_axis',(0.996895904609183,0.0787309048178609,-2.7669419661291E-16));
#13854=DIRECTION('ref_axis',(-0.0787309048178609,0.996895904609183,1.10831582297851E-32));
#13855=DIRECTION('center_axis',(-0.996895904609183,-0.0787309048178616,
2.51540178739009E-16));
#13856=DIRECTION('ref_axis',(-0.0787309048178616,0.996895904609183,9.57629751275587E-34));
#13857=DIRECTION('center_axis',(2.52323414687536E-16,0.,1.));
#13858=DIRECTION('ref_axis',(1.,0.,-2.03012210217171E-16));
#13859=DIRECTION('center_axis',(-0.93535834275593,0.353701527614571,0.));
#13860=DIRECTION('ref_axis',(-0.353701527614571,-0.93535834275593,0.));
#13861=DIRECTION('center_axis',(1.,0.,0.));
#13862=DIRECTION('ref_axis',(0.,0.,-1.));
#13863=DIRECTION('',(0.,0.,-1.));
#13864=DIRECTION('',(0.,1.,0.));
#13865=DIRECTION('',(0.,0.,1.));
#13866=DIRECTION('',(0.,-1.,0.));
#13867=DIRECTION('center_axis',(0.,-1.,0.));
#13868=DIRECTION('ref_axis',(0.,0.,-1.));
#13869=DIRECTION('',(-1.,0.,0.));
#13870=DIRECTION('',(0.,0.,-1.));
#13871=DIRECTION('',(1.,0.,0.));
#13872=DIRECTION('',(0.707106781186548,0.,0.707106781186548));
#13873=DIRECTION('',(0.,0.,1.));
#13874=DIRECTION('',(-0.707106781186547,0.,0.707106781186547));
#13875=DIRECTION('center_axis',(0.,0.,1.));
#13876=DIRECTION('ref_axis',(1.,0.,0.));
#13877=DIRECTION('',(1.,0.,0.));
#13878=DIRECTION('',(0.,1.,0.));
#13879=DIRECTION('',(-1.,0.,0.));
#13880=DIRECTION('center_axis',(0.,0.,-1.));
#13881=DIRECTION('ref_axis',(1.,0.,0.));
#13882=DIRECTION('center_axis',(0.,0.,1.));
#13883=DIRECTION('ref_axis',(1.,0.,0.));
#13884=DIRECTION('',(-1.,0.,0.));
#13885=DIRECTION('center_axis',(0.,0.,1.));
#13886=DIRECTION('ref_axis',(1.,0.,0.));
#13887=DIRECTION('',(1.,0.,0.));
#13888=DIRECTION('',(0.,-1.,0.));
#13889=DIRECTION('center_axis',(-1.,0.,0.));
#13890=DIRECTION('ref_axis',(0.,0.,1.));
#13891=DIRECTION('',(0.,1.,0.));
#13892=DIRECTION('',(0.,0.,1.));
#13893=DIRECTION('',(0.,-1.,0.));
#13894=DIRECTION('',(0.,0.,-1.));
#13895=DIRECTION('center_axis',(0.,0.,1.));
#13896=DIRECTION('ref_axis',(1.,0.,0.));
#13897=DIRECTION('',(-1.,0.,0.));
#13898=DIRECTION('center_axis',(0.,0.,1.));
#13899=DIRECTION('ref_axis',(1.,0.,0.));
#13900=DIRECTION('',(0.,-1.,0.));
#13901=DIRECTION('center_axis',(0.,0.,1.));
#13902=DIRECTION('ref_axis',(1.,0.,0.));
#13903=DIRECTION('',(0.,1.,0.));
#13904=DIRECTION('center_axis',(0.,0.,-1.));
#13905=DIRECTION('ref_axis',(1.,0.,0.));
#13906=DIRECTION('',(1.,0.,0.));
#13907=DIRECTION('center_axis',(1.,0.,0.));
#13908=DIRECTION('ref_axis',(0.,0.,-1.));
#13909=DIRECTION('',(0.,1.,0.));
#13910=DIRECTION('',(0.,0.,1.));
#13911=DIRECTION('',(0.,-1.,0.));
#13912=DIRECTION('',(0.,0.,-1.));
#13913=DIRECTION('center_axis',(0.,0.,-1.));
#13914=DIRECTION('ref_axis',(1.,0.,0.));
#13915=DIRECTION('',(0.,1.,0.));
#13916=DIRECTION('center_axis',(0.,0.,-1.));
#13917=DIRECTION('ref_axis',(-1.,0.,0.));
#13918=DIRECTION('',(1.,0.,0.));
#13919=DIRECTION('center_axis',(0.,0.,-1.));
#13920=DIRECTION('ref_axis',(1.,0.,0.));
#13921=DIRECTION('',(-1.,0.,0.));
#13922=DIRECTION('center_axis',(0.,0.,1.));
#13923=DIRECTION('ref_axis',(-1.,-4.44089209850063E-15,0.));
#13924=DIRECTION('',(0.,-1.,0.));
#13925=DIRECTION('center_axis',(1.,0.,0.));
#13926=DIRECTION('ref_axis',(0.,0.,-1.));
#13927=DIRECTION('',(0.,0.,-1.));
#13928=DIRECTION('',(0.,-1.,0.));
#13929=DIRECTION('',(0.,0.,1.));
#13930=DIRECTION('',(0.,1.,0.));
#13931=DIRECTION('center_axis',(0.,0.,1.));
#13932=DIRECTION('ref_axis',(-1.,0.,0.));
#13933=DIRECTION('',(0.,-1.,0.));
#13934=DIRECTION('',(1.,0.,0.));
#13935=DIRECTION('center_axis',(0.,0.,-1.));
#13936=DIRECTION('ref_axis',(1.,1.06581410364015E-14,0.));
#13937=DIRECTION('',(-1.,0.,0.));
#13938=DIRECTION('center_axis',(0.,0.,1.));
#13939=DIRECTION('ref_axis',(-1.,0.,0.));
#13940=DIRECTION('',(1.,0.,0.));
#13941=DIRECTION('center_axis',(0.,0.,1.));
#13942=DIRECTION('ref_axis',(1.,0.,0.));
#13943=DIRECTION('',(-1.,0.,0.));
#13944=DIRECTION('',(0.,1.,0.));
#13945=DIRECTION('center_axis',(-1.,0.,0.));
#13946=DIRECTION('ref_axis',(0.,0.,1.));
#13947=DIRECTION('',(0.,0.,1.));
#13948=DIRECTION('',(0.,1.,0.));
#13949=DIRECTION('',(0.,0.,-1.));
#13950=DIRECTION('',(0.,-1.,0.));
#13951=DIRECTION('center_axis',(0.,0.,1.));
#13952=DIRECTION('ref_axis',(-1.,0.,0.));
#13953=DIRECTION('',(0.,1.,0.));
#13954=DIRECTION('center_axis',(0.,0.,1.));
#13955=DIRECTION('ref_axis',(1.,0.,0.));
#13956=DIRECTION('',(-1.,0.,0.));
#13957=DIRECTION('center_axis',(0.,0.,1.));
#13958=DIRECTION('ref_axis',(-1.,0.,0.));
#13959=DIRECTION('',(1.,0.,0.));
#13960=DIRECTION('center_axis',(0.,0.,-1.));
#13961=DIRECTION('ref_axis',(1.,-4.44089209850063E-15,0.));
#13962=DIRECTION('',(0.,-1.,0.));
#13963=DIRECTION('center_axis',(1.,0.,0.));
#13964=DIRECTION('ref_axis',(0.,0.,-1.));
#13965=DIRECTION('',(0.,0.,1.));
#13966=DIRECTION('',(0.,1.,0.));
#13967=DIRECTION('',(0.,0.,-1.));
#13968=DIRECTION('',(0.,-1.,0.));
#13969=DIRECTION('center_axis',(0.,0.,-1.));
#13970=DIRECTION('ref_axis',(-1.,0.,0.));
#13971=DIRECTION('',(1.,0.,0.));
#13972=DIRECTION('center_axis',(0.,0.,-1.));
#13973=DIRECTION('ref_axis',(-1.,0.,0.));
#13974=DIRECTION('',(0.,-1.,0.));
#13975=DIRECTION('center_axis',(0.,0.,-1.));
#13976=DIRECTION('ref_axis',(-1.,0.,0.));
#13977=DIRECTION('',(0.,1.,0.));
#13978=DIRECTION('center_axis',(0.,0.,1.));
#13979=DIRECTION('ref_axis',(-1.,0.,0.));
#13980=DIRECTION('',(-1.,0.,0.));
#13981=DIRECTION('center_axis',(-0.707106781186548,0.,0.707106781186548));
#13982=DIRECTION('ref_axis',(0.,1.,0.));
#13983=DIRECTION('',(-0.707106781186547,0.,-0.707106781186547));
#13984=DIRECTION('',(0.,-1.,0.));
#13985=DIRECTION('',(0.707106781186547,0.,0.707106781186547));
#13986=DIRECTION('',(0.,1.,0.));
#13987=DIRECTION('center_axis',(0.707106781186548,0.,0.707106781186548));
#13988=DIRECTION('ref_axis',(0.,-1.,0.));
#13989=DIRECTION('',(0.707106781186547,0.,-0.707106781186547));
#13990=DIRECTION('',(0.,-1.,0.));
#13991=DIRECTION('',(-0.707106781186547,0.,0.707106781186547));
#13992=DIRECTION('',(0.,1.,0.));
#13993=DIRECTION('center_axis',(-0.707106781186548,0.,-0.707106781186548));
#13994=DIRECTION('ref_axis',(0.,-1.,0.));
#13995=DIRECTION('',(0.707106781186547,0.,-0.707106781186547));
#13996=DIRECTION('',(0.,1.,0.));
#13997=DIRECTION('',(-0.707106781186547,0.,0.707106781186547));
#13998=DIRECTION('',(0.,-1.,0.));
#13999=DIRECTION('center_axis',(0.707106781186548,0.,-0.707106781186548));
#14000=DIRECTION('ref_axis',(0.,1.,0.));
#14001=DIRECTION('',(0.,-1.,0.));
#14002=DIRECTION('',(-0.707106781186547,0.,-0.707106781186547));
#14003=DIRECTION('',(0.,1.,0.));
#14004=DIRECTION('',(0.707106781186547,0.,0.707106781186547));
#14005=DIRECTION('center_axis',(0.,0.,1.));
#14006=DIRECTION('ref_axis',(1.,0.,0.));
#14007=DIRECTION('center_axis',(0.,0.,1.));
#14008=DIRECTION('ref_axis',(1.,0.,0.));
#14009=DIRECTION('center_axis',(1.,0.,0.));
#14010=DIRECTION('ref_axis',(0.,0.,-1.));
#14011=DIRECTION('center_axis',(1.,0.,0.));
#14012=DIRECTION('ref_axis',(0.,0.,-1.));
#14013=DIRECTION('center_axis',(0.,1.,0.));
#14014=DIRECTION('ref_axis',(0.,0.,1.));
#14015=DIRECTION('center_axis',(0.,-1.,0.));
#14016=DIRECTION('ref_axis',(0.,0.,-1.));
#14017=DIRECTION('center_axis',(0.,0.,1.));
#14018=DIRECTION('ref_axis',(1.,0.,0.));
#14019=DIRECTION('center_axis',(0.518508516521689,-0.855072463768117,-4.74660568499161E-15));
#14020=DIRECTION('ref_axis',(0.855072463768117,0.518508516521689,-1.27467223778887E-31));
#14021=DIRECTION('center_axis',(0.,1.,0.));
#14022=DIRECTION('ref_axis',(1.,0.,0.));
#14023=DIRECTION('center_axis',(0.,1.,0.));
#14024=DIRECTION('ref_axis',(1.11022302462516E-14,0.,-1.));
#14025=DIRECTION('center_axis',(0.707106781186545,3.92523114670951E-15,
-0.70710678118655));
#14026=DIRECTION('ref_axis',(0.70710678118655,9.38409251374148E-32,0.707106781186545));
#14027=DIRECTION('center_axis',(1.66533453693773E-14,0.,1.));
#14028=DIRECTION('ref_axis',(-1.,0.,1.66533453693773E-14));
#14029=DIRECTION('center_axis',(0.,1.,0.));
#14030=DIRECTION('ref_axis',(1.,0.,0.));
#14031=DIRECTION('center_axis',(-0.707106781186545,-1.17756934401283E-14,
0.70710678118655));
#14032=DIRECTION('ref_axis',(-0.70710678118655,-2.63935455544261E-31,-0.707106781186545));
#14033=DIRECTION('center_axis',(1.,0.,1.11022302462516E-14));
#14034=DIRECTION('ref_axis',(-1.11022302462516E-14,0.,1.));
#14035=DIRECTION('center_axis',(0.,-1.,0.));
#14036=DIRECTION('ref_axis',(-1.11022302462516E-14,0.,1.));
#14037=DIRECTION('center_axis',(0.,-1.,0.));
#14038=DIRECTION('ref_axis',(0.,0.,-1.));
#14039=DIRECTION('center_axis',(0.,0.,-1.));
#14040=DIRECTION('ref_axis',(1.,0.,0.));
#14041=DIRECTION('center_axis',(0.,0.,-1.));
#14042=DIRECTION('ref_axis',(1.,0.,0.));
#14043=DIRECTION('center_axis',(0.,0.,-1.));
#14044=DIRECTION('ref_axis',(0.924701283533291,-0.380693493813441,0.));
#14045=DIRECTION('center_axis',(0.,0.,1.));
#14046=DIRECTION('ref_axis',(1.,0.,0.));
#14047=DIRECTION('center_axis',(-1.,0.,0.));
#14048=DIRECTION('ref_axis',(0.,0.,1.));
#14049=DIRECTION('center_axis',(0.,1.,0.));
#14050=DIRECTION('ref_axis',(0.,0.,1.));
#14051=DIRECTION('center_axis',(0.,-1.,0.));
#14052=DIRECTION('ref_axis',(0.,0.,-1.));
#14053=DIRECTION('center_axis',(0.707106781186548,0.,-0.707106781186548));
#14054=DIRECTION('ref_axis',(-0.707106781186548,0.,-0.707106781186548));
#14055=DIRECTION('center_axis',(0.707106781186564,0.,-0.707106781186531));
#14056=DIRECTION('ref_axis',(-0.707106781186531,0.,-0.707106781186564));
#14057=DIRECTION('center_axis',(0.,0.,-1.));
#14058=DIRECTION('ref_axis',(-1.,0.,0.));
#14059=DIRECTION('center_axis',(0.,-5.55111512312578E-15,1.));
#14060=DIRECTION('ref_axis',(0.,-1.,-5.55111512312578E-15));
#14061=DIRECTION('center_axis',(0.,-1.,0.));
#14062=DIRECTION('ref_axis',(0.,0.,-1.));
#14063=DIRECTION('center_axis',(0.,1.,0.));
#14064=DIRECTION('ref_axis',(0.,0.,1.));
#14065=DIRECTION('center_axis',(-0.707106781186548,0.,0.707106781186548));
#14066=DIRECTION('ref_axis',(0.707106781186548,0.,0.707106781186548));
#14067=DIRECTION('center_axis',(-0.707106781186553,0.,0.707106781186542));
#14068=DIRECTION('ref_axis',(0.707106781186542,0.,0.707106781186553));
#14069=DIRECTION('center_axis',(0.,0.,1.));
#14070=DIRECTION('ref_axis',(1.,0.,0.));
#14071=DIRECTION('center_axis',(0.,0.,-1.));
#14072=DIRECTION('ref_axis',(-1.,0.,0.));
#14073=DIRECTION('center_axis',(0.,-1.,0.));
#14074=DIRECTION('ref_axis',(0.,0.,-1.));
#14075=DIRECTION('center_axis',(0.,-1.,0.));
#14076=DIRECTION('ref_axis',(0.,0.,-1.));
#14077=DIRECTION('center_axis',(0.,0.,-1.));
#14078=DIRECTION('ref_axis',(-1.,0.,0.));
#14079=DIRECTION('center_axis',(0.,0.,-1.));
#14080=DIRECTION('ref_axis',(-1.,0.,0.));
#14081=DIRECTION('center_axis',(-0.739130434782608,0.673562321079551,0.));
#14082=DIRECTION('ref_axis',(0.673562321079551,0.739130434782608,0.));
#14083=DIRECTION('center_axis',(0.,1.,0.));
#14084=DIRECTION('ref_axis',(1.,0.,0.));
#14085=DIRECTION('center_axis',(1.,-3.33066907387547E-14,0.));
#14086=DIRECTION('ref_axis',(-3.33066907387547E-14,-1.,0.));
#14087=DIRECTION('center_axis',(0.,1.,0.));
#14088=DIRECTION('ref_axis',(1.,0.,0.));
#14089=DIRECTION('center_axis',(0.,1.,0.));
#14090=DIRECTION('ref_axis',(0.,0.,-1.));
#14091=DIRECTION('center_axis',(0.707106781186548,0.,0.707106781186548));
#14092=DIRECTION('ref_axis',(-0.707106781186548,0.,0.707106781186548));
#14093=DIRECTION('center_axis',(0.,1.,0.));
#14094=DIRECTION('ref_axis',(1.,0.,0.));
#14095=DIRECTION('center_axis',(0.,-5.55111512312578E-15,1.));
#14096=DIRECTION('ref_axis',(0.,1.,5.55111512312578E-15));
#14097=DIRECTION('center_axis',(0.,-1.,0.));
#14098=DIRECTION('ref_axis',(0.,0.,-1.));
#14099=DIRECTION('center_axis',(-1.,0.,0.));
#14100=DIRECTION('ref_axis',(0.,0.,-1.));
#14101=DIRECTION('center_axis',(-0.518508516521692,0.855072463768115,0.));
#14102=DIRECTION('ref_axis',(0.855072463768115,0.518508516521692,-5.55111512312579E-15));
#14103=DIRECTION('center_axis',(0.,0.,1.));
#14104=DIRECTION('ref_axis',(1.,0.,0.));
#14105=DIRECTION('center_axis',(-0.797101449275362,0.603845410318832,0.));
#14106=DIRECTION('ref_axis',(-0.603845410318832,-0.797101449275361,0.));
#14107=DIRECTION('center_axis',(1.,0.,0.));
#14108=DIRECTION('ref_axis',(0.,0.,-1.));
#14109=DIRECTION('center_axis',(0.707106781186548,0.,0.707106781186548));
#14110=DIRECTION('ref_axis',(0.707106781186548,0.,-0.707106781186548));
#14111=DIRECTION('center_axis',(0.707106781186545,-3.92523114670945E-15,
0.70710678118655));
#14112=DIRECTION('ref_axis',(0.70710678118655,3.86675578882201E-31,-0.707106781186545));
#14113=DIRECTION('center_axis',(0.,-1.,0.));
#14114=DIRECTION('ref_axis',(0.,0.,-1.));
#14115=DIRECTION('center_axis',(0.,1.,0.));
#14116=DIRECTION('ref_axis',(0.,0.,1.));
#14117=DIRECTION('center_axis',(0.,0.,-1.));
#14118=DIRECTION('ref_axis',(-1.,0.,0.));
#14119=DIRECTION('center_axis',(-5.55111512312578E-15,0.,1.));
#14120=DIRECTION('ref_axis',(1.,0.,5.55111512312578E-15));
#14121=DIRECTION('center_axis',(-1.,0.,0.));
#14122=DIRECTION('ref_axis',(0.,0.,1.));
#14123=DIRECTION('center_axis',(0.,0.,1.));
#14124=DIRECTION('ref_axis',(1.,0.,0.));
#14125=DIRECTION('center_axis',(0.,0.,-1.));
#14126=DIRECTION('ref_axis',(1.,0.,0.));
#14127=DIRECTION('center_axis',(0.,1.,0.));
#14128=DIRECTION('ref_axis',(1.,0.,0.));
#14129=DIRECTION('center_axis',(0.,1.,0.));
#14130=DIRECTION('ref_axis',(1.11022302462516E-14,0.,-1.));
#14131=DIRECTION('center_axis',(1.,0.,1.11022302462516E-14));
#14132=DIRECTION('ref_axis',(-1.11022302462516E-14,0.,1.));
#14133=DIRECTION('center_axis',(0.,1.,0.));
#14134=DIRECTION('ref_axis',(1.,0.,0.));
#14135=DIRECTION('center_axis',(0.707106781186545,-3.92523114670945E-15,
0.70710678118655));
#14136=DIRECTION('ref_axis',(-0.70710678118655,-3.86675578882201E-31,0.707106781186545));
#14137=DIRECTION('center_axis',(0.,0.,-1.));
#14138=DIRECTION('ref_axis',(-1.,0.,0.));
#14139=DIRECTION('center_axis',(0.,0.,-1.));
#14140=DIRECTION('ref_axis',(-1.,0.,0.));
#14141=DIRECTION('center_axis',(-1.,0.,0.));
#14142=DIRECTION('ref_axis',(0.,0.,1.));
#14143=DIRECTION('center_axis',(0.,-1.,0.));
#14144=DIRECTION('ref_axis',(0.,0.,-1.));
#14145=DIRECTION('center_axis',(0.,1.,0.));
#14146=DIRECTION('ref_axis',(0.,0.,1.));
#14147=DIRECTION('center_axis',(-0.707106781186548,0.,-0.707106781186548));
#14148=DIRECTION('ref_axis',(-0.707106781186548,0.,0.707106781186548));
#14149=DIRECTION('center_axis',(0.707106781186553,0.,0.707106781186542));
#14150=DIRECTION('ref_axis',(0.707106781186542,0.,-0.707106781186553));
#14151=DIRECTION('center_axis',(-1.,0.,0.));
#14152=DIRECTION('ref_axis',(0.,0.,1.));
#14153=DIRECTION('center_axis',(1.,0.,0.));
#14154=DIRECTION('ref_axis',(0.,0.,-1.));
#14155=DIRECTION('center_axis',(0.,0.,-1.));
#14156=DIRECTION('ref_axis',(0.924701283533291,-0.380693493813441,0.));
#14157=DIRECTION('center_axis',(0.797101449275362,-0.603845410318832,0.));
#14158=DIRECTION('ref_axis',(-0.603845410318832,-0.797101449275361,0.));
#14159=DIRECTION('center_axis',(0.,1.,0.));
#14160=DIRECTION('ref_axis',(1.,0.,0.));
#14161=DIRECTION('center_axis',(1.,0.,0.));
#14162=DIRECTION('ref_axis',(0.,0.,1.));
#14163=DIRECTION('center_axis',(0.,-1.,0.));
#14164=DIRECTION('ref_axis',(0.,0.,-1.));
#14165=DIRECTION('center_axis',(0.,0.,-1.));
#14166=DIRECTION('ref_axis',(1.,0.,0.));
#14167=DIRECTION('center_axis',(0.,1.,0.));
#14168=DIRECTION('ref_axis',(0.,0.,-1.));
#14169=DIRECTION('center_axis',(0.,0.,1.));
#14170=DIRECTION('ref_axis',(1.,0.,0.));
#14171=DIRECTION('center_axis',(0.739130434782608,-0.673562321079551,0.));
#14172=DIRECTION('ref_axis',(0.673562321079551,0.739130434782608,0.));
#14173=DIRECTION('center_axis',(1.,0.,0.));
#14174=DIRECTION('ref_axis',(0.,0.,-1.));
#14175=DIRECTION('center_axis',(0.,0.,1.));
#14176=DIRECTION('ref_axis',(1.,0.,0.));
#14177=DIRECTION('center_axis',(0.,0.,-1.));
#14178=DIRECTION('ref_axis',(-1.,0.,0.));
#14179=DIRECTION('center_axis',(0.,1.,0.));
#14180=DIRECTION('ref_axis',(0.,0.,1.));
#14181=DIRECTION('center_axis',(0.,0.,-1.));
#14182=DIRECTION('ref_axis',(-1.,0.,0.));
#14183=DIRECTION('center_axis',(0.518508516521689,-0.855072463768117,-4.74660568499161E-15));
#14184=DIRECTION('ref_axis',(0.855072463768117,0.518508516521689,-1.27467223778887E-31));
#14185=DIRECTION('center_axis',(0.,0.,1.));
#14186=DIRECTION('ref_axis',(-1.,0.,0.));
#14187=DIRECTION('center_axis',(0.,-1.,0.));
#14188=DIRECTION('ref_axis',(0.,0.,-1.));
#14189=DIRECTION('center_axis',(-1.,0.,0.));
#14190=DIRECTION('ref_axis',(0.,0.,-1.));
#14191=DIRECTION('center_axis',(0.,1.,0.));
#14192=DIRECTION('ref_axis',(0.,0.,-1.));
#14193=DIRECTION('center_axis',(0.,0.,-1.));
#14194=DIRECTION('ref_axis',(1.,0.,0.));
#14195=DIRECTION('center_axis',(0.,0.,-1.));
#14196=DIRECTION('ref_axis',(0.924701283533291,-0.380693493813441,0.));
#14197=DIRECTION('center_axis',(1.,0.,0.));
#14198=DIRECTION('ref_axis',(0.,0.,-1.));
#14199=DIRECTION('center_axis',(0.,-1.,0.));
#14200=DIRECTION('ref_axis',(0.,0.,-1.));
#14201=DIRECTION('center_axis',(0.,0.,-1.));
#14202=DIRECTION('ref_axis',(-1.,0.,0.));
#14203=DIRECTION('center_axis',(0.,0.,-1.));
#14204=DIRECTION('ref_axis',(-1.,0.,0.));
#14205=DIRECTION('center_axis',(-0.518508516521693,0.855072463768114,0.));
#14206=DIRECTION('ref_axis',(0.855072463768114,0.518508516521693,0.));
#14207=DIRECTION('center_axis',(0.,0.,-1.));
#14208=DIRECTION('ref_axis',(-1.,0.,0.));
#14209=DIRECTION('center_axis',(0.,1.,0.));
#14210=DIRECTION('ref_axis',(1.,0.,0.));
#14211=DIRECTION('center_axis',(-0.707106781186559,0.,-0.707106781186536));
#14212=DIRECTION('ref_axis',(0.707106781186536,0.,-0.707106781186559));
#14213=DIRECTION('center_axis',(0.,1.,0.));
#14214=DIRECTION('ref_axis',(0.,0.,-1.));
#14215=DIRECTION('center_axis',(0.,1.11022302462516E-14,1.));
#14216=DIRECTION('ref_axis',(0.,1.,-1.11022302462516E-14));
#14217=DIRECTION('center_axis',(-0.707106781186548,0.,-0.707106781186548));
#14218=DIRECTION('ref_axis',(-0.707106781186548,0.,0.707106781186548));
#14219=DIRECTION('center_axis',(0.707106781186545,-3.92523114670939E-15,
0.70710678118655));
#14220=DIRECTION('ref_axis',(0.70710678118655,-2.00573270066562E-31,-0.707106781186545));
#14221=DIRECTION('center_axis',(-0.707106781186559,0.,-0.707106781186536));
#14222=DIRECTION('ref_axis',(-0.707106781186536,0.,0.707106781186559));
#14223=DIRECTION('center_axis',(0.,1.,0.));
#14224=DIRECTION('ref_axis',(0.,0.,1.));
#14225=DIRECTION('center_axis',(0.,1.,0.));
#14226=DIRECTION('ref_axis',(0.,0.,1.));
#14227=DIRECTION('center_axis',(0.,0.,-1.));
#14228=DIRECTION('ref_axis',(-1.,0.,0.));
#14229=DIRECTION('center_axis',(0.,0.,1.));
#14230=DIRECTION('ref_axis',(1.,0.,0.));
#14231=DIRECTION('center_axis',(0.707106781186548,0.,0.707106781186548));
#14232=DIRECTION('ref_axis',(0.707106781186548,0.,-0.707106781186548));
#14233=DIRECTION('center_axis',(-0.707106781186545,-3.92523114670945E-15,
-0.70710678118655));
#14234=DIRECTION('ref_axis',(-0.70710678118655,3.86675578882201E-31,0.707106781186545));
#14235=DIRECTION('center_axis',(0.,1.,0.));
#14236=DIRECTION('ref_axis',(0.,0.,1.));
#14237=DIRECTION('center_axis',(0.,1.,0.));
#14238=DIRECTION('ref_axis',(0.,0.,1.));
#14239=DIRECTION('center_axis',(0.,-1.,0.));
#14240=DIRECTION('ref_axis',(0.,0.,-1.));
#14241=DIRECTION('center_axis',(0.,1.,0.));
#14242=DIRECTION('ref_axis',(1.,0.,0.));
#14243=DIRECTION('center_axis',(-1.,1.11022302462516E-14,0.));
#14244=DIRECTION('ref_axis',(1.11022302462516E-14,1.,0.));
#14245=DIRECTION('center_axis',(0.,1.,0.));
#14246=DIRECTION('ref_axis',(1.,0.,0.));
#14247=DIRECTION('center_axis',(-1.11022302462516E-14,0.,1.));
#14248=DIRECTION('ref_axis',(-1.,0.,-1.11022302462516E-14));
#14249=DIRECTION('center_axis',(0.,1.,0.));
#14250=DIRECTION('ref_axis',(1.,0.,0.));
#14251=DIRECTION('center_axis',(-0.707106781186545,0.,0.70710678118655));
#14252=DIRECTION('ref_axis',(-0.70710678118655,0.,-0.707106781186545));
#14253=DIRECTION('center_axis',(0.,1.,0.));
#14254=DIRECTION('ref_axis',(0.,0.,-1.));
#14255=DIRECTION('center_axis',(0.,1.,0.));
#14256=DIRECTION('ref_axis',(1.,0.,0.));
#14257=DIRECTION('center_axis',(-1.,0.,-1.11022302462516E-14));
#14258=DIRECTION('ref_axis',(1.11022302462516E-14,0.,-1.));
#14259=DIRECTION('center_axis',(-1.,0.,0.));
#14260=DIRECTION('ref_axis',(0.,0.,1.));
#14261=DIRECTION('center_axis',(0.,0.,-1.));
#14262=DIRECTION('ref_axis',(-1.,0.,0.));
#14263=DIRECTION('center_axis',(0.,-1.11022302462516E-14,1.));
#14264=DIRECTION('ref_axis',(0.,-1.,-1.11022302462516E-14));
#14265=DIRECTION('center_axis',(0.,1.,0.));
#14266=DIRECTION('ref_axis',(0.,0.,1.));
#14267=DIRECTION('center_axis',(0.,1.,0.));
#14268=DIRECTION('ref_axis',(0.,0.,1.));
#14269=DIRECTION('center_axis',(0.707106781186548,0.,-0.707106781186548));
#14270=DIRECTION('ref_axis',(-0.707106781186548,0.,-0.707106781186548));
#14271=DIRECTION('center_axis',(-0.707106781186553,0.,0.707106781186542));
#14272=DIRECTION('ref_axis',(0.707106781186542,0.,0.707106781186553));
#14273=DIRECTION('center_axis',(1.,0.,0.));
#14274=DIRECTION('ref_axis',(0.,0.,-1.));
#14275=DIRECTION('center_axis',(0.,0.,1.));
#14276=DIRECTION('ref_axis',(1.,0.,0.));
#14277=DIRECTION('center_axis',(0.797101449275362,0.603845410318832,0.));
#14278=DIRECTION('ref_axis',(-0.603845410318832,0.797101449275361,0.));
#14279=DIRECTION('center_axis',(-0.739130434782608,-0.673562321079551,0.));
#14280=DIRECTION('ref_axis',(0.673562321079551,-0.739130434782608,0.));
#14281=DIRECTION('center_axis',(0.,1.,0.));
#14282=DIRECTION('ref_axis',(1.,0.,0.));
#14283=DIRECTION('center_axis',(-0.707106781186539,0.,0.707106781186556));
#14284=DIRECTION('ref_axis',(-0.707106781186556,0.,-0.707106781186539));
#14285=DIRECTION('center_axis',(0.,1.,0.));
#14286=DIRECTION('ref_axis',(1.,0.,0.));
#14287=DIRECTION('center_axis',(-1.,-1.11022302462516E-14,0.));
#14288=DIRECTION('ref_axis',(-1.11022302462516E-14,1.,0.));
#14289=DIRECTION('center_axis',(0.,1.,0.));
#14290=DIRECTION('ref_axis',(0.,0.,-1.));
#14291=DIRECTION('center_axis',(0.,0.,-1.));
#14292=DIRECTION('ref_axis',(1.,3.33066907387547E-14,0.));
#14293=DIRECTION('center_axis',(-0.707106781186548,0.,0.707106781186548));
#14294=DIRECTION('ref_axis',(0.707106781186548,0.,0.707106781186548));
#14295=DIRECTION('center_axis',(-0.707106781186545,1.96261557335471E-14,
0.70710678118655));
#14296=DIRECTION('ref_axis',(0.70710678118655,-4.24411161318039E-31,0.707106781186545));
#14297=DIRECTION('center_axis',(0.,-1.,0.));
#14298=DIRECTION('ref_axis',(0.,0.,-1.));
#14299=DIRECTION('center_axis',(0.,1.,0.));
#14300=DIRECTION('ref_axis',(0.,0.,1.));
#14301=DIRECTION('center_axis',(-1.,0.,0.));
#14302=DIRECTION('ref_axis',(0.,0.,1.));
#14303=DIRECTION('center_axis',(0.,0.,-1.));
#14304=DIRECTION('ref_axis',(-1.,0.,0.));
#14305=DIRECTION('center_axis',(0.,0.,-1.));
#14306=DIRECTION('ref_axis',(-1.,0.,0.));
#14307=DIRECTION('center_axis',(0.,1.,0.));
#14308=DIRECTION('ref_axis',(1.,0.,0.));
#14309=DIRECTION('center_axis',(-1.,5.55111512312578E-15,0.));
#14310=DIRECTION('ref_axis',(5.55111512312578E-15,1.,0.));
#14311=DIRECTION('center_axis',(-0.710144927536232,-0.704055524724123,3.94209624685744E-15));
#14312=DIRECTION('ref_axis',(-0.704055524724123,0.710144927536232,2.77555756156289E-15));
#14313=DIRECTION('center_axis',(0.,1.,0.));
#14314=DIRECTION('ref_axis',(1.,0.,0.));
#14315=DIRECTION('center_axis',(-1.,0.,-2.22044604925031E-14));
#14316=DIRECTION('ref_axis',(2.22044604925031E-14,0.,-1.));
#14317=DIRECTION('center_axis',(-0.797101449275362,-0.603845410318832,0.));
#14318=DIRECTION('ref_axis',(-0.603845410318832,0.797101449275361,0.));
#14319=DIRECTION('center_axis',(0.,0.,1.));
#14320=DIRECTION('ref_axis',(1.,0.,0.));
#14321=DIRECTION('center_axis',(-0.518508516521693,-0.855072463768114,0.));
#14322=DIRECTION('ref_axis',(0.855072463768114,-0.518508516521693,0.));
#14323=DIRECTION('center_axis',(0.,-1.,0.));
#14324=DIRECTION('ref_axis',(0.,0.,-1.));
#14325=DIRECTION('center_axis',(0.,-1.,0.));
#14326=DIRECTION('ref_axis',(0.,0.,1.));
#14327=DIRECTION('center_axis',(1.,0.,0.));
#14328=DIRECTION('ref_axis',(0.,0.,-1.));
#14329=DIRECTION('center_axis',(-1.,0.,0.));
#14330=DIRECTION('ref_axis',(0.,0.,1.));
#14331=DIRECTION('center_axis',(1.,0.,0.));
#14332=DIRECTION('ref_axis',(0.,0.,-1.));
#14333=DIRECTION('center_axis',(0.,0.,1.));
#14334=DIRECTION('ref_axis',(1.,0.,0.));
#14335=DIRECTION('center_axis',(-0.739130434782608,-0.673562321079551,0.));
#14336=DIRECTION('ref_axis',(0.673562321079551,-0.739130434782608,0.));
#14337=DIRECTION('center_axis',(0.,0.,-1.));
#14338=DIRECTION('ref_axis',(1.,0.,0.));
#14339=DIRECTION('center_axis',(0.,1.,0.));
#14340=DIRECTION('ref_axis',(0.,0.,1.));
#14341=DIRECTION('center_axis',(0.,0.,-1.));
#14342=DIRECTION('ref_axis',(1.,0.,0.));
#14343=DIRECTION('center_axis',(0.,0.,-1.));
#14344=DIRECTION('ref_axis',(-1.,0.,0.));
#14345=DIRECTION('center_axis',(0.,0.,-1.));
#14346=DIRECTION('ref_axis',(-1.,0.,0.));
#14347=DIRECTION('center_axis',(0.,1.,0.));
#14348=DIRECTION('ref_axis',(0.,0.,1.));
#14349=DIRECTION('center_axis',(0.,-1.,0.));
#14350=DIRECTION('ref_axis',(0.,0.,1.));
#14351=DIRECTION('center_axis',(0.,0.,1.));
#14352=DIRECTION('ref_axis',(1.,0.,0.));
#14353=DIRECTION('center_axis',(0.,0.,-1.));
#14354=DIRECTION('ref_axis',(-1.,0.,0.));
#14355=DIRECTION('center_axis',(1.,0.,0.));
#14356=DIRECTION('ref_axis',(0.,0.,-1.));
#14357=DIRECTION('center_axis',(1.,0.,5.55111512312578E-15));
#14358=DIRECTION('ref_axis',(5.55111512312578E-15,0.,-1.));
#14359=DIRECTION('center_axis',(-1.,0.,0.));
#14360=DIRECTION('ref_axis',(0.,0.,1.));
#14361=DIRECTION('center_axis',(0.518508516521693,0.855072463768114,1.00999525007457E-15));
#14362=DIRECTION('ref_axis',(0.855072463768114,-0.518508516521693,-8.14669008397628E-32));
#14363=DIRECTION('center_axis',(0.,1.,0.));
#14364=DIRECTION('ref_axis',(0.,0.,1.));
#14365=DIRECTION('center_axis',(1.,0.,0.));
#14366=DIRECTION('ref_axis',(0.,0.,1.));
#14367=DIRECTION('center_axis',(0.,1.,0.));
#14368=DIRECTION('ref_axis',(0.,0.,1.));
#14369=DIRECTION('center_axis',(0.,0.,1.));
#14370=DIRECTION('ref_axis',(-1.,0.,0.));
#14371=DIRECTION('center_axis',(0.,1.,0.));
#14372=DIRECTION('ref_axis',(0.,0.,1.));
#14373=DIRECTION('center_axis',(0.,1.,0.));
#14374=DIRECTION('ref_axis',(1.,0.,0.));
#14375=DIRECTION('center_axis',(-0.710144927536229,-0.704055524724125,0.));
#14376=DIRECTION('ref_axis',(-0.704055524724125,0.710144927536229,0.));
#14377=DIRECTION('center_axis',(0.,0.,1.));
#14378=DIRECTION('ref_axis',(1.,0.,0.));
#14379=DIRECTION('center_axis',(0.710144927536229,0.704055524724125,0.));
#14380=DIRECTION('ref_axis',(-0.704055524724125,0.710144927536229,0.));
#14381=DIRECTION('center_axis',(-1.,0.,0.));
#14382=DIRECTION('ref_axis',(0.,0.,1.));
#14383=DIRECTION('center_axis',(1.,0.,5.55111512312578E-15));
#14384=DIRECTION('ref_axis',(5.55111512312578E-15,0.,-1.));
#14385=DIRECTION('center_axis',(0.,0.,1.));
#14386=DIRECTION('ref_axis',(1.,0.,0.));
#14387=DIRECTION('center_axis',(0.,0.,1.));
#14388=DIRECTION('ref_axis',(1.,0.,0.));
#14389=DIRECTION('center_axis',(0.,1.,0.));
#14390=DIRECTION('ref_axis',(0.,0.,1.));
#14391=DIRECTION('center_axis',(0.,0.,-1.));
#14392=DIRECTION('ref_axis',(-1.,0.,0.));
#14393=DIRECTION('center_axis',(-0.518508516521689,-0.855072463768117,4.74660568499161E-15));
#14394=DIRECTION('ref_axis',(0.855072463768117,-0.518508516521689,-1.27467223778887E-31));
#14395=DIRECTION('center_axis',(0.,1.,0.));
#14396=DIRECTION('ref_axis',(1.,0.,0.));
#14397=DIRECTION('center_axis',(0.,1.,0.));
#14398=DIRECTION('ref_axis',(0.,0.,1.));
#14399=DIRECTION('center_axis',(1.,0.,0.));
#14400=DIRECTION('ref_axis',(0.,0.,1.));
#14401=DIRECTION('center_axis',(0.,1.,0.));
#14402=DIRECTION('ref_axis',(0.,0.,1.));
#14403=DIRECTION('center_axis',(0.,0.,1.));
#14404=DIRECTION('ref_axis',(-1.,0.,0.));
#14405=DIRECTION('center_axis',(-1.,0.,0.));
#14406=DIRECTION('ref_axis',(0.,0.,1.));
#14407=DIRECTION('center_axis',(1.,-5.55111512312578E-15,0.));
#14408=DIRECTION('ref_axis',(5.55111512312578E-15,1.,0.));
#14409=DIRECTION('center_axis',(0.,-1.,0.));
#14410=DIRECTION('ref_axis',(0.,0.,-1.));
#14411=DIRECTION('center_axis',(0.,0.,-1.));
#14412=DIRECTION('ref_axis',(-1.,0.,0.));
#14413=DIRECTION('center_axis',(0.,0.,1.));
#14414=DIRECTION('ref_axis',(1.,0.,0.));
#14415=DIRECTION('center_axis',(0.,1.,0.));
#14416=DIRECTION('ref_axis',(1.,0.,0.));
#14417=DIRECTION('center_axis',(-0.710144927536232,-0.704055524724123,3.94209624685744E-15));
#14418=DIRECTION('ref_axis',(-0.704055524724123,0.710144927536232,2.77555756156289E-15));
#14419=DIRECTION('center_axis',(0.518508516521693,0.855072463768114,0.));
#14420=DIRECTION('ref_axis',(0.855072463768114,-0.518508516521693,0.));
#14421=DIRECTION('center_axis',(0.,0.,-1.));
#14422=DIRECTION('ref_axis',(-1.,0.,0.));
#16754=CARTESIAN_POINT('',(0.,0.,0.));
#16755=CARTESIAN_POINT('Origin',(0.,0.,115.));
#16756=CARTESIAN_POINT('',(160.,1.95943487863577E-14,-45.));
#16757=CARTESIAN_POINT('',(160.,-1.95943487863576E-14,-95.));
#16758=CARTESIAN_POINT('',(160.,-1.95943487863576E-14,115.));
#16759=CARTESIAN_POINT('',(56.5922444183314,149.657334840949,-95.));
#16760=CARTESIAN_POINT('Ctrl Pts',(56.5922444183314,149.657334840949,-95.));
#16761=CARTESIAN_POINT('Ctrl Pts',(60.5462378465639,148.162150106055,-95.));
#16762=CARTESIAN_POINT('Ctrl Pts',(64.4081265946212,146.52305102292,-94.8681994144769));
#16763=CARTESIAN_POINT('Ctrl Pts',(71.9578017024522,142.966730488755,-94.3871141013997));
#16764=CARTESIAN_POINT('Ctrl Pts',(75.6455459182189,141.049479319923,-94.0375811330598));
#16765=CARTESIAN_POINT('Ctrl Pts',(82.8520896158476,136.940627572589,-93.1507035872263));
#16766=CARTESIAN_POINT('Ctrl Pts',(86.3708709116552,134.74901877956,-92.6132279142068));
#16767=CARTESIAN_POINT('Ctrl Pts',(91.5232508355409,131.254717658139,-91.6807717500904));
#16768=CARTESIAN_POINT('Ctrl Pts',(93.2197161772174,130.055428691622,-91.3488437646329));
#16769=CARTESIAN_POINT('Ctrl Pts',(96.5704689047943,127.58712533728,-90.6445107692907));
#16770=CARTESIAN_POINT('Ctrl Pts',(98.2139345505394,126.326078432424,-90.2743825546963));
#16771=CARTESIAN_POINT('Ctrl Pts',(103.050070362074,122.465109833053,-89.1144758355367));
#16772=CARTESIAN_POINT('Ctrl Pts',(106.149349251733,119.786980782129,-88.2752185542421));
#16773=CARTESIAN_POINT('Ctrl Pts',(112.10933354305,114.228290909029,-86.4808050839628));
#16774=CARTESIAN_POINT('Ctrl Pts',(114.970003636752,111.347714259159,-85.5255886134343));
#16775=CARTESIAN_POINT('Ctrl Pts',(120.458203679568,105.386129890351,-83.5098605627197));
#16776=CARTESIAN_POINT('Ctrl Pts',(123.085719078493,102.305118804237,-82.4493145108988));
#16777=CARTESIAN_POINT('Ctrl Pts',(126.22481525846,98.3276308388503,-81.0620110399452));
#16778=CARTESIAN_POINT('Ctrl Pts',(126.845358313088,97.5258134181074,-80.7814609309442));
#16779=CARTESIAN_POINT('Ctrl Pts',(128.071857893764,95.9094803660136,-80.2142555183395));
#16780=CARTESIAN_POINT('Ctrl Pts',(128.677777212601,95.0949724534044,-79.9276008926568));
#16781=CARTESIAN_POINT('Ctrl Pts',(130.466680836712,92.6420084443857,-79.0620127301409));
#16782=CARTESIAN_POINT('Ctrl Pts',(131.623259690082,90.990947097925,-78.4763506491345));
#16783=CARTESIAN_POINT('Ctrl Pts',(137.230368463351,82.658242752523,-75.5075253594053));
#16784=CARTESIAN_POINT('Ctrl Pts',(141.156885196578,75.7456678635037,-73.0041701646379));
#16785=CARTESIAN_POINT('Ctrl Pts',(146.247760030425,65.0173884103724,-69.0861440470581));
#16786=CARTESIAN_POINT('Ctrl Pts',(147.810909187017,61.3811442891731,-67.7527018640001));
#16787=CARTESIAN_POINT('Ctrl Pts',(149.954354213166,55.8356435419837,-65.7130763478));
#16788=CARTESIAN_POINT('Ctrl Pts',(150.635252756495,53.9719392331638,-65.0266124141299));
#16789=CARTESIAN_POINT('Ctrl Pts',(151.605820654521,51.1533238711764,-63.9871451260196));
#16790=CARTESIAN_POINT('Ctrl Pts',(151.921076217439,50.2092866733786,-63.6387848556078));
#16791=CARTESIAN_POINT('Ctrl Pts',(152.532516926856,48.319945646416,-62.9412088896887));
#16792=CARTESIAN_POINT('Ctrl Pts',(152.828934942228,47.3740047564605,-62.5917585364604));
#16793=CARTESIAN_POINT('Ctrl Pts',(155.413776340098,38.8491671355886,-59.4409236358264));
#16794=CARTESIAN_POINT('Ctrl Pts',(157.125117056469,31.1910647608737,-56.5995154310153));
#16795=CARTESIAN_POINT('Ctrl Pts',(158.84500741576,19.5846841133227,-52.2866203497387));
#16796=CARTESIAN_POINT('Ctrl Pts',(159.276491887656,15.6959483595113,-50.8404415216121));
#16797=CARTESIAN_POINT('Ctrl Pts',(159.709623647027,9.83244782649476,-48.6590509514606));
#16798=CARTESIAN_POINT('Ctrl Pts',(159.818281747996,7.87287668664235,-47.9298972382464));
#16799=CARTESIAN_POINT('Ctrl Pts',(159.927179576913,4.92580700241418,-46.8331941701413));
#16800=CARTESIAN_POINT('Ctrl Pts',(159.968102560764,3.45034341369313,-46.2840992857951));
#16801=CARTESIAN_POINT('Ctrl Pts',(159.992025024361,1.72556508603403,-45.6421992563854));
#16802=CARTESIAN_POINT('Ctrl Pts',(159.997154300886,0.985641455265653,-45.3668240670506));
#16803=CARTESIAN_POINT('Ctrl Pts',(159.99943317645,0.492195768543,-45.1831795774147));
#16804=CARTESIAN_POINT('Ctrl Pts',(160.,0.244267011806123,-45.0909083946827));
#16805=CARTESIAN_POINT('Ctrl Pts',(160.,1.95943487863577E-14,-45.));
#16806=CARTESIAN_POINT('Origin',(0.,0.,-95.));
#16807=CARTESIAN_POINT('Origin',(0.,0.,-102.5));
#16808=CARTESIAN_POINT('',(170.,2.0818995585505E-14,-102.5));
#16809=CARTESIAN_POINT('',(-170.,-2.0818995585505E-14,-102.5));
#16810=CARTESIAN_POINT('Origin',(0.,0.,-102.5));
#16811=CARTESIAN_POINT('Origin',(0.,0.,-102.5));
#16812=CARTESIAN_POINT('',(-167.5,-2.05128338857182E-14,-105.));
#16813=CARTESIAN_POINT('Origin',(-167.5,-2.05128338857182E-14,-102.5));
#16814=CARTESIAN_POINT('Origin',(0.,0.,-105.));
#16815=CARTESIAN_POINT('Origin',(121.449578014911,-122.5,115.));
#16816=CARTESIAN_POINT('',(121.449578014911,-125.,32.5));
#16817=CARTESIAN_POINT('',(119.689439203101,-120.724637681159,32.5));
#16818=CARTESIAN_POINT('Origin',(121.449578014911,-122.5,32.5));
#16819=CARTESIAN_POINT('',(121.449578014911,-125.,-32.5));
#16820=CARTESIAN_POINT('',(121.449578014911,-125.,85.));
#16821=CARTESIAN_POINT('',(119.689439203101,-120.724637681159,-32.5));
#16822=CARTESIAN_POINT('Origin',(121.449578014911,-122.5,-32.5));
#16823=CARTESIAN_POINT('',(119.689439203101,-120.724637681159,115.));
#16824=CARTESIAN_POINT('Origin',(121.449578014911,-122.5,115.));
#16825=CARTESIAN_POINT('',(119.689439203101,-120.724637681159,82.5));
#16826=CARTESIAN_POINT('',(118.949578014911,-122.5,82.5));
#16827=CARTESIAN_POINT('Origin',(121.449578014911,-122.5,82.5));
#16828=CARTESIAN_POINT('',(121.449578014911,-125.,82.5));
#16829=CARTESIAN_POINT('Origin',(121.449578014911,-122.5,82.5));
#16830=CARTESIAN_POINT('',(121.449578014911,-125.,49.5));
#16831=CARTESIAN_POINT('',(121.449578014911,-125.,85.));
#16832=CARTESIAN_POINT('',(119.689439203101,-120.724637681159,49.5));
#16833=CARTESIAN_POINT('Origin',(121.449578014911,-122.5,49.5));
#16834=CARTESIAN_POINT('',(119.689439203101,-120.724637681159,115.));
#16835=CARTESIAN_POINT('Origin',(121.449578014911,-122.5,115.));
#16836=CARTESIAN_POINT('',(121.449578014911,-125.,-49.5));
#16837=CARTESIAN_POINT('',(119.689439203101,-120.724637681159,-49.5));
#16838=CARTESIAN_POINT('Origin',(121.449578014911,-122.5,-49.5));
#16839=CARTESIAN_POINT('',(121.449578014911,-125.,-82.5));
#16840=CARTESIAN_POINT('',(121.449578014911,-125.,85.));
#16841=CARTESIAN_POINT('',(119.689439203101,-120.724637681159,-82.5));
#16842=CARTESIAN_POINT('Origin',(121.449578014911,-122.5,-82.5));
#16843=CARTESIAN_POINT('',(119.689439203101,-120.724637681159,115.));
#16844=CARTESIAN_POINT('Origin',(-121.449578014911,-122.5,49.5));
#16845=CARTESIAN_POINT('',(-121.449578014911,-122.5,47.));
#16846=CARTESIAN_POINT('',(-119.689439203101,-120.724637681159,49.5));
#16847=CARTESIAN_POINT('Origin',(-121.449578014911,-122.5,49.5));
#16848=CARTESIAN_POINT('',(-121.449578014911,-125.,49.5));
#16849=CARTESIAN_POINT('Origin',(-121.449578014911,-122.5,49.5));
#16850=CARTESIAN_POINT('Origin',(-121.449578014911,-122.5,49.5));
#16851=CARTESIAN_POINT('Origin',(-121.449578014911,-122.5,32.5));
#16852=CARTESIAN_POINT('',(-119.689439203101,-120.724637681159,32.5));
#16853=CARTESIAN_POINT('',(-121.449578014911,-125.,32.5));
#16854=CARTESIAN_POINT('Origin',(-121.449578014911,-122.5,32.5));
#16855=CARTESIAN_POINT('',(-121.449578014911,-122.5,35.));
#16856=CARTESIAN_POINT('Origin',(-121.449578014911,-122.5,32.5));
#16857=CARTESIAN_POINT('Origin',(-121.449578014911,-122.5,32.5));
#16858=CARTESIAN_POINT('Origin',(-121.449578014911,-122.5,-32.5));
#16859=CARTESIAN_POINT('',(-119.689439203101,-120.724637681159,-32.5));
#16860=CARTESIAN_POINT('',(-121.449578014911,-122.5,-35.));
#16861=CARTESIAN_POINT('Origin',(-121.449578014911,-122.5,-32.5));
#16862=CARTESIAN_POINT('',(-121.449578014911,-125.,-32.5));
#16863=CARTESIAN_POINT('Origin',(-121.449578014911,-122.5,-32.5));
#16864=CARTESIAN_POINT('Origin',(-121.449578014911,-122.5,-32.5));
#16865=CARTESIAN_POINT('Origin',(-121.449578014911,-122.5,-49.5));
#16866=CARTESIAN_POINT('',(-121.449578014911,-125.,-49.5));
#16867=CARTESIAN_POINT('',(-119.689439203101,-120.724637681159,-49.5));
#16868=CARTESIAN_POINT('Origin',(-121.449578014911,-122.5,-49.5));
#16869=CARTESIAN_POINT('',(-121.449578014911,-122.5,-47.));
#16870=CARTESIAN_POINT('Origin',(-121.449578014911,-122.5,-49.5));
#16871=CARTESIAN_POINT('Origin',(-121.449578014911,-122.5,-49.5));
#16872=CARTESIAN_POINT('Origin',(0.,0.,124.));
#16873=CARTESIAN_POINT('',(-194.,-2.37581479034587E-14,125.));
#16874=CARTESIAN_POINT('Origin',(0.,0.,125.));
#16875=CARTESIAN_POINT('',(-195.,-2.38806125833734E-14,124.));
#16876=CARTESIAN_POINT('Origin',(-194.,-2.37581479034587E-14,124.));
#16877=CARTESIAN_POINT('',(195.,2.38806125833734E-14,124.));
#16878=CARTESIAN_POINT('Origin',(0.,0.,124.));
#16879=CARTESIAN_POINT('Origin',(0.,0.,124.));
#16880=CARTESIAN_POINT('Origin',(0.,0.,116.));
#16881=CARTESIAN_POINT('',(195.,2.38806125833734E-14,116.));
#16882=CARTESIAN_POINT('',(-195.,-2.38806125833734E-14,116.));
#16883=CARTESIAN_POINT('Origin',(0.,0.,116.));
#16884=CARTESIAN_POINT('Origin',(0.,0.,116.));
#16885=CARTESIAN_POINT('',(-194.,-2.37581479034587E-14,115.));
#16886=CARTESIAN_POINT('Origin',(-194.,-2.37581479034587E-14,116.));
#16887=CARTESIAN_POINT('Origin',(0.,0.,115.));
#16888=CARTESIAN_POINT('Origin',(155.884572681198,90.0000000000018,125.));
#16889=CARTESIAN_POINT('',(151.384572681198,90.0000000000018,124.475));
#16890=CARTESIAN_POINT('Origin',(155.884572681198,90.0000000000018,124.475));
#16891=CARTESIAN_POINT('',(150.859572681198,90.0000000000018,125.));
#16892=CARTESIAN_POINT('',(150.859572681198,90.0000000000018,125.));
#16893=CARTESIAN_POINT('Origin',(155.884572681198,90.0000000000018,125.));
#16894=CARTESIAN_POINT('Origin',(155.884572681198,90.0000000000018,125.));
#16895=CARTESIAN_POINT('',(151.384572681198,90.0000000000018,115.));
#16896=CARTESIAN_POINT('Origin',(155.884572681198,90.0000000000018,115.));
#16897=CARTESIAN_POINT('',(151.384572681198,90.0000000000018,125.));
#16898=CARTESIAN_POINT('Origin',(155.8845726812,-89.9999999999986,125.));
#16899=CARTESIAN_POINT('',(151.3845726812,-89.9999999999986,124.475));
#16900=CARTESIAN_POINT('Origin',(155.8845726812,-89.9999999999986,124.475));
#16901=CARTESIAN_POINT('',(150.8595726812,-89.9999999999986,125.));
#16902=CARTESIAN_POINT('',(150.8595726812,-89.9999999999986,125.));
#16903=CARTESIAN_POINT('Origin',(155.8845726812,-89.9999999999986,125.));
#16904=CARTESIAN_POINT('Origin',(155.8845726812,-89.9999999999986,125.));
#16905=CARTESIAN_POINT('',(151.3845726812,-89.9999999999986,115.));
#16906=CARTESIAN_POINT('Origin',(155.8845726812,-89.9999999999986,115.));
#16907=CARTESIAN_POINT('',(151.3845726812,-89.9999999999986,125.));
#16908=CARTESIAN_POINT('Origin',(0.,-180.,125.));
#16909=CARTESIAN_POINT('',(-4.49999999999999,-180.,124.475));
#16910=CARTESIAN_POINT('Origin',(0.,-180.,124.475));
#16911=CARTESIAN_POINT('',(-5.025,-180.,125.));
#16912=CARTESIAN_POINT('',(-5.025,-180.,125.));
#16913=CARTESIAN_POINT('Origin',(0.,-180.,125.));
#16914=CARTESIAN_POINT('Origin',(0.,-180.,125.));
#16915=CARTESIAN_POINT('',(-4.49999999999998,-180.,115.));
#16916=CARTESIAN_POINT('Origin',(0.,-180.,115.));
#16917=CARTESIAN_POINT('',(-4.49999999999998,-180.,125.));
#16918=CARTESIAN_POINT('Origin',(-155.884572681199,-90.0000000000007,125.));
#16919=CARTESIAN_POINT('',(-160.384572681199,-90.0000000000007,124.475));
#16920=CARTESIAN_POINT('Origin',(-155.884572681199,-90.0000000000007,124.475));
#16921=CARTESIAN_POINT('',(-160.909572681199,-90.0000000000007,125.));
#16922=CARTESIAN_POINT('',(-160.909572681199,-90.0000000000007,125.));
#16923=CARTESIAN_POINT('Origin',(-155.884572681199,-90.0000000000007,125.));
#16924=CARTESIAN_POINT('Origin',(-155.884572681199,-90.0000000000007,125.));
#16925=CARTESIAN_POINT('',(-160.384572681199,-90.0000000000007,115.));
#16926=CARTESIAN_POINT('Origin',(-155.884572681199,-90.0000000000007,115.));
#16927=CARTESIAN_POINT('',(-160.384572681199,-90.0000000000007,125.));
#16928=CARTESIAN_POINT('Origin',(-155.884572681199,89.9999999999996,125.));
#16929=CARTESIAN_POINT('',(-160.384572681199,89.9999999999996,124.475));
#16930=CARTESIAN_POINT('Origin',(-155.884572681199,89.9999999999996,124.475));
#16931=CARTESIAN_POINT('',(-160.909572681199,89.9999999999996,125.));
#16932=CARTESIAN_POINT('',(-160.909572681199,89.9999999999996,125.));
#16933=CARTESIAN_POINT('Origin',(-155.884572681199,89.9999999999996,125.));
#16934=CARTESIAN_POINT('Origin',(-155.884572681199,89.9999999999996,125.));
#16935=CARTESIAN_POINT('',(-160.384572681199,89.9999999999996,115.));
#16936=CARTESIAN_POINT('Origin',(-155.884572681199,89.9999999999996,115.));
#16937=CARTESIAN_POINT('',(-160.384572681199,89.9999999999996,125.));
#16938=CARTESIAN_POINT('Origin',(0.,180.,125.));
#16939=CARTESIAN_POINT('',(-4.49999999999999,180.,124.475));
#16940=CARTESIAN_POINT('Origin',(0.,180.,124.475));
#16941=CARTESIAN_POINT('',(-5.025,180.,125.));
#16942=CARTESIAN_POINT('',(-5.025,180.,125.));
#16943=CARTESIAN_POINT('Origin',(0.,180.,125.));
#16944=CARTESIAN_POINT('Origin',(0.,180.,125.));
#16945=CARTESIAN_POINT('',(-4.49999999999998,180.,115.));
#16946=CARTESIAN_POINT('Origin',(0.,180.,115.));
#16947=CARTESIAN_POINT('',(-4.49999999999998,180.,125.));
#16948=CARTESIAN_POINT('Origin',(0.,0.,125.));
#16949=CARTESIAN_POINT('',(195.,-2.38806125833734E-14,125.));
#16950=CARTESIAN_POINT('Origin',(0.,0.,-103.));
#16951=CARTESIAN_POINT('',(35.5,-4.3474961369731E-15,-103.));
#16952=CARTESIAN_POINT('Origin',(0.,0.,-103.));
#16953=CARTESIAN_POINT('',(37.5,-4.59242549680257E-15,-105.));
#16954=CARTESIAN_POINT('',(35.5,-4.3474961369731E-15,-103.));
#16955=CARTESIAN_POINT('Origin',(0.,0.,-105.));
#16956=CARTESIAN_POINT('Origin',(0.,0.,-96.9999999999999));
#16957=CARTESIAN_POINT('',(35.5,4.3474961369731E-15,-96.9999999999999));
#16958=CARTESIAN_POINT('',(-35.5,-4.3474961369731E-15,-96.9999999999999));
#16959=CARTESIAN_POINT('Origin',(0.,0.,-96.9999999999999));
#16960=CARTESIAN_POINT('Origin',(0.,0.,-96.9999999999999));
#16961=CARTESIAN_POINT('',(-37.5,-4.59242549680257E-15,-95.));
#16962=CARTESIAN_POINT('',(-35.5,-4.3474961369731E-15,-96.9999999999999));
#16963=CARTESIAN_POINT('Origin',(0.,0.,-95.));
#16964=CARTESIAN_POINT('Origin',(0.,0.,-93.));
#16965=CARTESIAN_POINT('',(35.5,-4.3474961369731E-15,-93.));
#16966=CARTESIAN_POINT('Origin',(-169.,-140.,-65.));
#16967=CARTESIAN_POINT('',(-169.,-125.,-60.5));
#16968=CARTESIAN_POINT('Origin',(-169.,-125.,-65.));
#16969=CARTESIAN_POINT('',(-169.,-140.,-60.5));
#16970=CARTESIAN_POINT('',(-169.,-140.,-60.5));
#16971=CARTESIAN_POINT('Origin',(-169.,-140.,-65.));
#16972=CARTESIAN_POINT('Origin',(-169.,-140.,65.));
#16973=CARTESIAN_POINT('',(-169.,-125.,69.5));
#16974=CARTESIAN_POINT('Origin',(-169.,-125.,65.));
#16975=CARTESIAN_POINT('',(-169.,-140.,69.5));
#16976=CARTESIAN_POINT('',(-169.,-140.,69.5));
#16977=CARTESIAN_POINT('Origin',(-169.,-140.,65.));
#16978=CARTESIAN_POINT('Origin',(169.,-140.,-65.));
#16979=CARTESIAN_POINT('',(169.,-125.,-60.5));
#16980=CARTESIAN_POINT('Origin',(169.,-125.,-65.));
#16981=CARTESIAN_POINT('',(169.,-140.,-60.5));
#16982=CARTESIAN_POINT('',(169.,-140.,-60.5));
#16983=CARTESIAN_POINT('Origin',(169.,-140.,-65.));
#16984=CARTESIAN_POINT('Origin',(169.,-140.,65.));
#16985=CARTESIAN_POINT('',(169.,-125.,69.5));
#16986=CARTESIAN_POINT('Origin',(169.,-125.,65.));
#16987=CARTESIAN_POINT('',(169.,-140.,69.5));
#16988=CARTESIAN_POINT('',(169.,-140.,69.5));
#16989=CARTESIAN_POINT('Origin',(169.,-140.,65.));
#16990=CARTESIAN_POINT('Origin',(-95.,158.745078663875,115.));
#16991=CARTESIAN_POINT('',(-82.1621621621622,137.293041006595,-44.9999999999999));
#16992=CARTESIAN_POINT('',(-91.875,183.548997205106,-45.));
#16993=CARTESIAN_POINT('Origin',(-95.,158.745078663875,-45.));
#16994=CARTESIAN_POINT('',(-91.875,183.548997205106,45.0000000000001));
#16995=CARTESIAN_POINT('',(-91.875,183.548997205106,-105.));
#16996=CARTESIAN_POINT('',(-82.1621621621622,137.293041006595,45.0000000000001));
#16997=CARTESIAN_POINT('Origin',(-95.,158.745078663875,45.0000000000001));
#16998=CARTESIAN_POINT('',(-82.1621621621621,137.293041006595,115.));
#16999=CARTESIAN_POINT('Origin',(0.,0.,115.));
#17000=CARTESIAN_POINT('',(-12.5969447708578,159.503344737469,-95.));
#17001=CARTESIAN_POINT('Origin',(0.,0.,-95.));
#17002=CARTESIAN_POINT('Ctrl Pts',(-82.1621621621622,137.293041006595,-45.));
#17003=CARTESIAN_POINT('Ctrl Pts',(-82.1621621620898,137.293041006638,-45.8956808810957));
#17004=CARTESIAN_POINT('Ctrl Pts',(-82.1332503382887,137.310362174487,-46.7855749735046));
#17005=CARTESIAN_POINT('Ctrl Pts',(-82.0763076034376,137.344386309753,-47.6698671589124));
#17006=CARTESIAN_POINT('Ctrl Pts',(-82.0604557369373,137.353858036944,-47.9160387154245));
#17007=CARTESIAN_POINT('Ctrl Pts',(-82.042431814488,137.36462402734,-48.161776221576));
#17008=CARTESIAN_POINT('Ctrl Pts',(-82.0222554199955,137.376670566071,-48.4070838498355));
#17009=CARTESIAN_POINT('Ctrl Pts',(-81.9465407866535,137.421876822489,-49.3276337100496));
#17010=CARTESIAN_POINT('Ctrl Pts',(-81.840502580685,137.485121623027,-50.2421320047361));
#17011=CARTESIAN_POINT('Ctrl Pts',(-81.7046585719633,137.56579962954,-51.1506976196694));
#17012=CARTESIAN_POINT('Ctrl Pts',(-81.6751455849419,137.583327446788,-51.3480893593125));
#17013=CARTESIAN_POINT('Ctrl Pts',(-81.6442279669171,137.601676775247,-51.5451821462862));
#17014=CARTESIAN_POINT('Ctrl Pts',(-81.6119109575879,137.620841408021,-51.7419836113765));
#17015=CARTESIAN_POINT('Ctrl Pts',(-81.497776835662,137.688525224661,-52.4370281986711));
#17016=CARTESIAN_POINT('Ctrl Pts',(-81.3661884614961,137.766377965718,-53.1284391494042));
#17017=CARTESIAN_POINT('Ctrl Pts',(-81.2171404377993,137.854188085092,-53.8164994257697));
#17018=CARTESIAN_POINT('Ctrl Pts',(-81.1308907209676,137.905001223993,-54.2146597134931));
#17019=CARTESIAN_POINT('Ctrl Pts',(-81.0387936079803,137.959149117421,-54.6116977958882));
#17020=CARTESIAN_POINT('Ctrl Pts',(-80.9408410263292,138.01659412532,-55.0076668915174));
#17021=CARTESIAN_POINT('Ctrl Pts',(-80.8078101077321,138.094611080472,-55.5454386545451));
#17022=CARTESIAN_POINT('Ctrl Pts',(-80.6639677088331,138.178711759688,-56.0812362030082));
#17023=CARTESIAN_POINT('Ctrl Pts',(-80.5092092471911,138.268822322297,-56.6151741291791));
#17024=CARTESIAN_POINT('Ctrl Pts',(-80.4598920531534,138.297538038736,-56.7853252151335));
#17025=CARTESIAN_POINT('Ctrl Pts',(-80.4094775869982,138.326857136585,-56.955221756991));
#17026=CARTESIAN_POINT('Ctrl Pts',(-80.3580264160791,138.356740035565,-57.1246996088993));
#17027=CARTESIAN_POINT('Ctrl Pts',(-80.2486201865606,138.420283298937,-57.48507882735));
#17028=CARTESIAN_POINT('Ctrl Pts',(-80.1344832799705,138.486400947608,-57.8436980583636));
#17029=CARTESIAN_POINT('Ctrl Pts',(-80.0161972390454,138.55471186287,-58.1989404973028));
#17030=CARTESIAN_POINT('Ctrl Pts',(-79.7044269738313,138.734761106227,-59.1352642472327));
#17031=CARTESIAN_POINT('Ctrl Pts',(-79.3625347898603,138.930810670846,-60.0529663482358));
#17032=CARTESIAN_POINT('Ctrl Pts',(-78.9916175899106,139.141382683262,-60.9537945777502));
#17033=CARTESIAN_POINT('Ctrl Pts',(-78.9517483894941,139.164016677497,-61.0506229298144));
#17034=CARTESIAN_POINT('Ctrl Pts',(-78.9115438397022,139.186818412233,-61.1472563431337));
#17035=CARTESIAN_POINT('Ctrl Pts',(-78.8710053024311,139.209786015874,-61.2436970022178));
#17036=CARTESIAN_POINT('Ctrl Pts',(-78.653076104096,139.333256466116,-61.762147763787));
#17037=CARTESIAN_POINT('Ctrl Pts',(-78.4254901802515,139.461523555169,-62.2750241275225));
#17038=CARTESIAN_POINT('Ctrl Pts',(-78.1883402386737,139.594353793634,-62.7825737116347));
#17039=CARTESIAN_POINT('Ctrl Pts',(-77.9757260681242,139.71344128228,-63.2376117062502));
#17040=CARTESIAN_POINT('Ctrl Pts',(-77.7554805786764,139.836164959048,-63.6882429907043));
#17041=CARTESIAN_POINT('Ctrl Pts',(-77.5277216033442,139.962324869928,-64.1345780407656));
#17042=CARTESIAN_POINT('Ctrl Pts',(-77.3016103965922,140.087572051301,-64.5776839892267));
#17043=CARTESIAN_POINT('Ctrl Pts',(-77.0680917138838,140.216207282072,-65.0165537711084));
#17044=CARTESIAN_POINT('Ctrl Pts',(-76.8272244703531,140.348059230023,-65.4512527482325));
#17045=CARTESIAN_POINT('Ctrl Pts',(-76.5598938718774,140.494397352381,-65.9337107861455));
#17046=CARTESIAN_POINT('Ctrl Pts',(-76.283495691648,140.6447064215,-66.4110683238974));
#17047=CARTESIAN_POINT('Ctrl Pts',(-75.9981293972275,140.798736954998,-66.8833902572378));
#17048=CARTESIAN_POINT('Ctrl Pts',(-75.7822524315751,140.915259630728,-67.2406974367265));
#17049=CARTESIAN_POINT('Ctrl Pts',(-75.5610017760309,141.034037807636,-67.5954458574455));
#17050=CARTESIAN_POINT('Ctrl Pts',(-75.3356990939032,141.154285467157,-67.9457481010467));
#17051=CARTESIAN_POINT('Ctrl Pts',(-75.3201844290252,141.162565892948,-67.9698704144792));
#17052=CARTESIAN_POINT('Ctrl Pts',(-75.3046505622078,141.170853279768,-67.9939716299542));
#17053=CARTESIAN_POINT('Ctrl Pts',(-75.2890979304666,141.179147367824,-68.0180511247126));
#17054=CARTESIAN_POINT('Ctrl Pts',(-75.248703999487,141.200689112399,-68.080591372915));
#17055=CARTESIAN_POINT('Ctrl Pts',(-75.2081802678764,141.222277777914,-68.1429904246721));
#17056=CARTESIAN_POINT('Ctrl Pts',(-75.1675344072028,141.243908793063,-68.205237202427));
#17057=CARTESIAN_POINT('Ctrl Pts',(-74.8854046764752,141.394053294326,-68.6373025186886));
#17058=CARTESIAN_POINT('Ctrl Pts',(-74.5969543424691,141.546476593965,-69.0627940644927));
#17059=CARTESIAN_POINT('Ctrl Pts',(-74.3023794330922,141.700940048339,-69.4819598157056));
#17060=CARTESIAN_POINT('Ctrl Pts',(-73.9413538470785,141.890247614456,-69.9956816438427));
#17061=CARTESIAN_POINT('Ctrl Pts',(-73.5711387365508,142.082613055927,-70.4999175422413));
#17062=CARTESIAN_POINT('Ctrl Pts',(-73.1920302731841,142.277638576512,-70.9950211945631));
#17063=CARTESIAN_POINT('Ctrl Pts',(-72.9571177373819,142.398485099378,-71.3018095300674));
#17064=CARTESIAN_POINT('Ctrl Pts',(-72.7187910465147,142.520352610966,-71.6050922936546));
#17065=CARTESIAN_POINT('Ctrl Pts',(-72.4771257062136,142.643143015591,-71.904961551415));
#17066=CARTESIAN_POINT('Ctrl Pts',(-72.2471941166274,142.759971489571,-72.1902710418823));
#17067=CARTESIAN_POINT('Ctrl Pts',(-72.0142391557779,142.877636119185,-72.472488769632));
#17068=CARTESIAN_POINT('Ctrl Pts',(-71.7783094935174,142.996063179386,-72.751667986971));
#17069=CARTESIAN_POINT('Ctrl Pts',(-71.3719031956286,143.200062552101,-73.2325748431889));
#17070=CARTESIAN_POINT('Ctrl Pts',(-70.9566250939629,143.406347242988,-73.7045023042245));
#17071=CARTESIAN_POINT('Ctrl Pts',(-70.5326862235245,143.614554186242,-74.1678187118353));
#17072=CARTESIAN_POINT('Ctrl Pts',(-70.0130610572177,143.869755053769,-74.7357092313069));
#17073=CARTESIAN_POINT('Ctrl Pts',(-69.4804552925272,144.127824642797,-75.2907111591283));
#17074=CARTESIAN_POINT('Ctrl Pts',(-68.9350883593252,144.388196564031,-75.8332462671249));
#17075=CARTESIAN_POINT('Ctrl Pts',(-68.5485065908993,144.572760445027,-76.2178207044695));
#17076=CARTESIAN_POINT('Ctrl Pts',(-68.1555132304399,144.758480717796,-76.596131950207));
#17077=CARTESIAN_POINT('Ctrl Pts',(-67.7561927121406,144.945149385449,-76.9683433312052));
#17078=CARTESIAN_POINT('Ctrl Pts',(-67.2837105909669,145.166018597041,-77.4087495080978));
#17079=CARTESIAN_POINT('Ctrl Pts',(-66.8023415189655,145.388228815956,-77.8406036136869));
#17080=CARTESIAN_POINT('Ctrl Pts',(-66.3123287087178,145.611383693817,-78.2640873513956));
#17081=CARTESIAN_POINT('Ctrl Pts',(-66.0648257909633,145.724098060108,-78.4779867811913));
#17082=CARTESIAN_POINT('Ctrl Pts',(-65.8148876609796,145.837153384037,-78.6899061289426));
#17083=CARTESIAN_POINT('Ctrl Pts',(-65.5628580637272,145.950365739295,-78.8996153026583));
#17084=CARTESIAN_POINT('Ctrl Pts',(-65.1942221791109,146.115957944278,-79.206350414755));
#17085=CARTESIAN_POINT('Ctrl Pts',(-64.820779748259,146.282034503608,-79.5086408854622));
#17086=CARTESIAN_POINT('Ctrl Pts',(-64.4438701328714,146.447897285852,-79.8055427686403));
#17087=CARTESIAN_POINT('Ctrl Pts',(-64.3122652712965,146.505811299202,-79.9092114723342));
#17088=CARTESIAN_POINT('Ctrl Pts',(-64.1802381240679,146.56369914227,-80.0122234022978));
#17089=CARTESIAN_POINT('Ctrl Pts',(-64.0478469452313,146.621530825729,-80.1145390866013));
#17090=CARTESIAN_POINT('Ctrl Pts',(-63.78695174754,146.735496186726,-80.3161663469507));
#17091=CARTESIAN_POINT('Ctrl Pts',(-63.5245936249025,146.849270772549,-80.5151564102869));
#17092=CARTESIAN_POINT('Ctrl Pts',(-63.2608931848606,146.962781832294,-80.7114996909868));
#17093=CARTESIAN_POINT('Ctrl Pts',(-62.7500940644695,147.182657648439,-81.0918250899897));
#17094=CARTESIAN_POINT('Ctrl Pts',(-62.2338700369337,147.401712680234,-81.4625003839186));
#17095=CARTESIAN_POINT('Ctrl Pts',(-61.7123790491669,147.619721826396,-81.8239969669797));
#17096=CARTESIAN_POINT('Ctrl Pts',(-60.9875045505543,147.922755386369,-82.3264786215886));
#17097=CARTESIAN_POINT('Ctrl Pts',(-60.2524717621619,148.22375568285,-82.8112825188533));
#17098=CARTESIAN_POINT('Ctrl Pts',(-59.5075864500793,148.522204166141,-83.2793071779857));
#17099=CARTESIAN_POINT('Ctrl Pts',(-59.1501577232241,148.665412871809,-83.5038859894309));
#17100=CARTESIAN_POINT('Ctrl Pts',(-58.7904606523049,148.808033919482,-83.724602128888));
#17101=CARTESIAN_POINT('Ctrl Pts',(-58.4285301239598,148.950009475213,-83.9415589199558));
#17102=CARTESIAN_POINT('Ctrl Pts',(-57.911059102069,149.152999359055,-84.2517534009057));
#17103=CARTESIAN_POINT('Ctrl Pts',(-57.3890213558604,149.354670232681,-84.5542415763276));
#17104=CARTESIAN_POINT('Ctrl Pts',(-56.8625067494514,149.554857247062,-84.8493362502414));
#17105=CARTESIAN_POINT('Ctrl Pts',(-55.9822840681341,149.889528210448,-85.3426730389139));
#17106=CARTESIAN_POINT('Ctrl Pts',(-55.0895386431195,150.220060731732,-85.8153114005049));
#17107=CARTESIAN_POINT('Ctrl Pts',(-54.1845193914356,150.545796080153,-86.2681831732401));
#17108=CARTESIAN_POINT('Ctrl Pts',(-53.3953903177273,150.829820130796,-86.6630634830924));
#17109=CARTESIAN_POINT('Ctrl Pts',(-52.5969297863791,151.110196736556,-87.0429162429449));
#17110=CARTESIAN_POINT('Ctrl Pts',(-51.7893118661202,151.386482806261,-87.4083895500494));
#17111=CARTESIAN_POINT('Ctrl Pts',(-50.7892348830617,151.72860911639,-87.8609568262193));
#17112=CARTESIAN_POINT('Ctrl Pts',(-49.7751097566078,152.064469149807,-88.2914533321514));
#17113=CARTESIAN_POINT('Ctrl Pts',(-48.7471190027564,152.393300182218,-88.7006682117858));
#17114=CARTESIAN_POINT('Ctrl Pts',(-48.4756335577533,152.480142246537,-88.8087391095864));
#17115=CARTESIAN_POINT('Ctrl Pts',(-48.2031811311436,152.566494018159,-88.9153259807367));
#17116=CARTESIAN_POINT('Ctrl Pts',(-47.9297652567514,152.652341336682,-89.0204439275952));
#17117=CARTESIAN_POINT('Ctrl Pts',(-47.4575992189624,152.800592378551,-89.2019737110398));
#17118=CARTESIAN_POINT('Ctrl Pts',(-46.9826690249351,152.947305215845,-89.3790749428026));
#17119=CARTESIAN_POINT('Ctrl Pts',(-46.5048664571461,153.092447219982,-89.5518784063299));
#17120=CARTESIAN_POINT('Ctrl Pts',(-46.0524027842201,153.22989203237,-89.715517731593));
#17121=CARTESIAN_POINT('Ctrl Pts',(-45.5969278339165,153.366049750584,-89.8754273982279));
#17122=CARTESIAN_POINT('Ctrl Pts',(-45.1392201295791,153.50064581587,-90.0314149120475));
#17123=CARTESIAN_POINT('Ctrl Pts',(-44.6903085940134,153.632655230997,-90.1844046775557));
#17124=CARTESIAN_POINT('Ctrl Pts',(-44.2394010756355,153.763116931994,-90.3335681685666));
#17125=CARTESIAN_POINT('Ctrl Pts',(-43.7875118830157,153.891695042633,-90.4786409992244));
#17126=CARTESIAN_POINT('Ctrl Pts',(-43.2921110680564,154.032653715327,-90.6376826397638));
#17127=CARTESIAN_POINT('Ctrl Pts',(-42.7955108465802,154.171367045258,-90.7918416708324));
#17128=CARTESIAN_POINT('Ctrl Pts',(-42.2979532665998,154.30775466438,-90.9411999794216));
#17129=CARTESIAN_POINT('Ctrl Pts',(-41.8806358039081,154.422147324535,-91.0664715718569));
#17130=CARTESIAN_POINT('Ctrl Pts',(-41.4625232501022,154.534937799496,-91.1884006026406));
#17131=CARTESIAN_POINT('Ctrl Pts',(-41.0436262570233,154.646114544382,-91.3070752601544));
#17132=CARTESIAN_POINT('Ctrl Pts',(-39.5524929062776,155.041866614378,-91.7295173942139));
#17133=CARTESIAN_POINT('Ctrl Pts',(-38.0514284305851,155.417169263234,-92.1107963665915));
#17134=CARTESIAN_POINT('Ctrl Pts',(-36.5408147180781,155.77152793962,-92.454022437313));
#17135=CARTESIAN_POINT('Ctrl Pts',(-36.1938322098199,155.852922846431,-92.5328602248509));
#17136=CARTESIAN_POINT('Ctrl Pts',(-35.8463458936313,155.93321278559,-92.6096870883139));
#17137=CARTESIAN_POINT('Ctrl Pts',(-35.4983599483625,156.01239194686,-92.684541040783));
#17138=CARTESIAN_POINT('Ctrl Pts',(-33.7317739216286,156.41435300825,-93.0645447400004));
#17139=CARTESIAN_POINT('Ctrl Pts',(-31.9523436552056,156.787699874605,-93.3939621738583));
#17140=CARTESIAN_POINT('Ctrl Pts',(-30.1603845094755,157.131655945597,-93.6757820461854));
#17141=CARTESIAN_POINT('Ctrl Pts',(-28.3684253637454,157.47561201659,-93.9576019185125));
#17142=CARTESIAN_POINT('Ctrl Pts',(-26.5639372568348,157.79017734767,-94.1918245741718));
#17143=CARTESIAN_POINT('Ctrl Pts',(-24.7472365628837,158.074585235959,-94.381496509228));
#17144=CARTESIAN_POINT('Ctrl Pts',(-24.5611024521864,158.103724878795,-94.4009297692435));
#17145=CARTESIAN_POINT('Ctrl Pts',(-24.3748401558089,158.132547950449,-94.4198947199084));
#17146=CARTESIAN_POINT('Ctrl Pts',(-24.1884499321931,158.161053644401,-94.4383946498845));
#17147=CARTESIAN_POINT('Ctrl Pts',(-21.8827037855024,158.51368423153,-94.6672486178073));
#17148=CARTESIAN_POINT('Ctrl Pts',(-19.5573481612408,158.817774755384,-94.8247861359747));
#17149=CARTESIAN_POINT('Ctrl Pts',(-17.2124345002704,159.071497582772,-94.9135091757608));
#17150=CARTESIAN_POINT('Ctrl Pts',(-15.6822612741615,159.237064393945,-94.9714053884356));
#17151=CARTESIAN_POINT('Ctrl Pts',(-14.1437598313738,159.381183387686,-95.));
#17152=CARTESIAN_POINT('Ctrl Pts',(-12.5969447708578,159.503344737469,-95.));
#17153=CARTESIAN_POINT('',(-12.5969447708577,159.503344737469,95.));
#17154=CARTESIAN_POINT('Ctrl Pts',(-12.5969447708577,159.503344737469,95.));
#17155=CARTESIAN_POINT('Ctrl Pts',(-14.9636417884215,159.316432345954,95.));
#17156=CARTESIAN_POINT('Ctrl Pts',(-17.3102321971143,159.0781682305,94.9330539868556));
#17157=CARTESIAN_POINT('Ctrl Pts',(-19.6366874222696,158.790458660472,94.7967566416616));
#17158=CARTESIAN_POINT('Ctrl Pts',(-21.1618309392931,158.601846225223,94.7074048199878));
#17159=CARTESIAN_POINT('Ctrl Pts',(-22.6783210761119,158.391983596727,94.5882491690846));
#17160=CARTESIAN_POINT('Ctrl Pts',(-24.1861500481769,158.161405361344,94.4386239423497));
#17161=CARTESIAN_POINT('Ctrl Pts',(-24.3718651728656,158.133005677741,94.4201950169514));
#17162=CARTESIAN_POINT('Ctrl Pts',(-24.5574491231664,158.104291546955,94.4013048160663));
#17163=CARTESIAN_POINT('Ctrl Pts',(-24.742901648231,158.075263811836,94.3819501633167));
#17164=CARTESIAN_POINT('Ctrl Pts',(-26.5589242771186,157.791013037557,94.1924219411736));
#17165=CARTESIAN_POINT('Ctrl Pts',(-28.3623429571352,157.476689937671,93.9584167982046));
#17166=CARTESIAN_POINT('Ctrl Pts',(-30.152843339076,157.13310297412,93.6769646228227));
#17167=CARTESIAN_POINT('Ctrl Pts',(-31.9433437210169,156.78951601057,93.3955124474409));
#17168=CARTESIAN_POINT('Ctrl Pts',(-33.7209258842786,156.416665133799,93.0666128972902));
#17169=CARTESIAN_POINT('Ctrl Pts',(-35.4852769954844,156.015368206333,92.6873548341285));
#17170=CARTESIAN_POINT('Ctrl Pts',(-35.8310461983781,155.936723928643,92.6130296290389));
#17171=CARTESIAN_POINT('Ctrl Pts',(-36.1763059771042,155.856986669202,92.5367605125138));
#17172=CARTESIAN_POINT('Ctrl Pts',(-36.5210521960025,155.776162483908,92.4585109007515));
#17173=CARTESIAN_POINT('Ctrl Pts',(-38.0313492281534,155.422080204005,92.1157075575005));
#17174=CARTESIAN_POINT('Ctrl Pts',(-39.531789681437,155.04713651561,91.7349542431376));
#17175=CARTESIAN_POINT('Ctrl Pts',(-41.0219877582951,154.651855858113,91.313202808891));
#17176=CARTESIAN_POINT('Ctrl Pts',(-41.437589578251,154.541615908673,91.1955804160267));
#17177=CARTESIAN_POINT('Ctrl Pts',(-41.8523940604112,154.429794280005,91.074763575325));
#17178=CARTESIAN_POINT('Ctrl Pts',(-42.2663906571552,154.316402951417,90.9506677174281));
#17179=CARTESIAN_POINT('Ctrl Pts',(-42.7657626262669,154.179627790745,90.8009805137071));
#17180=CARTESIAN_POINT('Ctrl Pts',(-43.263888543544,154.040588238986,90.6465480667306));
#17181=CARTESIAN_POINT('Ctrl Pts',(-43.7607921601594,153.899295220983,90.4872139652418));
#17182=CARTESIAN_POINT('Ctrl Pts',(-44.2084160951198,153.772014729181,90.3436815877405));
#17183=CARTESIAN_POINT('Ctrl Pts',(-44.6554133136073,153.642793503939,90.1960376830759));
#17184=CARTESIAN_POINT('Ctrl Pts',(-45.1011708062992,153.51183157811,90.0443759449032));
#17185=CARTESIAN_POINT('Ctrl Pts',(-45.5617485068334,153.376515529262,89.8876718720119));
#17186=CARTESIAN_POINT('Ctrl Pts',(-46.0211788417636,153.23928812832,89.7266157921222));
#17187=CARTESIAN_POINT('Ctrl Pts',(-46.4784104196994,153.100481269192,89.5614409688638));
#17188=CARTESIAN_POINT('Ctrl Pts',(-46.9549345962594,152.955817542015,89.3892966979082));
#17189=CARTESIAN_POINT('Ctrl Pts',(-47.4286966966318,152.809560712439,89.2128429647634));
#17190=CARTESIAN_POINT('Ctrl Pts',(-47.8993019180429,152.661902914232,89.0321483088218));
#17191=CARTESIAN_POINT('Ctrl Pts',(-48.9370157977482,152.33630825511,88.6337053168444));
#17192=CARTESIAN_POINT('Ctrl Pts',(-49.9607219667338,152.003487175208,88.2141700656783));
#17193=CARTESIAN_POINT('Ctrl Pts',(-50.9702419222352,151.664215661609,87.7727550423618));
#17194=CARTESIAN_POINT('Ctrl Pts',(-51.2399157194243,151.573585816353,87.6548395273436));
#17195=CARTESIAN_POINT('Ctrl Pts',(-51.5085772869238,151.48249561964,87.5353629667694));
#17196=CARTESIAN_POINT('Ctrl Pts',(-51.7762234015762,151.39095973765,87.4143109434925));
#17197=CARTESIAN_POINT('Ctrl Pts',(-52.7040666243346,151.07363419809,86.9946624104116));
#17198=CARTESIAN_POINT('Ctrl Pts',(-53.6197103208516,150.750948057866,86.5560940609331));
#17199=CARTESIAN_POINT('Ctrl Pts',(-54.522898061456,150.423576793448,86.0976450826551));
#17200=CARTESIAN_POINT('Ctrl Pts',(-55.3114117171572,150.137770530949,85.6974035120902));
#17201=CARTESIAN_POINT('Ctrl Pts',(-56.0904317952114,149.848393194912,85.2820098082707));
#17202=CARTESIAN_POINT('Ctrl Pts',(-56.8597968038474,149.55588757199,84.8508551158301));
#17203=CARTESIAN_POINT('Ctrl Pts',(-57.3859544162636,149.355847203052,84.5559946516678));
#17204=CARTESIAN_POINT('Ctrl Pts',(-57.9075999728538,149.154340665475,84.2537745826551));
#17205=CARTESIAN_POINT('Ctrl Pts',(-58.4246450085192,148.951533444028,83.9438875982944));
#17206=CARTESIAN_POINT('Ctrl Pts',(-59.1798215757925,148.65532083053,83.4912783032626));
#17207=CARTESIAN_POINT('Ctrl Pts',(-59.9251856576475,148.3563328907,83.0223558694528));
#17208=CARTESIAN_POINT('Ctrl Pts',(-60.6604276238275,148.055096320812,82.536209125394));
#17209=CARTESIAN_POINT('Ctrl Pts',(-61.0150211334615,147.909815532364,82.3017496030839));
#17210=CARTESIAN_POINT('Ctrl Pts',(-61.3672604880628,147.764011622712,82.0632845126909));
#17211=CARTESIAN_POINT('Ctrl Pts',(-61.7171120951143,147.617743088862,81.8207158106705));
#17212=CARTESIAN_POINT('Ctrl Pts',(-62.2383495586455,147.399820295193,81.4593171707193));
#17213=CARTESIAN_POINT('Ctrl Pts',(-62.7542769913379,147.180872854704,81.088778898013));
#17214=CARTESIAN_POINT('Ctrl Pts',(-63.2647378765564,146.961126802859,80.708636791763));
#17215=CARTESIAN_POINT('Ctrl Pts',(-63.5296293498669,146.847094842502,80.5113711333987));
#17216=CARTESIAN_POINT('Ctrl Pts',(-63.7931631002249,146.732798349721,80.3114362119227));
#17217=CARTESIAN_POINT('Ctrl Pts',(-64.0552014820334,146.618317965717,80.108854249111));
#17218=CARTESIAN_POINT('Ctrl Pts',(-64.4278584607107,146.455510083427,79.8207530111361));
#17219=CARTESIAN_POINT('Ctrl Pts',(-64.797203825589,146.292446583308,79.5274726487448));
#17220=CARTESIAN_POINT('Ctrl Pts',(-65.1621722401331,146.129699532309,79.2297442284713));
#17221=CARTESIAN_POINT('Ctrl Pts',(-65.297942280548,146.069156831048,79.1189877957436));
#17222=CARTESIAN_POINT('Ctrl Pts',(-65.4331070021292,146.008657850992,79.0076161106079));
#17223=CARTESIAN_POINT('Ctrl Pts',(-65.5676131150429,145.948231707859,78.8956678072283));
#17224=CARTESIAN_POINT('Ctrl Pts',(-65.8202507336994,145.834735625229,78.6853996479172));
#17225=CARTESIAN_POINT('Ctrl Pts',(-66.0707786683664,145.7214004756,78.4729134763841));
#17226=CARTESIAN_POINT('Ctrl Pts',(-66.3189251278449,145.608379463163,78.2583853065394));
#17227=CARTESIAN_POINT('Ctrl Pts',(-66.8077600897421,145.385734246204,77.8357765377006));
#17228=CARTESIAN_POINT('Ctrl Pts',(-67.2881427185282,145.163960479824,77.4047019300111));
#17229=CARTESIAN_POINT('Ctrl Pts',(-67.7597446135163,144.943488495273,76.965032086193));
#17230=CARTESIAN_POINT('Ctrl Pts',(-68.318258240347,144.682385626488,76.4443352830447));
#17231=CARTESIAN_POINT('Ctrl Pts',(-68.8645488295706,144.423066620625,75.9115540124255));
#17232=CARTESIAN_POINT('Ctrl Pts',(-69.3983709814738,144.166099904753,75.3662201410075));
#17233=CARTESIAN_POINT('Ctrl Pts',(-69.7852507803295,143.979867034883,74.9709973917619));
#17234=CARTESIAN_POINT('Ctrl Pts',(-70.1655820585078,143.794869292409,74.5691823587563));
#17235=CARTESIAN_POINT('Ctrl Pts',(-70.5392781657233,143.611316531388,74.1606111912411));
#17236=CARTESIAN_POINT('Ctrl Pts',(-70.9627708629114,143.403304587084,73.6975961841716));
#17237=CARTESIAN_POINT('Ctrl Pts',(-71.3777208982096,143.197162011134,73.2258699409069));
#17238=CARTESIAN_POINT('Ctrl Pts',(-71.7839076638945,142.993252942107,72.7450454092227));
#17239=CARTESIAN_POINT('Ctrl Pts',(-72.0208475537841,142.874307185022,72.4645672616853));
#17240=CARTESIAN_POINT('Ctrl Pts',(-72.2548059546961,142.756121130267,72.1809957430739));
#17241=CARTESIAN_POINT('Ctrl Pts',(-72.4857415364824,142.638764976099,71.8942661065626));
#17242=CARTESIAN_POINT('Ctrl Pts',(-72.8684374953895,142.444287686781,71.4191107738804));
#17243=CARTESIAN_POINT('Ctrl Pts',(-73.2428344044161,142.252088162916,70.9352862747557));
#17244=CARTESIAN_POINT('Ctrl Pts',(-73.6086679634405,142.062534534116,70.442372262658));
#17245=CARTESIAN_POINT('Ctrl Pts',(-73.8475013996346,141.938784967154,70.120574701025));
#17246=CARTESIAN_POINT('Ctrl Pts',(-74.0826769561078,141.816167236602,69.7949086505828));
#17247=CARTESIAN_POINT('Ctrl Pts',(-74.3141448724259,141.694770093608,69.4652303025532));
#17248=CARTESIAN_POINT('Ctrl Pts',(-74.5942217967198,141.547879159568,69.0663184395563));
#17249=CARTESIAN_POINT('Ctrl Pts',(-74.8691354183963,141.402625845848,68.6609941558653));
#17250=CARTESIAN_POINT('Ctrl Pts',(-75.1377859549508,141.259726775824,68.2506414100496));
#17251=CARTESIAN_POINT('Ctrl Pts',(-75.192420693496,141.230665775503,68.167189073544));
#17252=CARTESIAN_POINT('Ctrl Pts',(-75.2467964971052,141.201702079564,68.0835286394876));
#17253=CARTESIAN_POINT('Ctrl Pts',(-75.3009042600589,141.172841619946,67.9996715524561));
#17254=CARTESIAN_POINT('Ctrl Pts',(-75.5427668568644,141.043834887322,67.6248289841662));
#17255=CARTESIAN_POINT('Ctrl Pts',(-75.779235163084,140.916911689629,67.2461175539412));
#17256=CARTESIAN_POINT('Ctrl Pts',(-76.0095109018959,140.792593031219,66.8645514389451));
#17257=CARTESIAN_POINT('Ctrl Pts',(-76.4678093900085,140.545172032866,66.1051524049005));
#17258=CARTESIAN_POINT('Ctrl Pts',(-76.9030196715659,140.307330530175,65.3326162202851));
#17259=CARTESIAN_POINT('Ctrl Pts',(-77.314881639329,140.08000967159,64.5462581634978));
#17260=CARTESIAN_POINT('Ctrl Pts',(-77.3886533101512,140.039292536086,64.4054077032605));
#17261=CARTESIAN_POINT('Ctrl Pts',(-77.4616759218475,139.998912815778,64.2641138523276));
#17262=CARTESIAN_POINT('Ctrl Pts',(-77.5339480123353,139.958875765781,64.1223727486894));
#17263=CARTESIAN_POINT('Ctrl Pts',(-77.7608228970841,139.833192378979,63.6774223351203));
#17264=CARTESIAN_POINT('Ctrl Pts',(-77.9803042689531,139.710884654149,63.2280664572187));
#17265=CARTESIAN_POINT('Ctrl Pts',(-78.1922823959708,139.59214554871,62.774134193961));
#17266=CARTESIAN_POINT('Ctrl Pts',(-78.4291964078238,139.459438659422,62.2668039561155));
#17267=CARTESIAN_POINT('Ctrl Pts',(-78.656697695979,139.331212005233,61.7538460015109));
#17268=CARTESIAN_POINT('Ctrl Pts',(-78.8746118757149,139.207742605995,61.2351126948805));
#17269=CARTESIAN_POINT('Ctrl Pts',(-79.0457403477842,139.110781822329,60.8277503181747));
#17270=CARTESIAN_POINT('Ctrl Pts',(-79.2109597627441,139.016752899008,60.4168290717586));
#17271=CARTESIAN_POINT('Ctrl Pts',(-79.3701338567528,138.925814804349,60.0022364653027));
#17272=CARTESIAN_POINT('Ctrl Pts',(-79.5991272637939,138.794988087506,59.4057890717889));
#17273=CARTESIAN_POINT('Ctrl Pts',(-79.8155327390985,138.670602562738,58.8020121168909));
#17274=CARTESIAN_POINT('Ctrl Pts',(-80.0191366199309,138.553014310775,58.190105889466));
#17275=CARTESIAN_POINT('Ctrl Pts',(-80.1372766997562,138.484784346707,57.8350505228489));
#17276=CARTESIAN_POINT('Ctrl Pts',(-80.2512731188794,138.418744840624,57.4765876280007));
#17277=CARTESIAN_POINT('Ctrl Pts',(-80.3604379578907,138.35533929411,57.1167492175768));
#17278=CARTESIAN_POINT('Ctrl Pts',(-80.4119882901731,138.32539762955,56.9468246356937));
#17279=CARTESIAN_POINT('Ctrl Pts',(-80.4624757632866,138.296034849532,56.7765504471469));
#17280=CARTESIAN_POINT('Ctrl Pts',(-80.511824808259,138.267299337361,56.6061448214883));
#17281=CARTESIAN_POINT('Ctrl Pts',(-80.6661773762022,138.177421202995,56.0731548532513));
#17282=CARTESIAN_POINT('Ctrl Pts',(-80.80971869551,138.093493918004,55.5380894985181));
#17283=CARTESIAN_POINT('Ctrl Pts',(-80.9425086535139,138.015616119626,55.0009089778416));
#17284=CARTESIAN_POINT('Ctrl Pts',(-81.1848985336488,137.873460865587,54.0203595148038));
#17285=CARTESIAN_POINT('Ctrl Pts',(-81.3915079530963,137.751452856674,53.0327717650492));
#17286=CARTESIAN_POINT('Ctrl Pts',(-81.5622416952236,137.650284652651,52.0378044775898));
#17287=CARTESIAN_POINT('Ctrl Pts',(-81.5793285406492,137.640159849888,51.938229244056));
#17288=CARTESIAN_POINT('Ctrl Pts',(-81.5960560210763,137.630243783611,51.8385800942014));
#17289=CARTESIAN_POINT('Ctrl Pts',(-81.6124240130328,137.620537154591,51.7388566829908));
#17290=CARTESIAN_POINT('Ctrl Pts',(-81.6446771940527,137.601410210753,51.5423513790862));
#17291=CARTESIAN_POINT('Ctrl Pts',(-81.675534801156,137.583096367716,51.3455577967773));
#17292=CARTESIAN_POINT('Ctrl Pts',(-81.7049911434168,137.565602089959,51.1484722131202));
#17293=CARTESIAN_POINT('Ctrl Pts',(-81.840697101167,137.485005602549,50.240494988651));
#17294=CARTESIAN_POINT('Ctrl Pts',(-81.9466550214586,137.421808667808,49.3264666205647));
#17295=CARTESIAN_POINT('Ctrl Pts',(-82.0223229969576,137.376630218478,48.4062608221921));
#17296=CARTESIAN_POINT('Ctrl Pts',(-82.0939119350414,137.333887206121,47.5356606047341));
#17297=CARTESIAN_POINT('Ctrl Pts',(-82.1383964061816,137.307269356527,46.6595281125084));
#17298=CARTESIAN_POINT('Ctrl Pts',(-82.1548918638585,137.297394431107,45.777672594722));
#17299=CARTESIAN_POINT('Ctrl Pts',(-82.1597315135144,137.294497198405,45.5189424741761));
#17300=CARTESIAN_POINT('Ctrl Pts',(-82.1621621621139,137.293041006624,45.2597198077607));
#17301=CARTESIAN_POINT('Ctrl Pts',(-82.1621621621622,137.293041006595,45.0000000000001));
#17302=CARTESIAN_POINT('',(56.5922444183315,149.657334840949,95.));
#17303=CARTESIAN_POINT('Origin',(0.,0.,95.));
#17304=CARTESIAN_POINT('',(160.,3.36777869765522E-14,45.));
#17305=CARTESIAN_POINT('Ctrl Pts',(160.,3.36777869765522E-14,45.));
#17306=CARTESIAN_POINT('Ctrl Pts',(160.,0.244053147828224,45.0908288013671));
#17307=CARTESIAN_POINT('Ctrl Pts',(159.999433557959,0.492071829028524,45.1831334511064));
#17308=CARTESIAN_POINT('Ctrl Pts',(159.997155062312,0.985517893876185,45.3667780815545));
#17309=CARTESIAN_POINT('Ctrl Pts',(159.992026352869,1.72544209140982,45.6421534820189));
#17310=CARTESIAN_POINT('Ctrl Pts',(159.968105193101,3.45022173859571,46.2840540034421));
#17311=CARTESIAN_POINT('Ctrl Pts',(159.927183294251,4.92568645342637,46.8331493084511));
#17312=CARTESIAN_POINT('Ctrl Pts',(159.818287593492,7.87275838356731,47.9298532164966));
#17313=CARTESIAN_POINT('Ctrl Pts',(159.709630855535,9.83233101229018,48.6590074878283));
#17314=CARTESIAN_POINT('Ctrl Pts',(159.2765030292,15.6958359884224,50.8403997271284));
#17315=CARTESIAN_POINT('Ctrl Pts',(158.84502097174,19.5845746730536,52.2865796610741));
#17316=CARTESIAN_POINT('Ctrl Pts',(157.125137305964,31.190964030139,56.5994780417861));
#17317=CARTESIAN_POINT('Ctrl Pts',(155.413800322954,38.8490721013328,59.4408884221265));
#17318=CARTESIAN_POINT('Ctrl Pts',(152.828962450137,47.3739160272581,62.5917257526285));
#17319=CARTESIAN_POINT('Ctrl Pts',(152.532544816976,48.319857616323,62.9411763755992));
#17320=CARTESIAN_POINT('Ctrl Pts',(151.921104853419,50.2092000386463,63.638752880553));
#17321=CARTESIAN_POINT('Ctrl Pts',(151.60584962841,51.1532380133295,63.9871134500385));
#17322=CARTESIAN_POINT('Ctrl Pts',(150.63528262613,53.9718559190622,65.0265817145455));
#17323=CARTESIAN_POINT('Ctrl Pts',(149.954384630373,55.8355619005357,65.7130462914177));
#17324=CARTESIAN_POINT('Ctrl Pts',(147.810941106456,61.3810675999849,67.7526737154489));
#17325=CARTESIAN_POINT('Ctrl Pts',(146.24779276441,65.017314935261,69.0861171414286));
#17326=CARTESIAN_POINT('Ctrl Pts',(141.156919864418,75.7456037919146,73.004146909579));
#17327=CARTESIAN_POINT('Ctrl Pts',(137.230403745259,82.6581846336838,75.5075044348197));
#17328=CARTESIAN_POINT('Ctrl Pts',(131.623294985597,90.9908960669881,78.4763325219442));
#17329=CARTESIAN_POINT('Ctrl Pts',(130.466716096879,92.6419588132132,79.0619951565626));
#17330=CARTESIAN_POINT('Ctrl Pts',(128.677812363236,95.0949248954701,79.9275841406832));
#17331=CARTESIAN_POINT('Ctrl Pts',(128.071892999492,95.9094334951753,80.2142390390038));
#17332=CARTESIAN_POINT('Ctrl Pts',(126.845393169409,97.5257680899608,80.7814450557067));
#17333=CARTESIAN_POINT('Ctrl Pts',(126.224849980105,98.3275862731005,81.0619954633975));
#17334=CARTESIAN_POINT('Ctrl Pts',(123.085753077898,102.305078006677,82.4493004112037));
#17335=CARTESIAN_POINT('Ctrl Pts',(120.458236945284,105.386091967576,83.509847591627));
#17336=CARTESIAN_POINT('Ctrl Pts',(114.970035141697,111.347681824462,85.5255777952907));
#17337=CARTESIAN_POINT('Ctrl Pts',(112.109364020888,114.228261087591,86.4807952902017));
#17338=CARTESIAN_POINT('Ctrl Pts',(106.149377389369,119.786955934744,88.2752107002331));
#17339=CARTESIAN_POINT('Ctrl Pts',(103.05009718665,122.465087346466,89.1144688969865));
#17340=CARTESIAN_POINT('Ctrl Pts',(98.2139591883386,126.326059298113,90.2743768979733));
#17341=CARTESIAN_POINT('Ctrl Pts',(96.5704928774742,127.587107215203,90.6445055035526));
#17342=CARTESIAN_POINT('Ctrl Pts',(93.2197383402911,130.055412828185,91.3488393325667));
#17343=CARTESIAN_POINT('Ctrl Pts',(91.523272065474,131.254702876371,91.6807677118488));
#17344=CARTESIAN_POINT('Ctrl Pts',(86.3708892591745,134.749007104026,92.6132249860203));
#17345=CARTESIAN_POINT('Ctrl Pts',(82.8521059313916,136.940617783261,93.1507013044242));
#17346=CARTESIAN_POINT('Ctrl Pts',(75.6455579527511,141.049472945292,94.037579926942));
#17347=CARTESIAN_POINT('Ctrl Pts',(71.9578114879837,142.966725642616,94.3871133269088));
#17348=CARTESIAN_POINT('Ctrl Pts',(64.4081316590566,146.523048873891,94.8681992426883));
#17349=CARTESIAN_POINT('Ctrl Pts',(60.5462404390231,148.162149125729,95.));
#17350=CARTESIAN_POINT('Ctrl Pts',(56.5922444183315,149.657334840949,95.));
#17351=CARTESIAN_POINT('',(160.,-1.95943487863576E-14,125.));
#17352=CARTESIAN_POINT('',(160.,-1.95943487863576E-14,115.));
#17353=CARTESIAN_POINT('Origin',(0.,0.,125.));
#17354=CARTESIAN_POINT('',(160.,3.36777869765522E-14,-105.));
#17355=CARTESIAN_POINT('Origin',(-95.,158.745078663875,115.));
#17356=CARTESIAN_POINT('',(-80.,158.745078663875,-45.));
#17357=CARTESIAN_POINT('',(-93.125,173.627429788614,-45.));
#17358=CARTESIAN_POINT('Origin',(-95.,158.745078663875,-45.));
#17359=CARTESIAN_POINT('',(-87.2972972972973,145.873856069507,-45.));
#17360=CARTESIAN_POINT('Origin',(-95.,158.745078663875,-45.));
#17361=CARTESIAN_POINT('',(-87.2972972972973,145.873856069507,45.0000000000001));
#17362=CARTESIAN_POINT('',(-87.2972972972972,145.873856069507,115.));
#17363=CARTESIAN_POINT('',(-80.,158.745078663875,45.0000000000001));
#17364=CARTESIAN_POINT('Origin',(-95.,158.745078663875,45.0000000000001));
#17365=CARTESIAN_POINT('',(-93.125,173.627429788614,45.0000000000001));
#17366=CARTESIAN_POINT('Origin',(-95.,158.745078663875,45.0000000000001));
#17367=CARTESIAN_POINT('',(-93.125,173.627429788614,-105.));
#17368=CARTESIAN_POINT('Origin',(0.,0.,115.));
#17369=CARTESIAN_POINT('',(170.,0.,-45.));
#17370=CARTESIAN_POINT('',(170.,-2.0818995585505E-14,115.));
#17371=CARTESIAN_POINT('',(170.,0.,45.));
#17372=CARTESIAN_POINT('',(170.,0.,-80.));
#17373=CARTESIAN_POINT('',(170.,-2.0818995585505E-14,115.));
#17374=CARTESIAN_POINT('',(170.,-2.0818995585505E-14,115.));
#17375=CARTESIAN_POINT('Origin',(0.,0.,115.));
#17376=CARTESIAN_POINT('',(60.1292596944772,159.010918268508,95.));
#17377=CARTESIAN_POINT('Ctrl Pts',(170.,0.,45.));
#17378=CARTESIAN_POINT('Ctrl Pts',(170.,0.26003052026448,45.091082419179));
#17379=CARTESIAN_POINT('Ctrl Pts',(169.999394183212,0.524501631954243,45.1837202730264));
#17380=CARTESIAN_POINT('Ctrl Pts',(169.996958612046,1.05032722296935,45.3679040271418));
#17381=CARTESIAN_POINT('Ctrl Pts',(169.991476684799,1.83880024712644,45.6440863033289));
#17382=CARTESIAN_POINT('Ctrl Pts',(169.965910091794,3.67671754845105,46.2878568548837));
#17383=CARTESIAN_POINT('Ctrl Pts',(169.922176515592,5.24891333774521,46.8385332643445));
#17384=CARTESIAN_POINT('Ctrl Pts',(169.80580451179,8.38912428069815,47.9383702016001));
#17385=CARTESIAN_POINT('Ctrl Pts',(169.689693680506,10.47702552627,48.6695742664345));
#17386=CARTESIAN_POINT('Ctrl Pts',(169.22689115823,16.7242377993534,50.85699761865));
#17387=CARTESIAN_POINT('Ctrl Pts',(168.765886558002,20.8670784878288,52.3070408841403));
#17388=CARTESIAN_POINT('Ctrl Pts',(166.928601437382,33.2307048294446,56.6310354999103));
#17389=CARTESIAN_POINT('Ctrl Pts',(165.100719651717,41.3869108937082,59.4791921961275));
#17390=CARTESIAN_POINT('Ctrl Pts',(162.340601127124,50.4642501038184,62.6367460390978));
#17391=CARTESIAN_POINT('Ctrl Pts',(162.024090898783,51.4714701492619,62.9869306646656));
#17392=CARTESIAN_POINT('Ctrl Pts',(161.371221757297,53.4831474341294,63.6859498503516));
#17393=CARTESIAN_POINT('Ctrl Pts',(161.034658418127,54.4881463629123,64.0349720718961));
#17394=CARTESIAN_POINT('Ctrl Pts',(159.99868842936,57.488232922231,65.0762222429013));
#17395=CARTESIAN_POINT('Ctrl Pts',(159.272002630726,59.4716702238614,65.7637685033219));
#17396=CARTESIAN_POINT('Ctrl Pts',(156.984757165518,65.3726819287223,67.8063284591325));
#17397=CARTESIAN_POINT('Ctrl Pts',(155.317165023605,69.2410214317241,69.1413108297163));
#17398=CARTESIAN_POINT('Ctrl Pts',(149.887841477183,80.6510891236089,73.0627350000645));
#17399=CARTESIAN_POINT('Ctrl Pts',(145.702324214992,87.9989448939223,75.5667325529025));
#17400=CARTESIAN_POINT('Ctrl Pts',(139.729767240726,96.8511925371005,78.5342884232701));
#17401=CARTESIAN_POINT('Ctrl Pts',(138.498003901055,98.604927815123,79.1195924508518));
#17402=CARTESIAN_POINT('Ctrl Pts',(136.593151713623,101.210019876689,79.9844850983316));
#17403=CARTESIAN_POINT('Ctrl Pts',(135.948034234115,102.074941840187,80.2708709224333));
#17404=CARTESIAN_POINT('Ctrl Pts',(134.642784559476,103.790569561344,80.837287641356));
#17405=CARTESIAN_POINT('Ctrl Pts',(133.982461046718,104.641574331305,81.117419484298));
#17406=CARTESIAN_POINT('Ctrl Pts',(130.642458316523,108.862717363317,82.5025158428281));
#17407=CARTESIAN_POINT('Ctrl Pts',(127.847811255468,112.131361115642,83.5609252410729));
#17408=CARTESIAN_POINT('Ctrl Pts',(122.012996265914,118.453930836736,85.5717401251865));
#17409=CARTESIAN_POINT('Ctrl Pts',(118.972841259923,121.507859522579,86.5241790265868));
#17410=CARTESIAN_POINT('Ctrl Pts',(112.641836965441,127.399032367865,88.3125256163411));
#17411=CARTESIAN_POINT('Ctrl Pts',(109.351021141409,130.236292245747,89.1484916842017));
#17412=CARTESIAN_POINT('Ctrl Pts',(104.218688827331,134.325162608347,90.3032259939414));
#17413=CARTESIAN_POINT('Ctrl Pts',(102.474476255975,135.660766282279,90.6716939178001));
#17414=CARTESIAN_POINT('Ctrl Pts',(98.921480159219,138.272927774531,91.3722444352154));
#17415=CARTESIAN_POINT('Ctrl Pts',(97.122876159534,139.542038720585,91.702332993713));
#17416=CARTESIAN_POINT('Ctrl Pts',(91.6611011033309,143.239579445468,92.6294671833747));
#17417=CARTESIAN_POINT('Ctrl Pts',(87.9320862659756,145.558387389969,93.1636516044368));
#17418=CARTESIAN_POINT('Ctrl Pts',(80.2974529965281,149.905353396487,94.044773738069));
#17419=CARTESIAN_POINT('Ctrl Pts',(76.3918510029905,151.933518732781,94.3918381893336));
#17420=CARTESIAN_POINT('Ctrl Pts',(68.3991059160043,155.695444133984,94.8693319054603));
#17421=CARTESIAN_POINT('Ctrl Pts',(64.3120020922313,157.429233145195,95.));
#17422=CARTESIAN_POINT('Ctrl Pts',(60.1292596944772,159.010918268508,95.));
#17423=CARTESIAN_POINT('',(-13.3842538190363,169.472303783561,95.));
#17424=CARTESIAN_POINT('Origin',(0.,0.,95.));
#17425=CARTESIAN_POINT('Ctrl Pts',(-13.3842538190363,169.472303783561,95.));
#17426=CARTESIAN_POINT('Ctrl Pts',(-16.3602967714103,169.237267654579,95.));
#17427=CARTESIAN_POINT('Ctrl Pts',(-19.3081742236088,168.925670678062,94.9062326532765));
#17428=CARTESIAN_POINT('Ctrl Pts',(-22.2278148953825,168.540593873598,94.7143704136405));
#17429=CARTESIAN_POINT('Ctrl Pts',(-23.3889397061482,168.387450976242,94.6380678710557));
#17430=CARTESIAN_POINT('Ctrl Pts',(-24.545598563398,168.222686262647,94.5462511008142));
#17431=CARTESIAN_POINT('Ctrl Pts',(-25.6977869660726,168.046492807987,94.4386500863327));
#17432=CARTESIAN_POINT('Ctrl Pts',(-25.8082073233279,168.029607249892,94.428338107465));
#17433=CARTESIAN_POINT('Ctrl Pts',(-25.9185866942024,168.012616663519,94.417881455326));
#17434=CARTESIAN_POINT('Ctrl Pts',(-26.0289250306962,167.995521189932,94.4072795523634));
#17435=CARTESIAN_POINT('Ctrl Pts',(-28.1898062203598,167.66072107896,94.1996504234983));
#17436=CARTESIAN_POINT('Ctrl Pts',(-30.3349411351003,167.28569316815,93.9363563245313));
#17437=CARTESIAN_POINT('Ctrl Pts',(-32.4638933110135,166.871514180024,93.6130702105055));
#17438=CARTESIAN_POINT('Ctrl Pts',(-34.221408510367,166.529596745184,93.3461876259324));
#17439=CARTESIAN_POINT('Ctrl Pts',(-35.9678952264575,166.160997957463,93.0384211810286));
#17440=CARTESIAN_POINT('Ctrl Pts',(-37.7031085064815,165.766328332842,92.6873629078737));
#17441=CARTESIAN_POINT('Ctrl Pts',(-37.9092616110374,165.719439359984,92.6456552090426));
#17442=CARTESIAN_POINT('Ctrl Pts',(-38.1152551687545,165.672182239619,92.6033333314582));
#17443=CARTESIAN_POINT('Ctrl Pts',(-38.3210884337155,165.624557972509,92.5603906152076));
#17444=CARTESIAN_POINT('Ctrl Pts',(-40.0879915027861,165.215744247801,92.1917640127398));
#17445=CARTESIAN_POINT('Ctrl Pts',(-41.8430834916924,164.779875427169,91.7774366479129));
#17446=CARTESIAN_POINT('Ctrl Pts',(-43.5858629304468,164.317596600633,91.3132064962846));
#17447=CARTESIAN_POINT('Ctrl Pts',(-43.8340397160827,164.251766771175,91.2470987925417));
#17448=CARTESIAN_POINT('Ctrl Pts',(-44.0819665865614,164.185401421503,91.179977322963));
#17449=CARTESIAN_POINT('Ctrl Pts',(-44.3296416785955,164.118502515818,91.1118266024519));
#17450=CARTESIAN_POINT('Ctrl Pts',(-45.0538775881994,163.922880948011,90.9125445565501));
#17451=CARTESIAN_POINT('Ctrl Pts',(-45.7760781643882,163.722663714208,90.7044316798228));
#17452=CARTESIAN_POINT('Ctrl Pts',(-46.4958413663918,163.518001258673,90.4872126994076));
#17453=CARTESIAN_POINT('Ctrl Pts',(-46.7634084940561,163.441919367829,90.4064630049218));
#17454=CARTESIAN_POINT('Ctrl Pts',(-47.0307617265755,163.365185663339,90.3244129008275));
#17455=CARTESIAN_POINT('Ctrl Pts',(-47.2977613961294,163.287845073462,90.2410869824901));
#17456=CARTESIAN_POINT('Ctrl Pts',(-47.8655785725555,163.12336803332,90.0638811913652));
#17457=CARTESIAN_POINT('Ctrl Pts',(-48.4324760349077,162.955947512629,89.8806886779588));
#17458=CARTESIAN_POINT('Ctrl Pts',(-48.9967296166451,162.786117367686,89.6918458325172));
#17459=CARTESIAN_POINT('Ctrl Pts',(-49.1257349206187,162.747289099366,89.6486706902267));
#17460=CARTESIAN_POINT('Ctrl Pts',(-49.2546020849577,162.708334961929,89.6052003831832));
#17461=CARTESIAN_POINT('Ctrl Pts',(-49.383310644726,162.669261477904,89.5614392605881));
#17462=CARTESIAN_POINT('Ctrl Pts',(-49.6684474558472,162.582699335851,89.4644922745422));
#17463=CARTESIAN_POINT('Ctrl Pts',(-49.9526798261573,162.495592644993,89.3661699692017));
#17464=CARTESIAN_POINT('Ctrl Pts',(-50.2359343342916,162.407976313914,89.2664815691616));
#17465=CARTESIAN_POINT('Ctrl Pts',(-51.5020145058062,162.016352186871,88.8208981697932));
#17466=CARTESIAN_POINT('Ctrl Pts',(-52.7500857914976,161.614076535672,88.3475284276466));
#17467=CARTESIAN_POINT('Ctrl Pts',(-53.9798246569649,161.202290116088,87.8449659507344));
#17468=CARTESIAN_POINT('Ctrl Pts',(-54.325413657281,161.086567289816,87.7037326622131));
#17469=CARTESIAN_POINT('Ctrl Pts',(-54.669554935815,160.970093287806,87.5601941484649));
#17470=CARTESIAN_POINT('Ctrl Pts',(-55.0122415374991,160.852893293963,87.4143198954764));
#17471=CARTESIAN_POINT('Ctrl Pts',(-56.13874522836,160.467625165638,86.934791709707));
#17472=CARTESIAN_POINT('Ctrl Pts',(-57.2495354683247,160.074505380291,86.4300424847287));
#17473=CARTESIAN_POINT('Ctrl Pts',(-58.3441670040107,159.67453463909,85.8984368616859));
#17474=CARTESIAN_POINT('Ctrl Pts',(-59.0405329442612,159.420087373331,85.5602481310819));
#17475=CARTESIAN_POINT('Ctrl Pts',(-59.7303596715798,159.162867298507,85.2111914083026));
#17476=CARTESIAN_POINT('Ctrl Pts',(-60.4135358107492,158.903129896419,84.8508559644503));
#17477=CARTESIAN_POINT('Ctrl Pts',(-60.7310756209656,158.782404126538,84.6833722923855));
#17478=CARTESIAN_POINT('Ctrl Pts',(-61.0471798789429,158.661133474286,84.5134557611085));
#17479=CARTESIAN_POINT('Ctrl Pts',(-61.3618299268532,158.539348482521,84.3410435386296));
#17480=CARTESIAN_POINT('Ctrl Pts',(-62.2894869232013,158.180299753905,83.8327346872544));
#17481=CARTESIAN_POINT('Ctrl Pts',(-63.2045107694617,157.816777747238,83.3027807982613));
#17482=CARTESIAN_POINT('Ctrl Pts',(-64.1063866299605,157.449578057315,82.7495954719335));
#17483=CARTESIAN_POINT('Ctrl Pts',(-64.5997003097787,157.248724882063,82.4470107139811));
#17484=CARTESIAN_POINT('Ctrl Pts',(-65.0890804065802,157.046771276094,82.1374760952267));
#17485=CARTESIAN_POINT('Ctrl Pts',(-65.5744442404841,156.843846747502,81.820738416781));
#17486=CARTESIAN_POINT('Ctrl Pts',(-65.890670864759,156.711636363915,81.6143759319004));
#17487=CARTESIAN_POINT('Ctrl Pts',(-66.2051893463786,156.579016099359,81.4049462447273));
#17488=CARTESIAN_POINT('Ctrl Pts',(-66.5179674014292,156.446028480324,81.1923519764314));
#17489=CARTESIAN_POINT('Ctrl Pts',(-67.0362519774947,156.22566317451,80.8400755668865));
#17490=CARTESIAN_POINT('Ctrl Pts',(-67.5499166828611,156.004220985238,80.4790186029946));
#17491=CARTESIAN_POINT('Ctrl Pts',(-68.0586509128982,155.781963127688,80.1088529719505));
#17492=CARTESIAN_POINT('Ctrl Pts',(-68.3697825255568,155.646034696766,79.8824671246112));
#17493=CARTESIAN_POINT('Ctrl Pts',(-68.678883121499,155.50987721189,79.6527834047028));
#17494=CARTESIAN_POINT('Ctrl Pts',(-68.9855269800791,155.373726306775,79.4200399155403));
#17495=CARTESIAN_POINT('Ctrl Pts',(-69.4459231453065,155.169308860109,79.0705980242588));
#17496=CARTESIAN_POINT('Ctrl Pts',(-69.9004164530957,154.965069720224,78.7145458423159));
#17497=CARTESIAN_POINT('Ctrl Pts',(-70.3480524083544,154.761595478826,78.3523496618931));
#17498=CARTESIAN_POINT('Ctrl Pts',(-70.3867057728156,154.744025478206,78.3210740219363));
#17499=CARTESIAN_POINT('Ctrl Pts',(-70.4253080005176,154.726461174113,78.2897525398122));
#17500=CARTESIAN_POINT('Ctrl Pts',(-70.463858472605,154.708902940828,78.2583854988648));
#17501=CARTESIAN_POINT('Ctrl Pts',(-70.762416999286,154.572921201129,78.0154598737167));
#17502=CARTESIAN_POINT('Ctrl Pts',(-71.0581493646474,154.437181403389,77.7696245694438));
#17503=CARTESIAN_POINT('Ctrl Pts',(-71.3511110895723,154.301710155538,77.5207217504554));
#17504=CARTESIAN_POINT('Ctrl Pts',(-72.0300168261834,153.987770826653,76.9439175562788));
#17505=CARTESIAN_POINT('Ctrl Pts',(-72.6935068910743,153.675521193897,76.351201597096));
#17506=CARTESIAN_POINT('Ctrl Pts',(-73.3411064736323,153.365835369114,75.741687555929));
#17507=CARTESIAN_POINT('Ctrl Pts',(-73.8881569515263,153.104232701343,75.2268092939844));
#17508=CARTESIAN_POINT('Ctrl Pts',(-74.4238686181605,152.844459258757,74.699944915077));
#17509=CARTESIAN_POINT('Ctrl Pts',(-74.9479655229901,152.587032424301,74.1605856133349));
#17510=CARTESIAN_POINT('Ctrl Pts',(-75.2087163460111,152.458956378948,73.8922413805464));
#17511=CARTESIAN_POINT('Ctrl Pts',(-75.4665990358862,152.33145637757,73.6208150897529));
#17512=CARTESIAN_POINT('Ctrl Pts',(-75.7215484874426,152.204616299458,73.3461973876455));
#17513=CARTESIAN_POINT('Ctrl Pts',(-76.322479956938,151.905646468125,72.6989066471895));
#17514=CARTESIAN_POINT('Ctrl Pts',(-76.9070841752639,151.610359645666,72.0340893553267));
#17515=CARTESIAN_POINT('Ctrl Pts',(-77.4746362476924,151.319781418506,71.3502680491987));
#17516=CARTESIAN_POINT('Ctrl Pts',(-77.9832035397331,151.05940252238,70.7375151992105));
#17517=CARTESIAN_POINT('Ctrl Pts',(-78.4780791420081,150.802803992481,70.1095037375267));
#17518=CARTESIAN_POINT('Ctrl Pts',(-78.9587508849806,150.550707931619,69.4652010508605));
#17519=CARTESIAN_POINT('Ctrl Pts',(-79.168166589072,150.440876482494,69.1844957613384));
#17520=CARTESIAN_POINT('Ctrl Pts',(-79.3750144085231,150.331828466866,68.9004120357299));
#17521=CARTESIAN_POINT('Ctrl Pts',(-79.5788665952709,150.223838104592,68.6134266440515));
#17522=CARTESIAN_POINT('Ctrl Pts',(-79.9006718636303,150.053362290393,68.1603855829883));
#17523=CARTESIAN_POINT('Ctrl Pts',(-80.2149120831088,149.885575415521,67.7002696808478));
#17524=CARTESIAN_POINT('Ctrl Pts',(-80.5200023905008,149.721503208657,67.2348659577922));
#17525=CARTESIAN_POINT('Ctrl Pts',(-80.6006857382064,149.678113121872,67.1117865629343));
#17526=CARTESIAN_POINT('Ctrl Pts',(-80.6807292784571,149.634982740388,66.9883371043634));
#17527=CARTESIAN_POINT('Ctrl Pts',(-80.7601039316535,149.592130852357,66.8645501211407));
#17528=CARTESIAN_POINT('Ctrl Pts',(-80.9373628184296,149.496434333849,66.5881099483674));
#17529=CARTESIAN_POINT('Ctrl Pts',(-81.1114879618528,149.402022980671,66.3097454001126));
#17530=CARTESIAN_POINT('Ctrl Pts',(-81.2824610346225,149.308946880817,66.0294022553307));
#17531=CARTESIAN_POINT('Ctrl Pts',(-81.6641120200211,149.101179747369,65.4036122655823));
#17532=CARTESIAN_POINT('Ctrl Pts',(-82.0300183432883,148.900087324285,64.7680540995119));
#17533=CARTESIAN_POINT('Ctrl Pts',(-82.3798221155295,148.706304197954,64.1223741806755));
#17534=CARTESIAN_POINT('Ctrl Pts',(-82.5222365974763,148.627409898532,63.8595005971364));
#17535=CARTESIAN_POINT('Ctrl Pts',(-82.6619832251089,148.549726352339,63.5949503331329));
#17536=CARTESIAN_POINT('Ctrl Pts',(-82.7990243480897,148.473302833396,63.3286896484053));
#17537=CARTESIAN_POINT('Ctrl Pts',(-83.1522801825168,148.276303178352,62.6423398994197));
#17538=CARTESIAN_POINT('Ctrl Pts',(-83.4875625884937,148.087674689848,61.9446586895439));
#17539=CARTESIAN_POINT('Ctrl Pts',(-83.8042673895934,147.908230897748,61.2351072858843));
#17540=CARTESIAN_POINT('Ctrl Pts',(-84.0985651096953,147.741482876506,60.5757571286811));
#17541=CARTESIAN_POINT('Ctrl Pts',(-84.3768294699192,147.582661074393,59.9061636400998));
#17542=CARTESIAN_POINT('Ctrl Pts',(-84.6383399601401,147.432532301283,59.2257173412033));
#17543=CARTESIAN_POINT('Ctrl Pts',(-84.7699435606084,147.356980888188,58.8832867840793));
#17544=CARTESIAN_POINT('Ctrl Pts',(-84.8973046834799,147.283630599417,58.5381081607792));
#17545=CARTESIAN_POINT('Ctrl Pts',(-85.0203346904952,147.212576531754,58.1901066250535));
#17546=CARTESIAN_POINT('Ctrl Pts',(-85.0952405390784,147.169315823552,57.9782286371204));
#17547=CARTESIAN_POINT('Ctrl Pts',(-85.1686045115591,147.126868896399,57.7650647152473));
#17548=CARTESIAN_POINT('Ctrl Pts',(-85.2402620956793,147.085341132009,57.5510665884564));
#17549=CARTESIAN_POINT('Ctrl Pts',(-85.3452374681436,147.024504688973,57.2375682568791));
#17550=CARTESIAN_POINT('Ctrl Pts',(-85.4465991137606,146.96561284564,56.9221345842854));
#17551=CARTESIAN_POINT('Ctrl Pts',(-85.5438296400012,146.908996356665,56.6061514339965));
#17552=CARTESIAN_POINT('Ctrl Pts',(-85.7077466516527,146.813548907784,56.0734482210215));
#17553=CARTESIAN_POINT('Ctrl Pts',(-85.8602690201768,146.724370794082,55.5383934624432));
#17554=CARTESIAN_POINT('Ctrl Pts',(-86.0014326176293,146.641582055417,55.0009151052429));
#17555=CARTESIAN_POINT('Ctrl Pts',(-86.0457044679173,146.615617779146,54.8323506750891));
#17556=CARTESIAN_POINT('Ctrl Pts',(-86.088860270053,146.590281706134,54.6635481162933));
#17557=CARTESIAN_POINT('Ctrl Pts',(-86.1308986805349,146.5655780796,54.4945046808591));
#17558=CARTESIAN_POINT('Ctrl Pts',(-86.35758732035,146.432365823636,53.5829519839561));
#17559=CARTESIAN_POINT('Ctrl Pts',(-86.5517922493526,146.317539877232,52.6644417912851));
#17560=CARTESIAN_POINT('Ctrl Pts',(-86.7132062820898,146.221817306037,51.7388579964434));
#17561=CARTESIAN_POINT('Ctrl Pts',(-86.7337856955697,146.209613197519,51.6208510840248));
#17562=CARTESIAN_POINT('Ctrl Pts',(-86.7538322187789,146.197719546278,51.5027292367629));
#17563=CARTESIAN_POINT('Ctrl Pts',(-86.7733441493221,146.186138071075,51.3844919987536));
#17564=CARTESIAN_POINT('Ctrl Pts',(-86.9358369512435,146.089689062511,50.3998277671451));
#17565=CARTESIAN_POINT('Ctrl Pts',(-87.0612765053318,146.014877687189,49.4071627883501));
#17566=CARTESIAN_POINT('Ctrl Pts',(-87.1487224382178,145.962667067261,48.406261267487));
#17567=CARTESIAN_POINT('Ctrl Pts',(-87.2321973497412,145.912827392215,47.4508118470259));
#17568=CARTESIAN_POINT('Ctrl Pts',(-87.2810611497313,145.883578565544,46.4878534783608));
#17569=CARTESIAN_POINT('Ctrl Pts',(-87.293883511954,145.875900574328,45.5170658868486));
#17570=CARTESIAN_POINT('Ctrl Pts',(-87.2961567586591,145.874539361165,45.3449572179969));
#17571=CARTESIAN_POINT('Ctrl Pts',(-87.2972972972612,145.873856069529,45.1726025028241));
#17572=CARTESIAN_POINT('Ctrl Pts',(-87.2972972972973,145.873856069507,45.0000000000001));
#17573=CARTESIAN_POINT('',(-13.3842538190364,169.472303783561,-95.));
#17574=CARTESIAN_POINT('Ctrl Pts',(-87.2972972972973,145.873856069507,-45.));
#17575=CARTESIAN_POINT('Ctrl Pts',(-87.2972972972127,145.873856069558,-45.9848836362899));
#17576=CARTESIAN_POINT('Ctrl Pts',(-87.2601578418064,145.896106375359,-46.9618714459115));
#17577=CARTESIAN_POINT('Ctrl Pts',(-87.1873161145765,145.939618737676,-47.9312779503657));
#17578=CARTESIAN_POINT('Ctrl Pts',(-87.1753834170317,145.946746792964,-48.0900830069663));
#17579=CARTESIAN_POINT('Ctrl Pts',(-87.1624927075728,145.954445375665,-48.2486846405294));
#17580=CARTESIAN_POINT('Ctrl Pts',(-87.1486504118183,145.962710071443,-48.4070842669367));
#17581=CARTESIAN_POINT('Ctrl Pts',(-87.0614449138588,146.014777078506,-49.4049908672901));
#17582=CARTESIAN_POINT('Ctrl Pts',(-86.9364575008243,146.089318977909,-50.3948826080192));
#17583=CARTESIAN_POINT('Ctrl Pts',(-86.7745829867444,146.185402758173,-51.376980415473));
#17584=CARTESIAN_POINT('Ctrl Pts',(-86.7545092707146,146.197317904488,-51.4987682868518));
#17585=CARTESIAN_POINT('Ctrl Pts',(-86.7338679528499,146.209564522444,-51.6204362722608));
#17586=CARTESIAN_POINT('Ctrl Pts',(-86.7126608231955,146.222140775472,-51.7419848435814));
#17587=CARTESIAN_POINT('Ctrl Pts',(-86.55193500937,146.31745440517,-52.6631841460454));
#17588=CARTESIAN_POINT('Ctrl Pts',(-86.3587024471325,146.431705790483,-53.5775217053184));
#17589=CARTESIAN_POINT('Ctrl Pts',(-86.1332375713659,146.564203662116,-54.4851039931522));
#17590=CARTESIAN_POINT('Ctrl Pts',(-86.0899027947026,146.589670004295,-54.6595430298897));
#17591=CARTESIAN_POINT('Ctrl Pts',(-86.0453761108919,146.615811080381,-54.8337323062595));
#17592=CARTESIAN_POINT('Ctrl Pts',(-85.9996595589194,146.642621893329,-55.0076726367092));
#17593=CARTESIAN_POINT('Ctrl Pts',(-85.9107555125789,146.694760334527,-55.3459308502346));
#17594=CARTESIAN_POINT('Ctrl Pts',(-85.8173466193961,146.749432661039,-55.6832465331334));
#17595=CARTESIAN_POINT('Ctrl Pts',(-85.71942978857,146.806605547736,-56.0196221499469));
#17596=CARTESIAN_POINT('Ctrl Pts',(-85.6615625704552,146.840393772669,-56.2184145436795));
#17597=CARTESIAN_POINT('Ctrl Pts',(-85.602098822783,146.87506822937,-56.4169525834863));
#17598=CARTESIAN_POINT('Ctrl Pts',(-85.5410516857225,146.910613900087,-56.6151812431414));
#17599=CARTESIAN_POINT('Ctrl Pts',(-85.445683233865,146.966143704592,-56.9248560501086));
#17600=CARTESIAN_POINT('Ctrl Pts',(-85.3464897727364,147.023775596745,-57.2335577883328));
#17601=CARTESIAN_POINT('Ctrl Pts',(-85.2439494976614,147.083204214466,-57.5400724674477));
#17602=CARTESIAN_POINT('Ctrl Pts',(-85.1701205745959,147.125992775765,-57.7607628122539));
#17603=CARTESIAN_POINT('Ctrl Pts',(-85.0944922004626,147.169750155055,-57.9805153356884));
#17604=CARTESIAN_POINT('Ctrl Pts',(-85.0172143876343,147.214378570055,-58.1989426996576));
#17605=CARTESIAN_POINT('Ctrl Pts',(-84.7981706813637,147.340877665574,-58.8180743443513));
#17606=CARTESIAN_POINT('Ctrl Pts',(-84.5652672651916,147.474731098872,-59.4286784047483));
#17607=CARTESIAN_POINT('Ctrl Pts',(-84.3190010331543,147.615399903826,-60.0310545986629));
#17608=CARTESIAN_POINT('Ctrl Pts',(-84.1522200733756,147.710666226403,-60.4390069148932));
#17609=CARTESIAN_POINT('Ctrl Pts',(-83.9793110000177,147.809057875933,-60.8431861352841));
#17610=CARTESIAN_POINT('Ctrl Pts',(-83.8004373335544,147.9104009281,-61.2436928500744));
#17611=CARTESIAN_POINT('Ctrl Pts',(-83.5213153281546,148.068540896455,-61.8686604018594));
#17612=CARTESIAN_POINT('Ctrl Pts',(-83.227660732651,148.233872659777,-62.4846786679934));
#17613=CARTESIAN_POINT('Ctrl Pts',(-82.9199078493258,148.405825476924,-63.0919942464788));
#17614=CARTESIAN_POINT('Ctrl Pts',(-82.8826975341711,148.426616244011,-63.1654246034251));
#17615=CARTESIAN_POINT('Ctrl Pts',(-82.8452811563684,148.447503775454,-63.2387277690164));
#17616=CARTESIAN_POINT('Ctrl Pts',(-82.8076595183652,148.468487038094,-63.3119042074312));
#17617=CARTESIAN_POINT('Ctrl Pts',(-82.6657598925264,148.547630777586,-63.5879078527379));
#17618=CARTESIAN_POINT('Ctrl Pts',(-82.5209294596415,148.628142417463,-63.8621216215528));
#17619=CARTESIAN_POINT('Ctrl Pts',(-82.3732072730211,148.709968474063,-64.1345800057147));
#17620=CARTESIAN_POINT('Ctrl Pts',(-82.0282675642021,148.901036970834,-64.7707858313133));
#17621=CARTESIAN_POINT('Ctrl Pts',(-81.6675541821605,149.099276572551,-65.3974150592188));
#17622=CARTESIAN_POINT('Ctrl Pts',(-81.2913777116218,149.304092491018,-66.0147759266973));
#17623=CARTESIAN_POINT('Ctrl Pts',(-81.1136958590786,149.400834511515,-66.3063779571596));
#17624=CARTESIAN_POINT('Ctrl Pts',(-80.932568038796,149.499041513155,-66.5958998850957));
#17625=CARTESIAN_POINT('Ctrl Pts',(-80.7480156183748,149.59865632316,-66.8833928168321));
#17626=CARTESIAN_POINT('Ctrl Pts',(-80.4944836312975,149.735503841415,-67.2783410601955));
#17627=CARTESIAN_POINT('Ctrl Pts',(-80.2341755442533,149.875171570879,-67.6698536656852));
#17628=CARTESIAN_POINT('Ctrl Pts',(-79.9689674067322,150.016546384168,-68.0554758763857));
#17629=CARTESIAN_POINT('Ctrl Pts',(-79.9345638834303,150.034885910733,-68.1054998418476));
#17630=CARTESIAN_POINT('Ctrl Pts',(-79.9000779383347,150.053254141627,-68.1554246256358));
#17631=CARTESIAN_POINT('Ctrl Pts',(-79.8655136998482,150.071648626446,-68.2052448161789));
#17632=CARTESIAN_POINT('Ctrl Pts',(-79.7739999236149,150.120350661883,-68.3371509124479));
#17633=CARTESIAN_POINT('Ctrl Pts',(-79.6818941936877,150.16926027239,-68.46839508031));
#17634=CARTESIAN_POINT('Ctrl Pts',(-79.5892012521672,150.218371135719,-68.5989889747242));
#17635=CARTESIAN_POINT('Ctrl Pts',(-79.3779141702089,150.330315916359,-68.8966686299355));
#17636=CARTESIAN_POINT('Ctrl Pts',(-79.163579340244,150.443304640525,-69.1909515362395));
#17637=CARTESIAN_POINT('Ctrl Pts',(-78.9462744635298,150.557250733189,-69.4819552440033));
#17638=CARTESIAN_POINT('Ctrl Pts',(-78.484031024483,150.799632931579,-70.1009682946354));
#17639=CARTESIAN_POINT('Ctrl Pts',(-78.0084220634587,151.04629879067,-70.7052523960841));
#17640=CARTESIAN_POINT('Ctrl Pts',(-77.5199570397094,151.296570144028,-71.2955928713244));
#17641=CARTESIAN_POINT('Ctrl Pts',(-77.0216110413805,151.55190414212,-71.8978751211965));
#17642=CARTESIAN_POINT('Ctrl Pts',(-76.5098835991764,151.810990946169,-72.4856440211327));
#17643=CARTESIAN_POINT('Ctrl Pts',(-75.9853380432724,152.073093135985,-73.0597795388602));
#17644=CARTESIAN_POINT('Ctrl Pts',(-75.9066252473747,152.112423935644,-73.1459337561934));
#17645=CARTESIAN_POINT('Ctrl Pts',(-75.827623857029,152.151822604378,-73.23178106206));
#17646=CARTESIAN_POINT('Ctrl Pts',(-75.7483358179058,152.19128661854,-73.3173245146471));
#17647=CARTESIAN_POINT('Ctrl Pts',(-75.4824265393875,152.323637571463,-73.6042126507511));
#17648=CARTESIAN_POINT('Ctrl Pts',(-75.2132781171718,152.456731033711,-73.8876629525089));
#17649=CARTESIAN_POINT('Ctrl Pts',(-74.9409623838955,152.590472038921,-74.1677942224948));
#17650=CARTESIAN_POINT('Ctrl Pts',(-74.3167866632673,152.897020203802,-74.8098839585897));
#17651=CARTESIAN_POINT('Ctrl Pts',(-73.6759323983567,153.206997438947,-75.4344770901284));
#17652=CARTESIAN_POINT('Ctrl Pts',(-73.0188468713402,153.519527171665,-76.0423970896734));
#17653=CARTESIAN_POINT('Ctrl Pts',(-72.4866598929599,153.772651380418,-76.5347639039658));
#17654=CARTESIAN_POINT('Ctrl Pts',(-71.9438260409974,154.027449586919,-77.0161946043035));
#17655=CARTESIAN_POINT('Ctrl Pts',(-71.390591833358,154.283447572611,-77.4871484354879));
#17656=CARTESIAN_POINT('Ctrl Pts',(-71.0824660574145,154.426026568798,-77.7494478606924));
#17657=CARTESIAN_POINT('Ctrl Pts',(-70.7712601794406,154.568910483264,-78.0083517875374));
#17658=CARTESIAN_POINT('Ctrl Pts',(-70.4568502021148,154.712094742454,-78.2640882514698));
#17659=CARTESIAN_POINT('Ctrl Pts',(-70.0593478034779,154.893119807115,-78.5874108721342));
#17660=CARTESIAN_POINT('Ctrl Pts',(-69.6561647078897,155.074868533276,-78.9060258939702));
#17661=CARTESIAN_POINT('Ctrl Pts',(-69.248163363783,155.256846802623,-79.2194748965191));
#17662=CARTESIAN_POINT('Ctrl Pts',(-69.1753983116225,155.289301740462,-79.2753769991704));
#17663=CARTESIAN_POINT('Ctrl Pts',(-69.1024799874813,155.321763950337,-79.3311146571456));
#17664=CARTESIAN_POINT('Ctrl Pts',(-69.0294132721225,155.354230585197,-79.3866850949249));
#17665=CARTESIAN_POINT('Ctrl Pts',(-68.7054569495941,155.498178093751,-79.6330680693873));
#17666=CARTESIAN_POINT('Ctrl Pts',(-68.3790872245564,155.64198899673,-79.8757795810431));
#17667=CARTESIAN_POINT('Ctrl Pts',(-68.0508366323766,155.785376828615,-80.1145376578703));
#17668=CARTESIAN_POINT('Ctrl Pts',(-67.5615807059302,155.999095701336,-80.470405421273));
#17669=CARTESIAN_POINT('Ctrl Pts',(-67.0679849322336,156.211965564659,-80.8177011119818));
#17670=CARTESIAN_POINT('Ctrl Pts',(-66.5698782490513,156.423946748387,-81.1570290898547));
#17671=CARTESIAN_POINT('Ctrl Pts',(-66.2383201338304,156.565049215211,-81.3828982632343));
#17672=CARTESIAN_POINT('Ctrl Pts',(-65.9048194379772,156.705733562974,-81.6051889022944));
#17673=CARTESIAN_POINT('Ctrl Pts',(-65.5694149143534,156.845949350922,-81.8240186527302));
#17674=CARTESIAN_POINT('Ctrl Pts',(-64.6829201703191,157.216548285317,-82.4023991155329));
#17675=CARTESIAN_POINT('Ctrl Pts',(-63.7831508540726,157.583856508053,-82.9566758456117));
#17676=CARTESIAN_POINT('Ctrl Pts',(-62.8706182035639,157.947089454461,-83.4884243400324));
#17677=CARTESIAN_POINT('Ctrl Pts',(-62.3950459017896,158.136390657335,-83.7655485123189));
#17678=CARTESIAN_POINT('Ctrl Pts',(-61.9160072268454,158.324584912065,-84.0365547854392));
#17679=CARTESIAN_POINT('Ctrl Pts',(-61.4335758366808,158.511560631034,-84.3016715534536));
#17680=CARTESIAN_POINT('Ctrl Pts',(-61.0961749032255,158.642326960506,-84.4870878568419));
#17681=CARTESIAN_POINT('Ctrl Pts',(-60.7571134074066,158.772497700688,-84.6696164130183));
#17682=CARTESIAN_POINT('Ctrl Pts',(-60.4164146176901,158.902035370161,-84.8493358861248));
#17683=CARTESIAN_POINT('Ctrl Pts',(-59.3438850557613,159.309823669053,-85.4150979421665));
#17684=CARTESIAN_POINT('Ctrl Pts',(-58.2551149681582,159.711350535676,-85.9529757040515));
#17685=CARTESIAN_POINT('Ctrl Pts',(-57.1505460201433,160.105633614135,-86.4645921180823));
#17686=CARTESIAN_POINT('Ctrl Pts',(-56.4487513530865,160.356143790318,-86.7896507498597));
#17687=CARTESIAN_POINT('Ctrl Pts',(-55.7405793567733,160.603729602651,-87.1041092869249));
#17688=CARTESIAN_POINT('Ctrl Pts',(-55.0261465205371,160.84813707073,-87.4083941820344));
#17689=CARTESIAN_POINT('Ctrl Pts',(-53.8092543837208,161.264435861881,-87.9266820845914));
#17690=CARTESIAN_POINT('Ctrl Pts',(-52.5741889959425,161.671522365092,-88.415424491364));
#17691=CARTESIAN_POINT('Ctrl Pts',(-51.321279392281,162.068275297191,-88.8760332304436));
#17692=CARTESIAN_POINT('Ctrl Pts',(-51.0020471261459,162.169365062358,-88.9933929913939));
#17693=CARTESIAN_POINT('Ctrl Pts',(-50.6816565051252,162.269783934374,-89.1089265816755));
#17694=CARTESIAN_POINT('Ctrl Pts',(-50.3601131347592,162.369513278003,-89.2226578573149));
#17695=CARTESIAN_POINT('Ctrl Pts',(-50.0449901630546,162.467251281727,-89.3341182102819));
#17696=CARTESIAN_POINT('Ctrl Pts',(-49.7287558621685,162.564328303438,-89.4438470825149));
#17697=CARTESIAN_POINT('Ctrl Pts',(-49.4114172566784,162.660726190096,-89.5518664732));
#17698=CARTESIAN_POINT('Ctrl Pts',(-48.5859802317114,162.911469035119,-89.8328382898754));
#17699=CARTESIAN_POINT('Ctrl Pts',(-47.7517061842026,163.15799803978,-90.1026104418408));
#17700=CARTESIAN_POINT('Ctrl Pts',(-46.9134264693539,163.398683586024,-90.3600730618877));
#17701=CARTESIAN_POINT('Ctrl Pts',(-46.7837842030723,163.435906268529,-90.3998903650557));
#17702=CARTESIAN_POINT('Ctrl Pts',(-46.6540462294582,163.47298916605,-90.4394132489993));
#17703=CARTESIAN_POINT('Ctrl Pts',(-46.5242305246109,163.509926224964,-90.4786376019946));
#17704=CARTESIAN_POINT('Ctrl Pts',(-45.8392025345838,163.704840386199,-90.6856216469843));
#17705=CARTESIAN_POINT('Ctrl Pts',(-45.1519736911824,163.89572719544,-90.8843501937075));
#17706=CARTESIAN_POINT('Ctrl Pts',(-44.4626074592405,164.082529655127,-91.0751334104582));
#17707=CARTESIAN_POINT('Ctrl Pts',(-44.1783869467075,164.159546904268,-91.153791895796));
#17708=CARTESIAN_POINT('Ctrl Pts',(-43.893801405373,164.235870359354,-91.2310993615674));
#17709=CARTESIAN_POINT('Ctrl Pts',(-43.608853696462,164.311496491514,-91.3070783228867));
#17710=CARTESIAN_POINT('Ctrl Pts',(-42.1660734698655,164.69441547869,-91.6917837955071));
#17711=CARTESIAN_POINT('Ctrl Pts',(-40.7140157437857,165.059455982243,-92.0424908351377));
#17712=CARTESIAN_POINT('Ctrl Pts',(-39.2529743664741,165.406179164334,-92.3614696565619));
#17713=CARTESIAN_POINT('Ctrl Pts',(-38.9827628953543,165.47030368713,-92.4204630142665));
#17714=CARTESIAN_POINT('Ctrl Pts',(-38.7122441503414,165.533801695374,-92.4783712680377));
#17715=CARTESIAN_POINT('Ctrl Pts',(-38.4414200000023,165.596670438918,-92.5352089701923));
#17716=CARTESIAN_POINT('Ctrl Pts',(-38.2001914433258,165.652668902299,-92.5858354628386));
#17717=CARTESIAN_POINT('Ctrl Pts',(-37.9587206663411,165.708168099145,-92.6356114700981));
#17718=CARTESIAN_POINT('Ctrl Pts',(-37.7170088289231,165.763166128676,-92.6845472946188));
#17719=CARTESIAN_POINT('Ctrl Pts',(-36.0211739040145,166.14902881656,-93.0278779365432));
#17720=CARTESIAN_POINT('Ctrl Pts',(-34.3135008475802,166.510233714585,-93.3300633545587));
#17721=CARTESIAN_POINT('Ctrl Pts',(-32.5942104457704,166.846108960576,-93.5932011303994));
#17722=CARTESIAN_POINT('Ctrl Pts',(-30.8504021259006,167.186773951074,-93.8600913790159));
#17723=CARTESIAN_POINT('Ctrl Pts',(-29.094642715236,167.501381720967,-94.0868124355136));
#17724=CARTESIAN_POINT('Ctrl Pts',(-27.3271657460881,167.789235416743,-94.27560615426));
#17725=CARTESIAN_POINT('Ctrl Pts',(-26.91682780789,167.856063609749,-94.319436555814));
#17726=CARTESIAN_POINT('Ctrl Pts',(-26.505858326992,167.921449818373,-94.3612229556582));
#17727=CARTESIAN_POINT('Ctrl Pts',(-26.0942602532882,167.985385353875,-94.4009938026451));
#17728=CARTESIAN_POINT('Ctrl Pts',(-25.9629814123699,168.005777536275,-94.4136786790533));
#17729=CARTESIAN_POINT('Ctrl Pts',(-25.8316384428103,168.02602217232,-94.4261573441815));
#17730=CARTESIAN_POINT('Ctrl Pts',(-25.7002314412141,168.046118978926,-94.4384308363077));
#17731=CARTESIAN_POINT('Ctrl Pts',(-23.7387849731355,168.346093941119,-94.6216311033371));
#17732=CARTESIAN_POINT('Ctrl Pts',(-21.7630551046537,168.613150513186,-94.7590226613957));
#17733=CARTESIAN_POINT('Ctrl Pts',(-19.7730895732306,168.846191178979,-94.8521329477807));
#17734=CARTESIAN_POINT('Ctrl Pts',(-18.7114479901565,168.970517785369,-94.9018070503103));
#17735=CARTESIAN_POINT('Ctrl Pts',(-17.6478952698206,169.084909038081,-94.9387840850485));
#17736=CARTESIAN_POINT('Ctrl Pts',(-16.5829228051783,169.189282687295,-94.9633322911818));
#17737=CARTESIAN_POINT('Ctrl Pts',(-15.517950340536,169.29365633651,-94.9878804973151));
#17738=CARTESIAN_POINT('Ctrl Pts',(-14.4515581849858,169.388012296297,-95.));
#17739=CARTESIAN_POINT('Ctrl Pts',(-13.3842538190364,169.472303783561,-95.));
#17740=CARTESIAN_POINT('',(60.1292596944771,159.010918268508,-95.));
#17741=CARTESIAN_POINT('Origin',(0.,0.,-95.));
#17742=CARTESIAN_POINT('Ctrl Pts',(60.1292596944771,159.010918268508,-95.));
#17743=CARTESIAN_POINT('Ctrl Pts',(64.3119987470806,157.429234410148,-95.));
#17744=CARTESIAN_POINT('Ctrl Pts',(68.3990993783209,155.695446906751,-94.8693321132271));
#17745=CARTESIAN_POINT('Ctrl Pts',(76.3918383640665,151.93352498582,-94.391839127194));
#17746=CARTESIAN_POINT('Ctrl Pts',(80.2974374490313,149.90536162208,-94.0447751990941));
#17747=CARTESIAN_POINT('Ctrl Pts',(87.9320651786579,145.558400023304,-93.1636543714777));
#17748=CARTESIAN_POINT('Ctrl Pts',(91.6610773848025,143.239594513987,-92.629470733653));
#17749=CARTESIAN_POINT('Ctrl Pts',(97.1228487062774,139.542057800314,-91.7023378918564));
#17750=CARTESIAN_POINT('Ctrl Pts',(98.9214514964918,138.272948251204,-91.372249811654));
#17751=CARTESIAN_POINT('Ctrl Pts',(102.474445246975,135.660789676228,-90.6717003069366));
#17752=CARTESIAN_POINT('Ctrl Pts',(104.218656939756,134.325187322145,-90.3032328616472));
#17753=CARTESIAN_POINT('Ctrl Pts',(109.350986406493,130.236321299975,-89.1485001127697));
#17754=CARTESIAN_POINT('Ctrl Pts',(112.641800518645,127.399064480377,-88.3125351604413));
#17755=CARTESIAN_POINT('Ctrl Pts',(118.972801758344,121.507898082088,-86.5241909359486));
#17756=CARTESIAN_POINT('Ctrl Pts',(122.012955421471,118.453972784964,-85.5717532843836));
#17757=CARTESIAN_POINT('Ctrl Pts',(127.847768104756,112.131410184014,-83.5609410285741));
#17758=CARTESIAN_POINT('Ctrl Pts',(130.642414202373,108.862770163068,-82.5025330088399));
#17759=CARTESIAN_POINT('Ctrl Pts',(133.982415980692,104.641632024445,-81.1174384551523));
#17760=CARTESIAN_POINT('Ctrl Pts',(134.642739315732,103.790628244652,-80.8373069772816));
#17761=CARTESIAN_POINT('Ctrl Pts',(135.947988660783,102.075002527314,-80.270890996809));
#17762=CARTESIAN_POINT('Ctrl Pts',(136.593106061479,101.210081480818,-79.9845055141404));
#17763=CARTESIAN_POINT('Ctrl Pts',(138.4979580987,98.604992114986,-79.1196138720762));
#17764=CARTESIAN_POINT('Ctrl Pts',(139.729721387279,96.8512586573184,-78.5343105220887));
#17765=CARTESIAN_POINT('Ctrl Pts',(145.702278354011,87.9990202333266,-75.566758076221));
#17766=CARTESIAN_POINT('Ctrl Pts',(149.887796395751,80.6511722105745,-73.062763378222));
#17767=CARTESIAN_POINT('Ctrl Pts',(155.317122432713,69.2411167663415,-69.1413436830464));
#17768=CARTESIAN_POINT('Ctrl Pts',(156.984715626498,65.3727814509462,-67.8063628366596));
#17769=CARTESIAN_POINT('Ctrl Pts',(159.271963035734,59.4717762008594,-65.7638052213179));
#17770=CARTESIAN_POINT('Ctrl Pts',(159.998649543538,57.488341079772,-65.0762597501037));
#17771=CARTESIAN_POINT('Ctrl Pts',(161.034620693271,54.4882578372571,-64.0350107773724));
#17772=CARTESIAN_POINT('Ctrl Pts',(161.371184461829,53.4832599490673,-63.6859889324587));
#17773=CARTESIAN_POINT('Ctrl Pts',(162.024054573491,51.4715844807547,-62.9869704073305));
#17774=CARTESIAN_POINT('Ctrl Pts',(162.340565299031,50.4643653454645,-62.6367861123213));
#17775=CARTESIAN_POINT('Ctrl Pts',(165.100688409562,41.3870343438974,-59.4792352470941));
#17776=CARTESIAN_POINT('Ctrl Pts',(166.928575054619,33.2308356969195,-56.6310812172013));
#17777=CARTESIAN_POINT('Ctrl Pts',(168.765868892532,20.8672206982357,-52.3070906459483));
#17778=CARTESIAN_POINT('Ctrl Pts',(169.226876637901,16.7243838271306,-50.8570487361151));
#17779=CARTESIAN_POINT('Ctrl Pts',(169.689684284876,10.477177341883,-48.6696274303821));
#17780=CARTESIAN_POINT('Ctrl Pts',(169.805796892358,8.38927803590911,-47.9384240498734));
#17781=CARTESIAN_POINT('Ctrl Pts',(169.922171669824,5.24907001896995,-46.8385881425543));
#17782=CARTESIAN_POINT('Ctrl Pts',(169.965906660215,3.67687569683897,-46.2879122489256));
#17783=CARTESIAN_POINT('Ctrl Pts',(169.991474952794,1.8389601147623,-45.6441423007187));
#17784=CARTESIAN_POINT('Ctrl Pts',(169.996957619285,1.05048782907507,-45.3679602834514));
#17785=CARTESIAN_POINT('Ctrl Pts',(169.999393685716,0.524662730744418,-45.1837767020228));
#17786=CARTESIAN_POINT('Ctrl Pts',(170.,0.260336526753546,-45.091189605798));
#17787=CARTESIAN_POINT('Ctrl Pts',(170.,0.,-45.));
#17788=CARTESIAN_POINT('',(145.36231884058,-88.1464478086873,-32.5));
#17789=CARTESIAN_POINT('Origin',(0.,0.,-32.5));
#17790=CARTESIAN_POINT('',(150.289855072464,-79.4541343310581,-37.5));
#17791=CARTESIAN_POINT('Ctrl Pts',(145.36231884058,-88.1464478086873,-32.5));
#17792=CARTESIAN_POINT('Ctrl Pts',(145.729245618505,-87.5413488102603,-32.5000000006552));
#17793=CARTESIAN_POINT('Ctrl Pts',(146.089427518266,-86.9388521048938,-32.5405483747626));
#17794=CARTESIAN_POINT('Ctrl Pts',(146.443059039059,-86.3390436926112,-32.6214654834413));
#17795=CARTESIAN_POINT('Ctrl Pts',(146.591729838526,-86.0868772681335,-32.6554839759412));
#17796=CARTESIAN_POINT('Ctrl Pts',(146.739242777582,-85.8351860206267,-32.6966381016031));
#17797=CARTESIAN_POINT('Ctrl Pts',(146.885611849037,-85.5839764893768,-32.744917216543));
#17798=CARTESIAN_POINT('Ctrl Pts',(146.887215711036,-85.5812238216389,-32.7454462424977));
#17799=CARTESIAN_POINT('Ctrl Pts',(146.888819435246,-85.578471212414,-32.745976138191));
#17800=CARTESIAN_POINT('Ctrl Pts',(146.890423021642,-85.5757186617923,-32.7465069043789));
#17801=CARTESIAN_POINT('Ctrl Pts',(147.136163003217,-85.1539068149984,-32.8278436340878));
#17802=CARTESIAN_POINT('Ctrl Pts',(147.378654044698,-84.7334926273371,-32.9296159558605));
#17803=CARTESIAN_POINT('Ctrl Pts',(147.617771548819,-84.3148475830954,-33.0545296220188));
#17804=CARTESIAN_POINT('Ctrl Pts',(147.619992196193,-84.3109596911514,-33.0556896759668));
#17805=CARTESIAN_POINT('Ctrl Pts',(147.622212556282,-84.307071941363,-33.0568517414269));
#17806=CARTESIAN_POINT('Ctrl Pts',(147.624432625828,-84.303184339794,-33.0580158203818));
#17807=CARTESIAN_POINT('Ctrl Pts',(147.797445356378,-84.0002188025685,-33.1487339147363));
#17808=CARTESIAN_POINT('Ctrl Pts',(147.968707325063,-83.6981287773935,-33.2516890850514));
#17809=CARTESIAN_POINT('Ctrl Pts',(148.136615102467,-83.3998939040528,-33.3677714304339));
#17810=CARTESIAN_POINT('Ctrl Pts',(148.200188499827,-83.2869759415708,-33.4117226349792));
#17811=CARTESIAN_POINT('Ctrl Pts',(148.263281189286,-83.1746104687379,-33.4575552147659));
#17812=CARTESIAN_POINT('Ctrl Pts',(148.325806750806,-83.0629583612556,-33.505315729073));
#17813=CARTESIAN_POINT('Ctrl Pts',(148.328437712999,-83.0582602431351,-33.5073254048666));
#17814=CARTESIAN_POINT('Ctrl Pts',(148.331067922545,-83.0535629380491,-33.5093386477995));
#17815=CARTESIAN_POINT('Ctrl Pts',(148.333697371915,-83.0488664605802,-33.5113554669624));
#17816=CARTESIAN_POINT('Ctrl Pts',(148.479392264039,-82.7886398192674,-33.6231051943638));
#17817=CARTESIAN_POINT('Ctrl Pts',(148.622808980514,-82.5308543501899,-33.7458732653459));
#17818=CARTESIAN_POINT('Ctrl Pts',(148.762663380364,-82.2779954794438,-33.8812204176226));
#17819=CARTESIAN_POINT('Ctrl Pts',(148.840976562993,-82.1364040604732,-33.9570097118165));
#17820=CARTESIAN_POINT('Ctrl Pts',(148.918172933482,-81.9963571593236,-34.0367425583452));
#17821=CARTESIAN_POINT('Ctrl Pts',(148.994029023493,-81.858288006606,-34.1206866444586));
#17822=CARTESIAN_POINT('Ctrl Pts',(148.996712266486,-81.8534041128196,-34.1236559825947));
#17823=CARTESIAN_POINT('Ctrl Pts',(148.999393672824,-81.8485229853464,-34.1266302098562));
#17824=CARTESIAN_POINT('Ctrl Pts',(149.002073232326,-81.8436446453384,-34.1296093604689));
#17825=CARTESIAN_POINT('Ctrl Pts',(149.107681065301,-81.6513776267186,-34.24702479387));
#17826=CARTESIAN_POINT('Ctrl Pts',(149.210443318176,-81.4633981454561,-34.3720951240627));
#17827=CARTESIAN_POINT('Ctrl Pts',(149.309720948425,-81.2810297213995,-34.5068954514884));
#17828=CARTESIAN_POINT('Ctrl Pts',(149.401996349968,-81.1115240682479,-34.6321880708852));
#17829=CARTESIAN_POINT('Ctrl Pts',(149.491261252783,-80.9468661109974,-34.7658868965042));
#17830=CARTESIAN_POINT('Ctrl Pts',(149.577013895292,-80.7880986855831,-34.9096181572236));
#17831=CARTESIAN_POINT('Ctrl Pts',(149.5835211508,-80.7760507746002,-34.9205250635371));
#17832=CARTESIAN_POINT('Ctrl Pts',(149.590008187532,-80.7640367724579,-34.9314897186423));
#17833=CARTESIAN_POINT('Ctrl Pts',(149.596474789369,-80.7520571291769,-34.94251282205));
#17834=CARTESIAN_POINT('Ctrl Pts',(149.598641974416,-80.7480423306098,-34.9462070505615));
#17835=CARTESIAN_POINT('Ctrl Pts',(149.600807137209,-80.7440308818108,-34.9499087160619));
#17836=CARTESIAN_POINT('Ctrl Pts',(149.602970226706,-80.7400228807505,-34.9536178068362));
#17837=CARTESIAN_POINT('Ctrl Pts',(149.665071318773,-80.6249554074952,-35.0601037326242));
#17838=CARTESIAN_POINT('Ctrl Pts',(149.72550324979,-80.5126559823695,-35.1727795475935));
#17839=CARTESIAN_POINT('Ctrl Pts',(149.783030801438,-80.4054929784085,-35.2913281843215));
#17840=CARTESIAN_POINT('Ctrl Pts',(149.809543927947,-80.3561040126055,-35.3459645266126));
#17841=CARTESIAN_POINT('Ctrl Pts',(149.835440369613,-80.3078056561145,-35.401847873638));
#17842=CARTESIAN_POINT('Ctrl Pts',(149.860600799429,-80.260826858674,-35.4589450748328));
#17843=CARTESIAN_POINT('Ctrl Pts',(149.862244464558,-80.2577578566055,-35.4626750857764));
#17844=CARTESIAN_POINT('Ctrl Pts',(149.863885113164,-80.2546942576159,-35.4664102868023));
#17845=CARTESIAN_POINT('Ctrl Pts',(149.865522721632,-80.2516361085806,-35.4701507147205));
#17846=CARTESIAN_POINT('Ctrl Pts',(149.920874283244,-80.1482699328262,-35.5965780814448));
#17847=CARTESIAN_POINT('Ctrl Pts',(149.972772946805,-80.0510921734565,-35.7290075001422));
#17848=CARTESIAN_POINT('Ctrl Pts',(150.020328326758,-79.9618719405058,-35.8689218234402));
#17849=CARTESIAN_POINT('Ctrl Pts',(150.04142343791,-79.92229469955,-35.9309864774229));
#17850=CARTESIAN_POINT('Ctrl Pts',(150.061664115497,-79.8842828909716,-35.9945234855749));
#17851=CARTESIAN_POINT('Ctrl Pts',(150.080973718749,-79.8479888765764,-36.0596598378906));
#17852=CARTESIAN_POINT('Ctrl Pts',(150.081910893431,-79.8462273783758,-36.0628211737006));
#17853=CARTESIAN_POINT('Ctrl Pts',(150.082845417364,-79.8444707888363,-36.0659847749909));
#17854=CARTESIAN_POINT('Ctrl Pts',(150.083777280819,-79.842719127427,-36.0691506505178));
#17855=CARTESIAN_POINT('Ctrl Pts',(150.124316972746,-79.766515029516,-36.2068785740439));
#17856=CARTESIAN_POINT('Ctrl Pts',(150.159836015383,-79.6996105779044,-36.3489635265317));
#17857=CARTESIAN_POINT('Ctrl Pts',(150.189536570947,-79.6436016305286,-36.4961016996745));
#17858=CARTESIAN_POINT('Ctrl Pts',(150.205994764959,-79.6125649679198,-36.5776364910011));
#17859=CARTESIAN_POINT('Ctrl Pts',(150.220666659912,-79.5848732537884,-36.6607227768373));
#17860=CARTESIAN_POINT('Ctrl Pts',(150.233419649245,-79.5607919801431,-36.7454773415068));
#17861=CARTESIAN_POINT('Ctrl Pts',(150.233653158554,-79.5603510481059,-36.747029211371));
#17862=CARTESIAN_POINT('Ctrl Pts',(150.233885994755,-79.5599113833124,-36.7485818022511));
#17863=CARTESIAN_POINT('Ctrl Pts',(150.234118156878,-79.5594729876405,-36.7501351076896));
#17864=CARTESIAN_POINT('Ctrl Pts',(150.243593980634,-79.541579629057,-36.8135341168033));
#17865=CARTESIAN_POINT('Ctrl Pts',(150.251930637624,-79.5258311439938,-36.8780113419661));
#17866=CARTESIAN_POINT('Ctrl Pts',(150.25908694937,-79.5123085902626,-36.9432880969468));
#17867=CARTESIAN_POINT('Ctrl Pts',(150.266133192885,-79.49899402126,-37.0075608575311));
#17868=CARTESIAN_POINT('Ctrl Pts',(150.272035277523,-79.4878371314995,-37.0726101138062));
#17869=CARTESIAN_POINT('Ctrl Pts',(150.276731655023,-79.4789572453976,-37.1381835195656));
#17870=CARTESIAN_POINT('Ctrl Pts',(150.281154338818,-79.4705948579247,-37.1999354632936));
#17871=CARTESIAN_POINT('Ctrl Pts',(150.284507727575,-79.4642518495709,-37.2621532653189));
#17872=CARTESIAN_POINT('Ctrl Pts',(150.286719886614,-79.4600667280323,-37.3246214692043));
#17873=CARTESIAN_POINT('Ctrl Pts',(150.28878458935,-79.4561605749315,-37.3829257182103));
#17874=CARTESIAN_POINT('Ctrl Pts',(150.289855072332,-79.4541343313065,-37.4414487162201));
#17875=CARTESIAN_POINT('Ctrl Pts',(150.289855072464,-79.4541343310581,-37.5));
#17876=CARTESIAN_POINT('',(150.289855072464,-79.4541343310581,-44.5));
#17877=CARTESIAN_POINT('',(150.289855072464,-79.4541343310581,115.));
#17878=CARTESIAN_POINT('',(145.36231884058,-88.1464478086873,-49.5));
#17879=CARTESIAN_POINT('Ctrl Pts',(150.289855072464,-79.4541343310581,-44.5));
#17880=CARTESIAN_POINT('Ctrl Pts',(150.289855068577,-79.4541343384106,-44.7563523801461));
#17881=CARTESIAN_POINT('Ctrl Pts',(150.270581238553,-79.4906188049207,-45.0053815220034));
#17882=CARTESIAN_POINT('Ctrl Pts',(150.23440031069,-79.5589401936918,-45.2480116426047));
#17883=CARTESIAN_POINT('Ctrl Pts',(150.233993766309,-79.5597078820386,-45.2507379384179));
#17884=CARTESIAN_POINT('Ctrl Pts',(150.2335850823,-79.5604795994257,-45.2534634549803));
#17885=CARTESIAN_POINT('Ctrl Pts',(150.233174261933,-79.5612553394204,-45.2561881931872));
#17886=CARTESIAN_POINT('Ctrl Pts',(150.211108362005,-79.6029217280976,-45.4025387770759));
#17887=CARTESIAN_POINT('Ctrl Pts',(150.183223768725,-79.6555340186023,-45.5439666089425));
#17888=CARTESIAN_POINT('Ctrl Pts',(150.1506572954,-79.7168744981717,-45.6800320781738));
#17889=CARTESIAN_POINT('Ctrl Pts',(150.129869982031,-79.7560283776325,-45.7668832247325));
#17890=CARTESIAN_POINT('Ctrl Pts',(150.107175698374,-79.7987372958143,-45.8515497663918));
#17891=CARTESIAN_POINT('Ctrl Pts',(150.082875014061,-79.8444151271613,-45.9339198071965));
#17892=CARTESIAN_POINT('Ctrl Pts',(150.081600916097,-79.8468100404567,-45.9382385127928));
#17893=CARTESIAN_POINT('Ctrl Pts',(150.080322360848,-79.8492131928944,-45.9425510499967));
#17894=CARTESIAN_POINT('Ctrl Pts',(150.079039391808,-79.8516244996445,-45.94685739874));
#17895=CARTESIAN_POINT('Ctrl Pts',(150.044542112121,-79.9164612343949,-46.0626492162668));
#17896=CARTESIAN_POINT('Ctrl Pts',(150.006537123161,-79.9877842271942,-46.1748654509807));
#17897=CARTESIAN_POINT('Ctrl Pts',(149.965970804575,-80.0637685565973,-46.2827346305569));
#17898=CARTESIAN_POINT('Ctrl Pts',(149.933351576217,-80.1248672778719,-46.3694718432009));
#17899=CARTESIAN_POINT('Ctrl Pts',(149.899077126141,-80.1889782570263,-46.4533984421142));
#17900=CARTESIAN_POINT('Ctrl Pts',(149.863649966461,-80.2551332464111,-46.5341227219249));
#17901=CARTESIAN_POINT('Ctrl Pts',(149.861515024356,-80.2591199355374,-46.5389873982183));
#17902=CARTESIAN_POINT('Ctrl Pts',(149.85937578758,-80.2631142503699,-46.5438407130638));
#17903=CARTESIAN_POINT('Ctrl Pts',(149.857232364154,-80.2671159825673,-46.5486825816028));
#17904=CARTESIAN_POINT('Ctrl Pts',(149.804252858279,-80.3660277477057,-46.6683601962307));
#17905=CARTESIAN_POINT('Ctrl Pts',(149.748484158479,-80.4699094430547,-46.7819066280769));
#17906=CARTESIAN_POINT('Ctrl Pts',(149.690355247898,-80.5778965450365,-46.8902500251402));
#17907=CARTESIAN_POINT('Ctrl Pts',(149.661473306408,-80.6315510369212,-46.9440815458665));
#17908=CARTESIAN_POINT('Ctrl Pts',(149.632008986731,-80.6862185045812,-46.9966292711324));
#17909=CARTESIAN_POINT('Ctrl Pts',(149.60201639041,-80.741790230842,-47.0480105076949));
#17910=CARTESIAN_POINT('Ctrl Pts',(149.599223408299,-80.7469652025476,-47.0527952510041));
#17911=CARTESIAN_POINT('Ctrl Pts',(149.596425806469,-80.7521480873936,-47.0575699305601));
#17912=CARTESIAN_POINT('Ctrl Pts',(149.593623625112,-80.7573388040449,-47.0623346471253));
#17913=CARTESIAN_POINT('Ctrl Pts',(149.503321107799,-80.9246137661054,-47.2158814184506));
#17914=CARTESIAN_POINT('Ctrl Pts',(149.407759531995,-81.1009468141059,-47.3595995786781));
#17915=CARTESIAN_POINT('Ctrl Pts',(149.309404815745,-81.2816192446479,-47.4931449450858));
#17916=CARTESIAN_POINT('Ctrl Pts',(149.306147321137,-81.2876030905749,-47.4975679491626));
#17917=CARTESIAN_POINT('Ctrl Pts',(149.302886794892,-81.2935916372183,-47.501979751875));
#17918=CARTESIAN_POINT('Ctrl Pts',(149.299623326396,-81.2995847135535,-47.5063803428043));
#17919=CARTESIAN_POINT('Ctrl Pts',(149.201294060241,-81.4801578671638,-47.6389714425028));
#17920=CARTESIAN_POINT('Ctrl Pts',(149.100390942177,-81.6646756184357,-47.7614147349028));
#17921=CARTESIAN_POINT('Ctrl Pts',(148.997297013874,-81.8523394986245,-47.8757113225169));
#17922=CARTESIAN_POINT('Ctrl Pts',(148.993783486671,-81.8587352404397,-47.8796066457086));
#17923=CARTESIAN_POINT('Ctrl Pts',(148.99026742009,-81.8651346268366,-47.8834924864782));
#17924=CARTESIAN_POINT('Ctrl Pts',(148.986748829868,-81.871537625153,-47.8873689234621));
#17925=CARTESIAN_POINT('Ctrl Pts',(148.828989572841,-82.1586219951734,-48.0611725720732));
#17926=CARTESIAN_POINT('Ctrl Pts',(148.666197518726,-82.4528887104789,-48.2162655070009));
#17927=CARTESIAN_POINT('Ctrl Pts',(148.499047675041,-82.7528397905676,-48.3561560144813));
#17928=CARTESIAN_POINT('Ctrl Pts',(148.443888606593,-82.851822965143,-48.4023195639484));
#17929=CARTESIAN_POINT('Ctrl Pts',(148.388255039765,-82.9514250577883,-48.4468280100297));
#17930=CARTESIAN_POINT('Ctrl Pts',(148.332171389768,-83.0515919680528,-48.4898085924912));
#17931=CARTESIAN_POINT('Ctrl Pts',(148.328463625565,-83.0582141348388,-48.4926500955871));
#17932=CARTESIAN_POINT('Ctrl Pts',(148.324753888106,-83.0648387811285,-48.4954849142925));
#17933=CARTESIAN_POINT('Ctrl Pts',(148.321042184227,-83.0714658916725,-48.4983130852896));
#17934=CARTESIAN_POINT('Ctrl Pts',(148.127526079489,-83.4169817679216,-48.6457646742983));
#17935=CARTESIAN_POINT('Ctrl Pts',(147.928023779063,-83.7703038873281,-48.7751050652708));
#17936=CARTESIAN_POINT('Ctrl Pts',(147.726117191241,-84.1248695147338,-48.8871259760477));
#17937=CARTESIAN_POINT('Ctrl Pts',(147.691851026851,-84.1850438963965,-48.9061373762463));
#17938=CARTESIAN_POINT('Ctrl Pts',(147.657515670427,-84.2452539899323,-48.9246499566981));
#17939=CARTESIAN_POINT('Ctrl Pts',(147.623128700903,-84.3054675885421,-48.9426676169133));
#17940=CARTESIAN_POINT('Ctrl Pts',(147.61966084937,-84.3115399997817,-48.9444846589923));
#17941=CARTESIAN_POINT('Ctrl Pts',(147.616192453019,-84.3176124815105,-48.9462966777585));
#17942=CARTESIAN_POINT('Ctrl Pts',(147.612723530195,-84.3236850001122,-48.9481036768601));
#17943=CARTESIAN_POINT('Ctrl Pts',(147.41439805748,-84.6708634135425,-49.0514135425518));
#17944=CARTESIAN_POINT('Ctrl Pts',(147.213653682834,-85.0194306321946,-49.1388789349076));
#17945=CARTESIAN_POINT('Ctrl Pts',(147.010609976465,-85.3690841855301,-49.211977417735));
#17946=CARTESIAN_POINT('Ctrl Pts',(146.970506380402,-85.4381450055664,-49.2264152551867));
#17947=CARTESIAN_POINT('Ctrl Pts',(146.930313102763,-85.5072481940793,-49.2402927866165));
#17948=CARTESIAN_POINT('Ctrl Pts',(146.89003109062,-85.5763914060563,-49.253621628096));
#17949=CARTESIAN_POINT('Ctrl Pts',(146.887290932544,-85.5810948287668,-49.254528314001));
#17950=CARTESIAN_POINT('Ctrl Pts',(146.884550362083,-85.5857984397406,-49.2554324609279));
#17951=CARTESIAN_POINT('Ctrl Pts',(146.881809379355,-85.5905022385503,-49.2563340725845));
#17952=CARTESIAN_POINT('Ctrl Pts',(146.534412670951,-86.18666952076,-49.3706058330548));
#17953=CARTESIAN_POINT('Ctrl Pts',(146.180413916078,-86.7858240349752,-49.4448187829498));
#17954=CARTESIAN_POINT('Ctrl Pts',(145.819603406779,-87.3878896744197,-49.4786922813549));
#17955=CARTESIAN_POINT('Ctrl Pts',(145.668377265966,-87.6402328319036,-49.4928896461978));
#17956=CARTESIAN_POINT('Ctrl Pts',(145.515954394526,-87.8930873961788,-49.4999999997319));
#17957=CARTESIAN_POINT('Ctrl Pts',(145.36231884058,-88.1464478086873,-49.5));
#17958=CARTESIAN_POINT('Origin',(0.,0.,-49.5));
#17959=CARTESIAN_POINT('',(114.505594583524,-125.652173913043,-87.5));
#17960=CARTESIAN_POINT('Ctrl Pts',(114.505594583524,-125.652173913043,-87.5));
#17961=CARTESIAN_POINT('Ctrl Pts',(114.875320875519,-125.315245966795,-87.4999999999648));
#17962=CARTESIAN_POINT('Ctrl Pts',(115.240344836351,-124.979614106079,-87.4659613711684));
#17963=CARTESIAN_POINT('Ctrl Pts',(115.600645995236,-124.645458529299,-87.3949999533009));
#17964=CARTESIAN_POINT('Ctrl Pts',(115.815592867061,-124.44610947321,-87.3526661044782));
#17965=CARTESIAN_POINT('Ctrl Pts',(116.028858889205,-124.247285601145,-87.2971925568625));
#17966=CARTESIAN_POINT('Ctrl Pts',(116.240439697972,-124.049023288465,-87.2279752537402));
#17967=CARTESIAN_POINT('Ctrl Pts',(116.245828883255,-124.043973339257,-87.2262122163766));
#17968=CARTESIAN_POINT('Ctrl Pts',(116.251215926061,-124.038924730883,-87.2244403150212));
#17969=CARTESIAN_POINT('Ctrl Pts',(116.25660079453,-124.033877495354,-87.2226595463956));
#17970=CARTESIAN_POINT('Ctrl Pts',(116.416321748786,-123.884171095005,-87.1698400456397));
#17971=CARTESIAN_POINT('Ctrl Pts',(116.574127437902,-123.735675042354,-87.1092235237401));
#17972=CARTESIAN_POINT('Ctrl Pts',(116.729307011656,-123.58910958441,-87.0406588494489));
#17973=CARTESIAN_POINT('Ctrl Pts',(116.845631220437,-123.479242605673,-86.9892620625242));
#17974=CARTESIAN_POINT('Ctrl Pts',(116.960479920625,-123.37046021929,-86.9333980876332));
#17975=CARTESIAN_POINT('Ctrl Pts',(117.073550031386,-123.263067798316,-86.8729844025496));
#17976=CARTESIAN_POINT('Ctrl Pts',(117.079344844514,-123.257563965281,-86.8698882172442));
#17977=CARTESIAN_POINT('Ctrl Pts',(117.085135613102,-123.252063194138,-86.866779947454));
#17978=CARTESIAN_POINT('Ctrl Pts',(117.090922329314,-123.24656549557,-86.8636595351634));
#17979=CARTESIAN_POINT('Ctrl Pts',(117.252833947858,-123.09274055571,-86.7763507773278));
#17980=CARTESIAN_POINT('Ctrl Pts',(117.411527264105,-122.941364416115,-86.6795632238425));
#17981=CARTESIAN_POINT('Ctrl Pts',(117.566613453642,-122.792879292936,-86.5721870844575));
#17982=CARTESIAN_POINT('Ctrl Pts',(117.663683594909,-122.699940831258,-86.5049791850956));
#17983=CARTESIAN_POINT('Ctrl Pts',(117.759340859083,-122.608134753005,-86.4336238696905));
#17984=CARTESIAN_POINT('Ctrl Pts',(117.853493006743,-122.517566847009,-86.3578587588989));
#17985=CARTESIAN_POINT('Ctrl Pts',(117.859134880481,-122.512139751579,-86.3533186905155));
#17986=CARTESIAN_POINT('Ctrl Pts',(117.864772463519,-122.506716022107,-86.3487614273767));
#17987=CARTESIAN_POINT('Ctrl Pts',(117.870405487109,-122.50129592327,-86.3441871089973));
#17988=CARTESIAN_POINT('Ctrl Pts',(117.971986956638,-122.403554169479,-86.2616974876356));
#17989=CARTESIAN_POINT('Ctrl Pts',(118.072186599589,-122.30689585151,-86.1735699087614));
#17990=CARTESIAN_POINT('Ctrl Pts',(118.169344470473,-122.212953361586,-86.0806804467523));
#17991=CARTESIAN_POINT('Ctrl Pts',(118.186308138285,-122.196551096098,-86.064462038893));
#17992=CARTESIAN_POINT('Ctrl Pts',(118.203179139124,-122.180231567867,-86.0480985649969));
#17993=CARTESIAN_POINT('Ctrl Pts',(118.219948731942,-122.164003379953,-86.031594805261));
#17994=CARTESIAN_POINT('Ctrl Pts',(118.225239204071,-122.158883710274,-86.0263881981678));
#17995=CARTESIAN_POINT('Ctrl Pts',(118.2305200644,-122.153772676115,-86.0211674735436));
#17996=CARTESIAN_POINT('Ctrl Pts',(118.235791265575,-122.148670330441,-86.0159325934032));
#17997=CARTESIAN_POINT('Ctrl Pts',(118.348386205055,-122.039682211169,-85.9041134855647));
#17998=CARTESIAN_POINT('Ctrl Pts',(118.456626331103,-121.93460772812,-85.7857889099975));
#17999=CARTESIAN_POINT('Ctrl Pts',(118.560193282322,-121.833823583021,-85.6604137446068));
#18000=CARTESIAN_POINT('Ctrl Pts',(118.564867100718,-121.829275348417,-85.6547557547995));
#18001=CARTESIAN_POINT('Ctrl Pts',(118.569531415015,-121.824735838064,-85.649083428181));
#18002=CARTESIAN_POINT('Ctrl Pts',(118.57418617698,-121.820205105343,-85.6433966843365));
#18003=CARTESIAN_POINT('Ctrl Pts',(118.656113089351,-121.740461190303,-85.5433062032005));
#18004=CARTESIAN_POINT('Ctrl Pts',(118.73510902298,-121.663408950085,-85.4387098917068));
#18005=CARTESIAN_POINT('Ctrl Pts',(118.810850743183,-121.589398131891,-85.3292725022762));
#18006=CARTESIAN_POINT('Ctrl Pts',(118.830778159304,-121.569926110822,-85.3004798581098));
#18007=CARTESIAN_POINT('Ctrl Pts',(118.850480457642,-121.55066448544,-85.2713523136894));
#18008=CARTESIAN_POINT('Ctrl Pts',(118.869952060987,-121.531619330202,-85.2418842081897));
#18009=CARTESIAN_POINT('Ctrl Pts',(118.873852582751,-121.527804233869,-85.2359812024218));
#18010=CARTESIAN_POINT('Ctrl Pts',(118.87774476105,-121.523996924348,-85.2300626384257));
#18011=CARTESIAN_POINT('Ctrl Pts',(118.881628379448,-121.520197619565,-85.2241287426541));
#18012=CARTESIAN_POINT('Ctrl Pts',(118.95393335679,-121.449462388123,-85.1136518225858));
#18013=CARTESIAN_POINT('Ctrl Pts',(119.02337219024,-121.381403002896,-84.997686167018));
#18014=CARTESIAN_POINT('Ctrl Pts',(119.088533293332,-121.317439625781,-84.8776565982198));
#18015=CARTESIAN_POINT('Ctrl Pts',(119.107675671506,-121.298649103585,-84.8423955101026));
#18016=CARTESIAN_POINT('Ctrl Pts',(119.126449081002,-121.280211875349,-84.806783878756));
#18017=CARTESIAN_POINT('Ctrl Pts',(119.144818331366,-121.262163368406,-84.7708581772728));
#18018=CARTESIAN_POINT('Ctrl Pts',(119.147770180269,-121.259263061406,-84.7650850923405));
#18019=CARTESIAN_POINT('Ctrl Pts',(119.150711776641,-121.256372617005,-84.7593040201353));
#18020=CARTESIAN_POINT('Ctrl Pts',(119.153643085904,-121.253492073365,-84.7535149461629));
#18021=CARTESIAN_POINT('Ctrl Pts',(119.21747721143,-121.190763453579,-84.6274482498757));
#18022=CARTESIAN_POINT('Ctrl Pts',(119.276475877687,-121.132687812744,-84.4974947071808));
#18023=CARTESIAN_POINT('Ctrl Pts',(119.3302916925,-121.079649407404,-84.3634783755698));
#18024=CARTESIAN_POINT('Ctrl Pts',(119.344664771979,-121.065483957748,-84.3276854141062));
#18025=CARTESIAN_POINT('Ctrl Pts',(119.358668331281,-121.05167764448,-84.2916027835657));
#18026=CARTESIAN_POINT('Ctrl Pts',(119.37229615525,-121.038237390605,-84.2552274353945));
#18027=CARTESIAN_POINT('Ctrl Pts',(119.374201887271,-121.036357888622,-84.2501406610181));
#18028=CARTESIAN_POINT('Ctrl Pts',(119.376100550482,-121.034485269244,-84.2450470253995));
#18029=CARTESIAN_POINT('Ctrl Pts',(119.377992089409,-121.032619589192,-84.2399466200188));
#18030=CARTESIAN_POINT('Ctrl Pts',(119.432704267991,-120.978655370581,-84.0924189714974));
#18031=CARTESIAN_POINT('Ctrl Pts',(119.481511542453,-120.930442075976,-83.9390510932668));
#18032=CARTESIAN_POINT('Ctrl Pts',(119.523061427335,-120.889361770021,-83.7819751614011));
#18033=CARTESIAN_POINT('Ctrl Pts',(119.530667692994,-120.881841467105,-83.7532202979454));
#18034=CARTESIAN_POINT('Ctrl Pts',(119.538030846415,-120.874560108481,-83.7243411856429));
#18035=CARTESIAN_POINT('Ctrl Pts',(119.545142732111,-120.867526032261,-83.6953509136308));
#18036=CARTESIAN_POINT('Ctrl Pts',(119.546090881023,-120.866588256825,-83.6914859619103));
#18037=CARTESIAN_POINT('Ctrl Pts',(119.547034430282,-120.865655009876,-83.6876198631647));
#18038=CARTESIAN_POINT('Ctrl Pts',(119.547973377994,-120.864726293782,-83.6837526181087));
#18039=CARTESIAN_POINT('Ctrl Pts',(119.593937460371,-120.819263077397,-83.4944402974946));
#18040=CARTESIAN_POINT('Ctrl Pts',(119.62890424618,-120.784628102355,-83.3022686788512));
#18041=CARTESIAN_POINT('Ctrl Pts',(119.65264519197,-120.761105073466,-83.1071682749086));
#18042=CARTESIAN_POINT('Ctrl Pts',(119.676892336666,-120.737080492046,-82.9079079856867));
#18043=CARTESIAN_POINT('Ctrl Pts',(119.689439200918,-120.724637683323,-82.7055895150371));
#18044=CARTESIAN_POINT('Ctrl Pts',(119.689439203101,-120.724637681159,-82.5));
#18045=CARTESIAN_POINT('',(102.653719754201,-135.507246376812,-87.5));
#18046=CARTESIAN_POINT('Origin',(0.,0.,-87.5));
#18047=CARTESIAN_POINT('',(95.8022538025509,-140.434782608696,-82.5));
#18048=CARTESIAN_POINT('Ctrl Pts',(102.653719754201,-135.507246376812,-87.5));
#18049=CARTESIAN_POINT('Ctrl Pts',(102.215883490062,-135.838929901929,-87.4999999991685));
#18050=CARTESIAN_POINT('Ctrl Pts',(101.781087350657,-136.164971110003,-87.4669218367414));
#18051=CARTESIAN_POINT('Ctrl Pts',(101.349415497286,-136.485515662914,-87.4008783684644));
#18052=CARTESIAN_POINT('Ctrl Pts',(101.07973591123,-136.68577037414,-87.3596188444822));
#18053=CARTESIAN_POINT('Ctrl Pts',(100.811275778686,-136.88387961001,-87.3054922341186));
#18054=CARTESIAN_POINT('Ctrl Pts',(100.544056427545,-137.079877141377,-87.2385159157322));
#18055=CARTESIAN_POINT('Ctrl Pts',(100.541162556084,-137.081999710944,-87.2377905908054));
#18056=CARTESIAN_POINT('Ctrl Pts',(100.538268831608,-137.084122031661,-87.2370637322218));
#18057=CARTESIAN_POINT('Ctrl Pts',(100.535375254373,-137.086244103409,-87.2363353381554));
#18058=CARTESIAN_POINT('Ctrl Pts',(100.190565643195,-137.339118201716,-87.1495371453096));
#18059=CARTESIAN_POINT('Ctrl Pts',(99.8478512789412,-137.588453369916,-87.040933511602));
#18060=CARTESIAN_POINT('Ctrl Pts',(99.5077977395583,-137.833951510589,-86.9074976668159));
#18061=CARTESIAN_POINT('Ctrl Pts',(99.5037755731161,-137.836855272111,-86.9059193824726));
#18062=CARTESIAN_POINT('Ctrl Pts',(99.4997536170413,-137.839758608548,-86.9043375053786));
#18063=CARTESIAN_POINT('Ctrl Pts',(99.4957318889749,-137.842661507683,-86.9027520347699));
#18064=CARTESIAN_POINT('Ctrl Pts',(99.2674376143156,-138.007445213001,-86.8127524483652));
#18065=CARTESIAN_POINT('Ctrl Pts',(99.0398204570979,-138.170861151964,-86.711145683115));
#18066=CARTESIAN_POINT('Ctrl Pts',(98.8161737755042,-138.33062666086,-86.597820472154));
#18067=CARTESIAN_POINT('Ctrl Pts',(98.7076262937751,-138.408169254089,-86.5428177948124));
#18068=CARTESIAN_POINT('Ctrl Pts',(98.600013904115,-138.484852125992,-86.4850552618045));
#18069=CARTESIAN_POINT('Ctrl Pts',(98.4937108917853,-138.56041611792,-86.4245237415767));
#18070=CARTESIAN_POINT('Ctrl Pts',(98.4889708281906,-138.563785525046,-86.4218246341001));
#18071=CARTESIAN_POINT('Ctrl Pts',(98.4842329483831,-138.56715301161,-86.419119965262));
#18072=CARTESIAN_POINT('Ctrl Pts',(98.479497264693,-138.570518570128,-86.4164097092555));
#18073=CARTESIAN_POINT('Ctrl Pts',(98.2490703748719,-138.73427849005,-86.2845352212039));
#18074=CARTESIAN_POINT('Ctrl Pts',(98.0238750005084,-138.8934512373,-86.1394754931963));
#18075=CARTESIAN_POINT('Ctrl Pts',(97.8050966305876,-139.047339894881,-85.9780962529129));
#18076=CARTESIAN_POINT('Ctrl Pts',(97.7156206980972,-139.110277246236,-85.9120954045925));
#18077=CARTESIAN_POINT('Ctrl Pts',(97.6272183327067,-139.172330541299,-85.8433644738521));
#18078=CARTESIAN_POINT('Ctrl Pts',(97.5399718160535,-139.233451074562,-85.7716868356771));
#18079=CARTESIAN_POINT('Ctrl Pts',(97.5352562713784,-139.236754548629,-85.7678127657659));
#18080=CARTESIAN_POINT('Ctrl Pts',(97.5305452293931,-139.240054504138,-85.7639310032341));
#18081=CARTESIAN_POINT('Ctrl Pts',(97.5258387376046,-139.243350910624,-85.7600415156019));
#18082=CARTESIAN_POINT('Ctrl Pts',(97.3552183240805,-139.362852710079,-85.6190392536152));
#18083=CARTESIAN_POINT('Ctrl Pts',(97.1907405919816,-139.47757645948,-85.4680354210839));
#18084=CARTESIAN_POINT('Ctrl Pts',(97.0346910654179,-139.586057153202,-85.3056163231383));
#18085=CARTESIAN_POINT('Ctrl Pts',(96.9159928871056,-139.668572371353,-85.1820731668481));
#18086=CARTESIAN_POINT('Ctrl Pts',(96.8021704778946,-139.747475893107,-85.0519259141839));
#18087=CARTESIAN_POINT('Ctrl Pts',(96.694215926304,-139.822132033515,-84.9145642707921));
#18088=CARTESIAN_POINT('Ctrl Pts',(96.6906380099125,-139.824606347239,-84.9100117209624));
#18089=CARTESIAN_POINT('Ctrl Pts',(96.6870657587802,-139.827076536154,-84.9054498746293));
#18090=CARTESIAN_POINT('Ctrl Pts',(96.6834992847061,-139.82954252561,-84.9008787661799));
#18091=CARTESIAN_POINT('Ctrl Pts',(96.5933790288425,-139.891854937294,-84.7853726796454));
#18092=CARTESIAN_POINT('Ctrl Pts',(96.5068951547278,-139.951522102754,-84.6638795752373));
#18093=CARTESIAN_POINT('Ctrl Pts',(96.4259038292281,-140.007303114121,-84.5370163776214));
#18094=CARTESIAN_POINT('Ctrl Pts',(96.3961160047755,-140.027818829404,-84.4903573232502));
#18095=CARTESIAN_POINT('Ctrl Pts',(96.3670708290736,-140.047809094726,-84.4429721152884));
#18096=CARTESIAN_POINT('Ctrl Pts',(96.3388592767016,-140.067213127358,-84.3948922769621));
#18097=CARTESIAN_POINT('Ctrl Pts',(96.3362565453866,-140.069003297665,-84.390456544423));
#18098=CARTESIAN_POINT('Ctrl Pts',(96.3336613068006,-140.070788207782,-84.3860158118469));
#18099=CARTESIAN_POINT('Ctrl Pts',(96.3310735989047,-140.072567833443,-84.3815700581723));
#18100=CARTESIAN_POINT('Ctrl Pts',(96.2565223686416,-140.123838412584,-84.2534889844106));
#18101=CARTESIAN_POINT('Ctrl Pts',(96.18818677241,-140.170746863762,-84.1211671345774));
#18102=CARTESIAN_POINT('Ctrl Pts',(96.126962800212,-140.212720695597,-83.9840977199587));
#18103=CARTESIAN_POINT('Ctrl Pts',(96.1019843048262,-140.229845412064,-83.9281753807562));
#18104=CARTESIAN_POINT('Ctrl Pts',(96.0781891189942,-140.246149048065,-83.8714630194104));
#18105=CARTESIAN_POINT('Ctrl Pts',(96.0556361395659,-140.261594051371,-83.8139272219729));
#18106=CARTESIAN_POINT('Ctrl Pts',(96.0542034790336,-140.262575183231,-83.8102723050498));
#18107=CARTESIAN_POINT('Ctrl Pts',(96.0527757857576,-140.263552881361,-83.8066133446794));
#18108=CARTESIAN_POINT('Ctrl Pts',(96.0513530943973,-140.264527122689,-83.802950400001));
#18109=CARTESIAN_POINT('Ctrl Pts',(95.9866237488953,-140.308852972491,-83.6362944279056));
#18110=CARTESIAN_POINT('Ctrl Pts',(95.9322125151014,-140.346047836819,-83.4612414093815));
#18111=CARTESIAN_POINT('Ctrl Pts',(95.8913844101215,-140.373937837985,-83.2831693720156));
#18112=CARTESIAN_POINT('Ctrl Pts',(95.883045620544,-140.379634131044,-83.2467996886822));
#18113=CARTESIAN_POINT('Ctrl Pts',(95.8752733682718,-140.384942326837,-83.2103039208797));
#18114=CARTESIAN_POINT('Ctrl Pts',(95.8680953540231,-140.38984398165,-83.1737276630787));
#18115=CARTESIAN_POINT('Ctrl Pts',(95.8676809810245,-140.390126944783,-83.1716161858517));
#18116=CARTESIAN_POINT('Ctrl Pts',(95.8672684958815,-140.390408616667,-83.1695042863138));
#18117=CARTESIAN_POINT('Ctrl Pts',(95.8668579005401,-140.390688996011,-83.1673919642828));
#18118=CARTESIAN_POINT('Ctrl Pts',(95.8468264218082,-140.404367701805,-83.0643393244232));
#18119=CARTESIAN_POINT('Ctrl Pts',(95.8312774654238,-140.414980545424,-82.9601876791363));
#18120=CARTESIAN_POINT('Ctrl Pts',(95.8204649814164,-140.422358778653,-82.855032721006));
#18121=CARTESIAN_POINT('Ctrl Pts',(95.8099639220234,-140.429524501655,-82.7529064695304));
#18122=CARTESIAN_POINT('Ctrl Pts',(95.8039305392802,-140.433639185389,-82.649833883227));
#18123=CARTESIAN_POINT('Ctrl Pts',(95.8025570944415,-140.434575788992,-82.5459117712175));
#18124=CARTESIAN_POINT('Ctrl Pts',(95.802355077537,-140.434713551904,-82.5306261020837));
#18125=CARTESIAN_POINT('Ctrl Pts',(95.8022538025544,-140.434782608693,-82.5153220699784));
#18126=CARTESIAN_POINT('Ctrl Pts',(95.8022538025544,-140.434782608693,-82.5));
#18127=CARTESIAN_POINT('',(95.8022538025509,-140.434782608696,82.5));
#18128=CARTESIAN_POINT('',(95.802253802551,-140.434782608696,115.));
#18129=CARTESIAN_POINT('',(102.653719754201,-135.507246376812,87.5));
#18130=CARTESIAN_POINT('Ctrl Pts',(95.8022538025509,-140.434782608696,82.5));
#18131=CARTESIAN_POINT('Ctrl Pts',(95.8022538066581,-140.434782605894,82.7267635628216));
#18132=CARTESIAN_POINT('Ctrl Pts',(95.82442316008,-140.419665963906,82.9488530674831));
#18133=CARTESIAN_POINT('Ctrl Pts',(95.8667225776694,-140.39078140277,83.1666939397165));
#18134=CARTESIAN_POINT('Ctrl Pts',(95.8671957348732,-140.390458302857,83.1691306866946));
#18135=CARTESIAN_POINT('Ctrl Pts',(95.8676714126208,-140.390133479021,83.1715669081132));
#18136=CARTESIAN_POINT('Ctrl Pts',(95.8681496080969,-140.389806933124,83.1740026044675));
#18137=CARTESIAN_POINT('Ctrl Pts',(95.9022176054037,-140.366542880454,83.3475284970882));
#18138=CARTESIAN_POINT('Ctrl Pts',(95.9496913058969,-140.334107437353,83.5193033103427));
#18139=CARTESIAN_POINT('Ctrl Pts',(96.0075075764076,-140.294541978645,83.6842311536385));
#18140=CARTESIAN_POINT('Ctrl Pts',(96.0214298424345,-140.28501454222,83.7239460866381));
#18141=CARTESIAN_POINT('Ctrl Pts',(96.0359516723965,-140.275073772703,83.7632638427573));
#18142=CARTESIAN_POINT('Ctrl Pts',(96.0510300136253,-140.264748363786,83.8021130045776));
#18143=CARTESIAN_POINT('Ctrl Pts',(96.0526816582041,-140.263617343775,83.8063684466409));
#18144=CARTESIAN_POINT('Ctrl Pts',(96.0543400150297,-140.262481684736,83.8106183997866));
#18145=CARTESIAN_POINT('Ctrl Pts',(96.0560050279566,-140.261341424076,83.8148627669174));
#18146=CARTESIAN_POINT('Ctrl Pts',(96.1087379306462,-140.22522803811,83.9492868276993));
#18147=CARTESIAN_POINT('Ctrl Pts',(96.1682453864418,-140.18443183692,84.0791983701197));
#18148=CARTESIAN_POINT('Ctrl Pts',(96.233756492817,-140.139445304686,84.2050184596988));
#18149=CARTESIAN_POINT('Ctrl Pts',(96.2645815930226,-140.118277682267,84.2642208924426));
#18150=CARTESIAN_POINT('Ctrl Pts',(96.2967352970668,-140.096182731474,84.322517794146));
#18151=CARTESIAN_POINT('Ctrl Pts',(96.3301343379528,-140.073213779952,84.379954552556));
#18152=CARTESIAN_POINT('Ctrl Pts',(96.333181322976,-140.071118329022,84.3851944917284));
#18153=CARTESIAN_POINT('Ctrl Pts',(96.3362387534725,-140.069015548404,84.3904274269311));
#18154=CARTESIAN_POINT('Ctrl Pts',(96.339306565948,-140.066905478751,84.395653391359));
#18155=CARTESIAN_POINT('Ctrl Pts',(96.4117861971904,-140.017053321377,84.5191211644543));
#18156=CARTESIAN_POINT('Ctrl Pts',(96.489984201705,-139.963182743649,84.6383213999031));
#18157=CARTESIAN_POINT('Ctrl Pts',(96.5721307821755,-139.906480636874,84.7523713006202));
#18158=CARTESIAN_POINT('Ctrl Pts',(96.6081754745549,-139.881600599455,84.8024146933422));
#18159=CARTESIAN_POINT('Ctrl Pts',(96.6449798263787,-139.856175797165,84.8514667731971));
#18160=CARTESIAN_POINT('Ctrl Pts',(96.6823922460869,-139.830307960496,84.8994546030534));
#18161=CARTESIAN_POINT('Ctrl Pts',(96.6866911658705,-139.827335585127,84.9049687032572));
#18162=CARTESIAN_POINT('Ctrl Pts',(96.6909982721174,-139.824357251048,84.910468962333));
#18163=CARTESIAN_POINT('Ctrl Pts',(96.6953133447454,-139.821373105703,84.9159552790206));
#18164=CARTESIAN_POINT('Ctrl Pts',(96.8598715711489,-139.707570695464,85.1251796933976));
#18165=CARTESIAN_POINT('Ctrl Pts',(97.0374177648447,-139.584350177983,85.3170893285477));
#18166=CARTESIAN_POINT('Ctrl Pts',(97.2253643458243,-139.453317347345,85.4947229628092));
#18167=CARTESIAN_POINT('Ctrl Pts',(97.3220405832959,-139.385916488094,85.5860944116501));
#18168=CARTESIAN_POINT('Ctrl Pts',(97.4214682311097,-139.316448807693,85.6736891876995));
#18169=CARTESIAN_POINT('Ctrl Pts',(97.5232920470747,-139.245134572953,85.7579251167103));
#18170=CARTESIAN_POINT('Ctrl Pts',(97.5293253469238,-139.24090903733,85.7629162930178));
#18171=CARTESIAN_POINT('Ctrl Pts',(97.5353667088665,-139.236677264114,85.7678953452721));
#18172=CARTESIAN_POINT('Ctrl Pts',(97.5414160595531,-139.232439298912,85.7728623680769));
#18173=CARTESIAN_POINT('Ctrl Pts',(97.7162996211817,-139.10992194342,85.9164563972194));
#18174=CARTESIAN_POINT('Ctrl Pts',(97.8952913851829,-138.984032327629,86.0478104714154));
#18175=CARTESIAN_POINT('Ctrl Pts',(98.0778068948705,-138.855116179527,86.1688889205228));
#18176=CARTESIAN_POINT('Ctrl Pts',(98.208102146782,-138.763084756986,86.255325120134));
#18177=CARTESIAN_POINT('Ctrl Pts',(98.3401938135588,-138.669510449023,86.3365230930489));
#18178=CARTESIAN_POINT('Ctrl Pts',(98.4738752709946,-138.57451383921,86.4131838583196));
#18179=CARTESIAN_POINT('Ctrl Pts',(98.4804799835179,-138.569820403707,86.4169713867184));
#18180=CARTESIAN_POINT('Ctrl Pts',(98.4870884834125,-138.565123562489,86.4207477533717));
#18181=CARTESIAN_POINT('Ctrl Pts',(98.4937007396701,-138.560423334432,86.424513039284));
#18182=CARTESIAN_POINT('Ctrl Pts',(98.7840182406829,-138.354055279349,86.589831556));
#18183=CARTESIAN_POINT('Ctrl Pts',(99.0816753157249,-138.141093442614,86.7335191053828));
#18184=CARTESIAN_POINT('Ctrl Pts',(99.3855316242237,-137.922137706692,86.8583876044078));
#18185=CARTESIAN_POINT('Ctrl Pts',(99.4178327967954,-137.898861813403,86.8716616382947));
#18186=CARTESIAN_POINT('Ctrl Pts',(99.4502040185954,-137.875518189568,86.8847230539631));
#18187=CARTESIAN_POINT('Ctrl Pts',(99.4826439161487,-137.852107558311,86.8975752625191));
#18188=CARTESIAN_POINT('Ctrl Pts',(99.4892006235699,-137.847375833759,86.9001729332139));
#18189=CARTESIAN_POINT('Ctrl Pts',(99.4957601913217,-137.842641332283,86.9027620700699));
#18190=CARTESIAN_POINT('Ctrl Pts',(99.5023226100944,-137.83790405835,86.9053427012608));
#18191=CARTESIAN_POINT('Ctrl Pts',(99.7610782414197,-137.651113737626,87.0070967764188));
#18192=CARTESIAN_POINT('Ctrl Pts',(100.023540548063,-137.460524429705,87.0951230469053));
#18193=CARTESIAN_POINT('Ctrl Pts',(100.286778082508,-137.268209583308,87.1698025078672));
#18194=CARTESIAN_POINT('Ctrl Pts',(100.367689287584,-137.209097853635,87.1927567009067));
#18195=CARTESIAN_POINT('Ctrl Pts',(100.448673514288,-137.149823232307,87.2144496896512));
#18196=CARTESIAN_POINT('Ctrl Pts',(100.529644945652,-137.09044635394,87.2348918842082));
#18197=CARTESIAN_POINT('Ctrl Pts',(100.535236887059,-137.086345746859,87.2363036358874));
#18198=CARTESIAN_POINT('Ctrl Pts',(100.54082877009,-137.082244650117,87.2377094234242));
#18199=CARTESIAN_POINT('Ctrl Pts',(100.546420565381,-137.078143084482,87.2391092498982));
#18200=CARTESIAN_POINT('Ctrl Pts',(101.006759430624,-136.740485861341,87.3543485419369));
#18201=CARTESIAN_POINT('Ctrl Pts',(101.469785371656,-136.397290219446,87.4312211195578));
#18202=CARTESIAN_POINT('Ctrl Pts',(101.935255321594,-136.048534052163,87.4701010401868));
#18203=CARTESIAN_POINT('Ctrl Pts',(102.174111254841,-135.869569803615,87.4900522738327));
#18204=CARTESIAN_POINT('Ctrl Pts',(102.41361062282,-135.689141412998,87.4999999996522));
#18205=CARTESIAN_POINT('Ctrl Pts',(102.653719754201,-135.507246376812,87.5));
#18206=CARTESIAN_POINT('',(114.505594583524,-125.652173913043,87.5));
#18207=CARTESIAN_POINT('Origin',(0.,0.,87.5));
#18208=CARTESIAN_POINT('Ctrl Pts',(119.689439203101,-120.724637681159,82.5));
#18209=CARTESIAN_POINT('Ctrl Pts',(119.689439202149,-120.724637682103,82.7035326184388));
#18210=CARTESIAN_POINT('Ctrl Pts',(119.677137855384,-120.736837058147,82.9047280297056));
#18211=CARTESIAN_POINT('Ctrl Pts',(119.653068783703,-120.760685368386,83.1036884565072));
#18212=CARTESIAN_POINT('Ctrl Pts',(119.653066214653,-120.760687913874,83.1037096928656));
#18213=CARTESIAN_POINT('Ctrl Pts',(119.653063645461,-120.7606904595,83.1037309292184));
#18214=CARTESIAN_POINT('Ctrl Pts',(119.65306107613,-120.760693005265,83.1037521655658));
#18215=CARTESIAN_POINT('Ctrl Pts',(119.641919852112,-120.771732040823,83.1958379462712));
#18216=CARTESIAN_POINT('Ctrl Pts',(119.628149514819,-120.785373482771,83.2877525623368));
#18217=CARTESIAN_POINT('Ctrl Pts',(119.611957511351,-120.801406080558,83.3788351082885));
#18218=CARTESIAN_POINT('Ctrl Pts',(119.594967539022,-120.818228791431,83.4744063535959));
#18219=CARTESIAN_POINT('Ctrl Pts',(119.575311134738,-120.837684355099,83.5690634426131));
#18220=CARTESIAN_POINT('Ctrl Pts',(119.553189137451,-120.859567147649,83.6620443511901));
#18221=CARTESIAN_POINT('Ctrl Pts',(119.550837400782,-120.861893455034,83.6719289293931));
#18222=CARTESIAN_POINT('Ctrl Pts',(119.548457766993,-120.864247225519,83.6817945489539));
#18223=CARTESIAN_POINT('Ctrl Pts',(119.546050454752,-120.866628234349,83.6916402803607));
#18224=CARTESIAN_POINT('Ctrl Pts',(119.545706019787,-120.866968905857,83.6930489942347));
#18225=CARTESIAN_POINT('Ctrl Pts',(119.545361019709,-120.867310133486,83.6944572963286));
#18226=CARTESIAN_POINT('Ctrl Pts',(119.545015455303,-120.867651916433,83.6958651833482));
#18227=CARTESIAN_POINT('Ctrl Pts',(119.498574793915,-120.913584384682,83.8850721826734));
#18228=CARTESIAN_POINT('Ctrl Pts',(119.442053836954,-120.969435426432,84.0677448259361));
#18229=CARTESIAN_POINT('Ctrl Pts',(119.376325844471,-121.034263033589,84.2444400249401));
#18230=CARTESIAN_POINT('Ctrl Pts',(119.375341514618,-121.035233879443,84.2470861784681));
#18231=CARTESIAN_POINT('Ctrl Pts',(119.374355124207,-121.036206734213,84.2497309822512));
#18232=CARTESIAN_POINT('Ctrl Pts',(119.373366676024,-121.037181594879,84.2523744389027));
#18233=CARTESIAN_POINT('Ctrl Pts',(119.316775771354,-121.09299458329,84.4037183393109));
#18234=CARTESIAN_POINT('Ctrl Pts',(119.253023740074,-121.155791267856,84.5514088442846));
#18235=CARTESIAN_POINT('Ctrl Pts',(119.183533814645,-121.224111670241,84.6934551431387));
#18236=CARTESIAN_POINT('Ctrl Pts',(119.172587065774,-121.234874184132,84.7158316984741));
#18237=CARTESIAN_POINT('Ctrl Pts',(119.161497891706,-121.24577380549,84.7380680951027));
#18238=CARTESIAN_POINT('Ctrl Pts',(119.150271823512,-121.256804856299,84.7601564357349));
#18239=CARTESIAN_POINT('Ctrl Pts',(119.148539861699,-121.258506730759,84.7635642328208));
#18240=CARTESIAN_POINT('Ctrl Pts',(119.146804666256,-121.260211709207,84.7669684593409));
#18241=CARTESIAN_POINT('Ctrl Pts',(119.14506625839,-121.261919769913,84.7703690853657));
#18242=CARTESIAN_POINT('Ctrl Pts',(119.003325684158,-121.401185997451,85.0476381285352));
#18243=CARTESIAN_POINT('Ctrl Pts',(118.842142582395,-121.559065373447,85.2991641768823));
#18244=CARTESIAN_POINT('Ctrl Pts',(118.664609105015,-121.732125921824,85.5295568165563));
#18245=CARTESIAN_POINT('Ctrl Pts',(118.63378202579,-121.76217631747,85.5695624102107));
#18246=CARTESIAN_POINT('Ctrl Pts',(118.602462004168,-121.79268438568,85.6089309118895));
#18247=CARTESIAN_POINT('Ctrl Pts',(118.570665287738,-121.823632077489,85.6476865935974));
#18248=CARTESIAN_POINT('Ctrl Pts',(118.567733597815,-121.826485486471,85.6512599072698));
#18249=CARTESIAN_POINT('Ctrl Pts',(118.564797840986,-121.829342646821,85.6548280160811));
#18250=CARTESIAN_POINT('Ctrl Pts',(118.561858031783,-121.832203542636,85.6583909367604));
#18251=CARTESIAN_POINT('Ctrl Pts',(118.462775019687,-121.928626866429,85.7784752308077));
#18252=CARTESIAN_POINT('Ctrl Pts',(118.358568310361,-122.029796769546,85.8929376116578));
#18253=CARTESIAN_POINT('Ctrl Pts',(118.251586147631,-122.133379333937,86.0001705914024));
#18254=CARTESIAN_POINT('Ctrl Pts',(118.244181404727,-122.140548774516,86.0075926945414));
#18255=CARTESIAN_POINT('Ctrl Pts',(118.236763378118,-122.147729761558,86.0149801740683));
#18256=CARTESIAN_POINT('Ctrl Pts',(118.229332851436,-122.154921516527,86.0223325018977));
#18257=CARTESIAN_POINT('Ctrl Pts',(118.226055490992,-122.158093562638,86.0255753714058));
#18258=CARTESIAN_POINT('Ctrl Pts',(118.222775639178,-122.161267761231,86.0288114700421));
#18259=CARTESIAN_POINT('Ctrl Pts',(118.219493362288,-122.164444046394,86.0320407520764));
#18260=CARTESIAN_POINT('Ctrl Pts',(118.104628229969,-122.27559993839,86.1450512994916));
#18261=CARTESIAN_POINT('Ctrl Pts',(117.986476048706,-122.389622505763,86.2501973510142));
#18262=CARTESIAN_POINT('Ctrl Pts',(117.865390836685,-122.506120837556,86.3482582753081));
#18263=CARTESIAN_POINT('Ctrl Pts',(117.861984025646,-122.509398593743,86.3510172830664));
#18264=CARTESIAN_POINT('Ctrl Pts',(117.858574879434,-122.512678322681,86.3537706967459));
#18265=CARTESIAN_POINT('Ctrl Pts',(117.855163404827,-122.515960016733,86.3565185352213));
#18266=CARTESIAN_POINT('Ctrl Pts',(117.634786727148,-122.727953044864,86.5340252101117));
#18267=CARTESIAN_POINT('Ctrl Pts',(117.404749933279,-122.948091220296,86.6884140414481));
#18268=CARTESIAN_POINT('Ctrl Pts',(117.165977820927,-123.175215090991,86.8223776639549));
#18269=CARTESIAN_POINT('Ctrl Pts',(117.138194024572,-123.201643484612,86.8379658244401));
#18270=CARTESIAN_POINT('Ctrl Pts',(117.11029196616,-123.228166449504,86.8532774834095));
#18271=CARTESIAN_POINT('Ctrl Pts',(117.082273113257,-123.25478214762,86.8683169246699));
#18272=CARTESIAN_POINT('Ctrl Pts',(117.07907454041,-123.257820539291,86.8700337954002));
#18273=CARTESIAN_POINT('Ctrl Pts',(117.075874453948,-123.260860131433,86.871747111702));
#18274=CARTESIAN_POINT('Ctrl Pts',(117.072672856275,-123.263900921107,86.8734568798933));
#18275=CARTESIAN_POINT('Ctrl Pts',(116.860769276682,-123.465161130014,86.9866210051082));
#18276=CARTESIAN_POINT('Ctrl Pts',(116.644679573649,-123.669347678144,87.082787673174));
#18277=CARTESIAN_POINT('Ctrl Pts',(116.426318407412,-123.874581811768,87.1633254409075));
#18278=CARTESIAN_POINT('Ctrl Pts',(116.366869225742,-123.930457137519,87.1852519787982));
#18279=CARTESIAN_POINT('Ctrl Pts',(116.307251761957,-123.986410050552,87.2060203754224));
#18280=CARTESIAN_POINT('Ctrl Pts',(116.247504799008,-124.042402536954,87.2256588635444));
#18281=CARTESIAN_POINT('Ctrl Pts',(116.245124621172,-124.044633145315,87.2264412145101));
#18282=CARTESIAN_POINT('Ctrl Pts',(116.242744233986,-124.046863820072,87.2272217734333));
#18283=CARTESIAN_POINT('Ctrl Pts',(116.24036363979,-124.049094558926,87.2280005421223));
#18284=CARTESIAN_POINT('Ctrl Pts',(115.8311772319,-124.432523208838,87.3618585356373));
#18285=CARTESIAN_POINT('Ctrl Pts',(115.413668084723,-124.819944300696,87.4448575139198));
#18286=CARTESIAN_POINT('Ctrl Pts',(114.988112172538,-125.210757502246,87.4801920397485));
#18287=CARTESIAN_POINT('Ctrl Pts',(114.828401703243,-125.357429086495,87.4934530321137));
#18288=CARTESIAN_POINT('Ctrl Pts',(114.667557757302,-125.504578460163,87.4999999998164));
#18289=CARTESIAN_POINT('Ctrl Pts',(114.505594583524,-125.652173913043,87.5));
#18290=CARTESIAN_POINT('',(145.36231884058,-88.1464478086873,49.5));
#18291=CARTESIAN_POINT('Origin',(0.,0.,49.5));
#18292=CARTESIAN_POINT('',(150.289855072464,-79.4541343310581,44.5));
#18293=CARTESIAN_POINT('Ctrl Pts',(145.36231884058,-88.1464478086873,49.5));
#18294=CARTESIAN_POINT('Ctrl Pts',(145.729245608051,-87.5413488274995,49.4999999993448));
#18295=CARTESIAN_POINT('Ctrl Pts',(146.089427497743,-86.938852139224,49.459451627546));
#18296=CARTESIAN_POINT('Ctrl Pts',(146.443059008834,-86.3390437438767,49.3785345234731));
#18297=CARTESIAN_POINT('Ctrl Pts',(146.591729818533,-86.0868773022461,49.3445160296351));
#18298=CARTESIAN_POINT('Ctrl Pts',(146.739242767663,-85.8351860376504,49.3033619016674));
#18299=CARTESIAN_POINT('Ctrl Pts',(146.885611849037,-85.5839764893769,49.2550827834563));
#18300=CARTESIAN_POINT('Ctrl Pts',(146.887215711036,-85.581223821639,49.2545537575016));
#18301=CARTESIAN_POINT('Ctrl Pts',(146.888819435246,-85.5784712124141,49.2540238618083));
#18302=CARTESIAN_POINT('Ctrl Pts',(146.890423021642,-85.5757186617924,49.2534930956204));
#18303=CARTESIAN_POINT('Ctrl Pts',(147.136163003217,-85.1539068149984,49.1721563659123));
#18304=CARTESIAN_POINT('Ctrl Pts',(147.378654044698,-84.733492627337,49.0703840441395));
#18305=CARTESIAN_POINT('Ctrl Pts',(147.617771548819,-84.3148475830954,48.9454703779811));
#18306=CARTESIAN_POINT('Ctrl Pts',(147.619992196193,-84.3109596911514,48.9443103240332));
#18307=CARTESIAN_POINT('Ctrl Pts',(147.622212556282,-84.307071941363,48.943148258573));
#18308=CARTESIAN_POINT('Ctrl Pts',(147.624432625828,-84.303184339794,48.9419841796181));
#18309=CARTESIAN_POINT('Ctrl Pts',(147.797445356911,-84.0002188016352,48.8512660849843));
#18310=CARTESIAN_POINT('Ctrl Pts',(147.968707326118,-83.6981287755317,48.7483109143164));
#18311=CARTESIAN_POINT('Ctrl Pts',(148.136615104019,-83.3998939012959,48.6322285684957));
#18312=CARTESIAN_POINT('Ctrl Pts',(148.200188500854,-83.2869759397415,48.5882773642776));
#18313=CARTESIAN_POINT('Ctrl Pts',(148.263281189795,-83.1746104678287,48.5424447848479));
#18314=CARTESIAN_POINT('Ctrl Pts',(148.325806750807,-83.0629583612551,48.4946842709289));
#18315=CARTESIAN_POINT('Ctrl Pts',(148.328437713,-83.0582602431345,48.4926745951353));
#18316=CARTESIAN_POINT('Ctrl Pts',(148.331067922545,-83.0535629380485,48.4906613522023));
#18317=CARTESIAN_POINT('Ctrl Pts',(148.333697371916,-83.0488664605796,48.4886445330394));
#18318=CARTESIAN_POINT('Ctrl Pts',(148.479392264376,-82.7886398186652,48.3768948053783));
#18319=CARTESIAN_POINT('Ctrl Pts',(148.622808981178,-82.5308543489962,48.2541267340886));
#18320=CARTESIAN_POINT('Ctrl Pts',(148.762663381336,-82.2779954776877,48.1187795814413));
#18321=CARTESIAN_POINT('Ctrl Pts',(148.840976563632,-82.1364040593145,48.0429902875284));
#18322=CARTESIAN_POINT('Ctrl Pts',(148.918172933796,-81.9963571587517,47.9632574413117));
#18323=CARTESIAN_POINT('Ctrl Pts',(148.994029023493,-81.8582880066048,47.8793133555439));
#18324=CARTESIAN_POINT('Ctrl Pts',(148.996712266487,-81.8534041128184,47.8763440174079));
#18325=CARTESIAN_POINT('Ctrl Pts',(148.999393672824,-81.8485229853453,47.8733697901463));
#18326=CARTESIAN_POINT('Ctrl Pts',(149.002073232327,-81.8436446453373,47.8703906395336));
#18327=CARTESIAN_POINT('Ctrl Pts',(149.107681065302,-81.6513776267181,47.7529752061311));
#18328=CARTESIAN_POINT('Ctrl Pts',(149.210443318177,-81.4633981454557,47.6279048759376));
#18329=CARTESIAN_POINT('Ctrl Pts',(149.309720948425,-81.2810297213993,47.4931045485117));
#18330=CARTESIAN_POINT('Ctrl Pts',(149.401996350024,-81.111524068145,47.3678119290385));
#18331=CARTESIAN_POINT('Ctrl Pts',(149.491261252891,-80.9468661107977,47.2341131033335));
#18332=CARTESIAN_POINT('Ctrl Pts',(149.577013895448,-80.7880986852943,47.0903818425147));
#18333=CARTESIAN_POINT('Ctrl Pts',(149.583521150904,-80.7760507744081,47.0794749362875));
#18334=CARTESIAN_POINT('Ctrl Pts',(149.590008187584,-80.7640367723622,47.0685102812695));
#18335=CARTESIAN_POINT('Ctrl Pts',(149.596474789369,-80.752057129177,47.0574871779499));
#18336=CARTESIAN_POINT('Ctrl Pts',(149.598641974416,-80.7480423306098,47.0537929494384));
#18337=CARTESIAN_POINT('Ctrl Pts',(149.600807137209,-80.7440308818109,47.050091283938));
#18338=CARTESIAN_POINT('Ctrl Pts',(149.602970226706,-80.7400228807506,47.0463821931637));
#18339=CARTESIAN_POINT('Ctrl Pts',(149.665071318886,-80.6249554072859,46.9398962671819));
#18340=CARTESIAN_POINT('Ctrl Pts',(149.72550325001,-80.5126559819617,46.8272204519951));
#18341=CARTESIAN_POINT('Ctrl Pts',(149.783030801752,-80.4054929778246,46.7086718150296));
#18342=CARTESIAN_POINT('Ctrl Pts',(149.809543928151,-80.3561040122254,46.6540354729443));
#18343=CARTESIAN_POINT('Ctrl Pts',(149.835440369712,-80.3078056559303,46.5981521261349));
#18344=CARTESIAN_POINT('Ctrl Pts',(149.860600799428,-80.260826858675,46.5410549251661));
#18345=CARTESIAN_POINT('Ctrl Pts',(149.862244464557,-80.2577578566065,46.5373249142225));
#18346=CARTESIAN_POINT('Ctrl Pts',(149.863885113163,-80.2546942576169,46.5335897131967));
#18347=CARTESIAN_POINT('Ctrl Pts',(149.865522721631,-80.2516361085815,46.5298492852785));
#18348=CARTESIAN_POINT('Ctrl Pts',(149.920874283176,-80.148269932952,46.4034219187085));
#18349=CARTESIAN_POINT('Ctrl Pts',(149.972772946679,-80.0510921736928,46.2709925001795));
#18350=CARTESIAN_POINT('Ctrl Pts',(150.020328326584,-79.961871940831,46.1310781770696));
#18351=CARTESIAN_POINT('Ctrl Pts',(150.041423437799,-79.9222946997582,46.0690135229251));
#18352=CARTESIAN_POINT('Ctrl Pts',(150.061664115444,-79.884282891071,46.0054765146034));
#18353=CARTESIAN_POINT('Ctrl Pts',(150.080973718749,-79.8479888765764,45.9403401621094));
#18354=CARTESIAN_POINT('Ctrl Pts',(150.081910893431,-79.8462273783758,45.9371788262994));
#18355=CARTESIAN_POINT('Ctrl Pts',(150.082845417364,-79.8444707888363,45.9340152250091));
#18356=CARTESIAN_POINT('Ctrl Pts',(150.083777280819,-79.842719127427,45.9308493494822));
#18357=CARTESIAN_POINT('Ctrl Pts',(150.124316972743,-79.7665150295208,45.7931214259646));
#18358=CARTESIAN_POINT('Ctrl Pts',(150.159836015379,-79.6996105779127,45.6510364734858));
#18359=CARTESIAN_POINT('Ctrl Pts',(150.189536570941,-79.643601630539,45.5038983003528));
#18360=CARTESIAN_POINT('Ctrl Pts',(150.205994764956,-79.6125649679259,45.4223635090175));
#18361=CARTESIAN_POINT('Ctrl Pts',(150.22066665991,-79.5848732537911,45.3392772231722));
#18362=CARTESIAN_POINT('Ctrl Pts',(150.233419649245,-79.5607919801431,45.2545226584932));
#18363=CARTESIAN_POINT('Ctrl Pts',(150.233653158554,-79.5603510481059,45.252970788629));
#18364=CARTESIAN_POINT('Ctrl Pts',(150.233885994755,-79.5599113833124,45.2514181977489));
#18365=CARTESIAN_POINT('Ctrl Pts',(150.234118156878,-79.5594729876405,45.2498648923104));
#18366=CARTESIAN_POINT('Ctrl Pts',(150.243593980634,-79.5415796290569,45.1864658831964));
#18367=CARTESIAN_POINT('Ctrl Pts',(150.251930637624,-79.5258311439937,45.1219886580334));
#18368=CARTESIAN_POINT('Ctrl Pts',(150.25908694937,-79.5123085902624,45.0567119030525));
#18369=CARTESIAN_POINT('Ctrl Pts',(150.266133192886,-79.4989940212598,44.9924391424681));
#18370=CARTESIAN_POINT('Ctrl Pts',(150.272035277524,-79.4878371314994,44.9273898861929));
#18371=CARTESIAN_POINT('Ctrl Pts',(150.276731655023,-79.4789572453975,44.8618164804335));
#18372=CARTESIAN_POINT('Ctrl Pts',(150.281154338818,-79.4705948579246,44.8000645367055));
#18373=CARTESIAN_POINT('Ctrl Pts',(150.284507727575,-79.4642518495708,44.7378467346804));
#18374=CARTESIAN_POINT('Ctrl Pts',(150.286719886614,-79.4600667280322,44.6753785307951));
#18375=CARTESIAN_POINT('Ctrl Pts',(150.28878458935,-79.4561605749315,44.6170742817893));
#18376=CARTESIAN_POINT('Ctrl Pts',(150.289855072332,-79.4541343313065,44.5585512837797));
#18377=CARTESIAN_POINT('Ctrl Pts',(150.289855072464,-79.4541343310581,44.5));
#18378=CARTESIAN_POINT('',(150.289855072464,-79.4541343310581,37.5));
#18379=CARTESIAN_POINT('',(150.289855072464,-79.4541343310581,115.));
#18380=CARTESIAN_POINT('',(145.36231884058,-88.1464478086873,32.5));
#18381=CARTESIAN_POINT('Ctrl Pts',(150.289855072464,-79.4541343310581,37.5));
#18382=CARTESIAN_POINT('Ctrl Pts',(150.289855068577,-79.4541343384106,37.2436476198539));
#18383=CARTESIAN_POINT('Ctrl Pts',(150.270581238553,-79.4906188049207,36.9946184779966));
#18384=CARTESIAN_POINT('Ctrl Pts',(150.23440031069,-79.5589401936918,36.7519883573953));
#18385=CARTESIAN_POINT('Ctrl Pts',(150.233993766309,-79.5597078820386,36.7492620615822));
#18386=CARTESIAN_POINT('Ctrl Pts',(150.2335850823,-79.5604795994257,36.7465365450198));
#18387=CARTESIAN_POINT('Ctrl Pts',(150.233174261933,-79.5612553394204,36.7438118068128));
#18388=CARTESIAN_POINT('Ctrl Pts',(150.211108362005,-79.6029217280991,36.597461222919));
#18389=CARTESIAN_POINT('Ctrl Pts',(150.183223768723,-79.6555340186059,36.4560333910476));
#18390=CARTESIAN_POINT('Ctrl Pts',(150.150657295397,-79.7168744981781,36.3199679218119));
#18391=CARTESIAN_POINT('Ctrl Pts',(150.129869982028,-79.7560283776372,36.2331167752582));
#18392=CARTESIAN_POINT('Ctrl Pts',(150.107175698373,-79.7987372958168,36.1484502336036));
#18393=CARTESIAN_POINT('Ctrl Pts',(150.082875014061,-79.8444151271613,36.0660801928035));
#18394=CARTESIAN_POINT('Ctrl Pts',(150.081600916097,-79.8468100404567,36.0617614872072));
#18395=CARTESIAN_POINT('Ctrl Pts',(150.080322360848,-79.8492131928944,36.0574489500033));
#18396=CARTESIAN_POINT('Ctrl Pts',(150.079039391808,-79.8516244996445,36.05314260126));
#18397=CARTESIAN_POINT('Ctrl Pts',(150.044542112121,-79.9164612343937,35.9373507837354));
#18398=CARTESIAN_POINT('Ctrl Pts',(150.006537123162,-79.9877842271916,35.8251345490234));
#18399=CARTESIAN_POINT('Ctrl Pts',(149.965970804577,-80.0637685565931,35.717265369449));
#18400=CARTESIAN_POINT('Ctrl Pts',(149.933351576219,-80.124867277869,35.6305281568029));
#18401=CARTESIAN_POINT('Ctrl Pts',(149.899077126142,-80.1889782570248,35.5466015578877));
#18402=CARTESIAN_POINT('Ctrl Pts',(149.863649966461,-80.255133246411,35.4658772780751));
#18403=CARTESIAN_POINT('Ctrl Pts',(149.861515024356,-80.2591199355374,35.4610126017817));
#18404=CARTESIAN_POINT('Ctrl Pts',(149.85937578758,-80.2631142503699,35.4561592869362));
#18405=CARTESIAN_POINT('Ctrl Pts',(149.857232364154,-80.2671159825673,35.4513174183972));
#18406=CARTESIAN_POINT('Ctrl Pts',(149.804252858278,-80.3660277477068,35.331639803768));
#18407=CARTESIAN_POINT('Ctrl Pts',(149.748484158478,-80.4699094430571,35.2180933719206));
#18408=CARTESIAN_POINT('Ctrl Pts',(149.690355247896,-80.5778965450401,35.1097499748562));
#18409=CARTESIAN_POINT('Ctrl Pts',(149.661473306407,-80.6315510369237,35.0559184541312));
#18410=CARTESIAN_POINT('Ctrl Pts',(149.63200898673,-80.6862185045824,35.0033707288664));
#18411=CARTESIAN_POINT('Ctrl Pts',(149.60201639041,-80.741790230842,34.9519894923051));
#18412=CARTESIAN_POINT('Ctrl Pts',(149.599223408299,-80.7469652025476,34.9472047489959));
#18413=CARTESIAN_POINT('Ctrl Pts',(149.596425806469,-80.7521480873936,34.9424300694399));
#18414=CARTESIAN_POINT('Ctrl Pts',(149.593623625112,-80.7573388040449,34.9376653528747));
#18415=CARTESIAN_POINT('Ctrl Pts',(149.503321107799,-80.9246137661054,34.7841185815494));
#18416=CARTESIAN_POINT('Ctrl Pts',(149.407759531995,-81.1009468141059,34.6404004213219));
#18417=CARTESIAN_POINT('Ctrl Pts',(149.309404815745,-81.2816192446479,34.5068550549142));
#18418=CARTESIAN_POINT('Ctrl Pts',(149.306147321137,-81.2876030905749,34.5024320508374));
#18419=CARTESIAN_POINT('Ctrl Pts',(149.302886794892,-81.2935916372183,34.498020248125));
#18420=CARTESIAN_POINT('Ctrl Pts',(149.299623326396,-81.2995847135534,34.4936196571957));
#18421=CARTESIAN_POINT('Ctrl Pts',(149.201294060241,-81.4801578671638,34.3610285574972));
#18422=CARTESIAN_POINT('Ctrl Pts',(149.100390942177,-81.6646756184357,34.2385852650971));
#18423=CARTESIAN_POINT('Ctrl Pts',(148.997297013874,-81.8523394986245,34.1242886774831));
#18424=CARTESIAN_POINT('Ctrl Pts',(148.993783486671,-81.8587352404397,34.1203933542914));
#18425=CARTESIAN_POINT('Ctrl Pts',(148.99026742009,-81.8651346268365,34.1165075135218));
#18426=CARTESIAN_POINT('Ctrl Pts',(148.986748829868,-81.871537625153,34.1126310765379));
#18427=CARTESIAN_POINT('Ctrl Pts',(148.82898957284,-82.158621995175,33.9388274279259));
#18428=CARTESIAN_POINT('Ctrl Pts',(148.666197518725,-82.4528887104821,33.7837344929974));
#18429=CARTESIAN_POINT('Ctrl Pts',(148.499047675039,-82.7528397905726,33.6438439855164));
#18430=CARTESIAN_POINT('Ctrl Pts',(148.443888606591,-82.8518229651463,33.5976804360501));
#18431=CARTESIAN_POINT('Ctrl Pts',(148.388255039764,-82.95142505779,33.5531719899696));
#18432=CARTESIAN_POINT('Ctrl Pts',(148.332171389768,-83.0515919680528,33.5101914075088));
#18433=CARTESIAN_POINT('Ctrl Pts',(148.328463625565,-83.0582141348388,33.507349904413));
#18434=CARTESIAN_POINT('Ctrl Pts',(148.324753888106,-83.0648387811286,33.5045150857075));
#18435=CARTESIAN_POINT('Ctrl Pts',(148.321042184227,-83.0714658916725,33.5016869147104));
#18436=CARTESIAN_POINT('Ctrl Pts',(148.127526079484,-83.4169817679298,33.3542353256982));
#18437=CARTESIAN_POINT('Ctrl Pts',(147.928023779053,-83.7703038873448,33.224894934723));
#18438=CARTESIAN_POINT('Ctrl Pts',(147.726117191227,-84.1248695147591,33.1128740239443));
#18439=CARTESIAN_POINT('Ctrl Pts',(147.691851026841,-84.1850438964133,33.0938626237485));
#18440=CARTESIAN_POINT('Ctrl Pts',(147.657515670422,-84.2452539899407,33.0753500432994));
#18441=CARTESIAN_POINT('Ctrl Pts',(147.623128700903,-84.3054675885421,33.0573323830867));
#18442=CARTESIAN_POINT('Ctrl Pts',(147.61966084937,-84.3115399997818,33.0555153410077));
#18443=CARTESIAN_POINT('Ctrl Pts',(147.616192453019,-84.3176124815105,33.0537033222415));
#18444=CARTESIAN_POINT('Ctrl Pts',(147.612723530195,-84.3236850001122,33.0518963231399));
#18445=CARTESIAN_POINT('Ctrl Pts',(147.414398057485,-84.6708634135347,32.9485864574506));
#18446=CARTESIAN_POINT('Ctrl Pts',(147.213653682843,-85.0194306321787,32.8611210650963));
#18447=CARTESIAN_POINT('Ctrl Pts',(147.010609976479,-85.3690841855062,32.78802258227));
#18448=CARTESIAN_POINT('Ctrl Pts',(146.970506380411,-85.4381450055505,32.7735847448165));
#18449=CARTESIAN_POINT('Ctrl Pts',(146.930313102768,-85.5072481940713,32.7597072133851));
#18450=CARTESIAN_POINT('Ctrl Pts',(146.89003109062,-85.5763914060563,32.746378371904));
#18451=CARTESIAN_POINT('Ctrl Pts',(146.887290932544,-85.5810948287668,32.745471685999));
#18452=CARTESIAN_POINT('Ctrl Pts',(146.884550362083,-85.5857984397406,32.7445675390721));
#18453=CARTESIAN_POINT('Ctrl Pts',(146.881809379355,-85.5905022385503,32.7436659274155));
#18454=CARTESIAN_POINT('Ctrl Pts',(146.534412670975,-86.1866695207185,32.6293941669531));
#18455=CARTESIAN_POINT('Ctrl Pts',(146.180413916128,-86.7858240348916,32.5551812170606));
#18456=CARTESIAN_POINT('Ctrl Pts',(145.819603406855,-87.3878896742938,32.5213077186522));
#18457=CARTESIAN_POINT('Ctrl Pts',(145.668377266016,-87.6402328318194,32.5071103538045));
#18458=CARTESIAN_POINT('Ctrl Pts',(145.515954394551,-87.8930873961367,32.5000000002681));
#18459=CARTESIAN_POINT('Ctrl Pts',(145.36231884058,-88.1464478086873,32.5));
#18460=CARTESIAN_POINT('Origin',(0.,0.,32.5));
#18461=CARTESIAN_POINT('',(-145.36231884058,-88.1464478086873,-49.5));
#18462=CARTESIAN_POINT('Origin',(0.,0.,-49.5));
#18463=CARTESIAN_POINT('',(-150.289855072464,-79.4541343310581,-44.5));
#18464=CARTESIAN_POINT('Ctrl Pts',(-145.36231884058,-88.1464478086873,-49.5));
#18465=CARTESIAN_POINT('Ctrl Pts',(-145.729245608051,-87.5413488274995,
-49.4999999993448));
#18466=CARTESIAN_POINT('Ctrl Pts',(-146.089427497743,-86.938852139224,-49.459451627546));
#18467=CARTESIAN_POINT('Ctrl Pts',(-146.443059008834,-86.3390437438767,
-49.3785345234731));
#18468=CARTESIAN_POINT('Ctrl Pts',(-146.591729818533,-86.0868773022461,
-49.3445160296351));
#18469=CARTESIAN_POINT('Ctrl Pts',(-146.739242767663,-85.8351860376504,
-49.3033619016674));
#18470=CARTESIAN_POINT('Ctrl Pts',(-146.885611849037,-85.5839764893769,
-49.2550827834563));
#18471=CARTESIAN_POINT('Ctrl Pts',(-146.887215711036,-85.581223821639,-49.2545537575016));
#18472=CARTESIAN_POINT('Ctrl Pts',(-146.888819435246,-85.5784712124141,
-49.2540238618083));
#18473=CARTESIAN_POINT('Ctrl Pts',(-146.890423021642,-85.5757186617924,
-49.2534930956204));
#18474=CARTESIAN_POINT('Ctrl Pts',(-147.136163003217,-85.1539068149984,
-49.1721563659123));
#18475=CARTESIAN_POINT('Ctrl Pts',(-147.378654044698,-84.733492627337,-49.0703840441395));
#18476=CARTESIAN_POINT('Ctrl Pts',(-147.617771548819,-84.3148475830954,
-48.9454703779811));
#18477=CARTESIAN_POINT('Ctrl Pts',(-147.619992196193,-84.3109596911514,
-48.9443103240332));
#18478=CARTESIAN_POINT('Ctrl Pts',(-147.622212556282,-84.307071941363,-48.943148258573));
#18479=CARTESIAN_POINT('Ctrl Pts',(-147.624432625828,-84.303184339794,-48.9419841796181));
#18480=CARTESIAN_POINT('Ctrl Pts',(-147.797445356911,-84.0002188016352,
-48.8512660849843));
#18481=CARTESIAN_POINT('Ctrl Pts',(-147.968707326118,-83.6981287755317,
-48.7483109143164));
#18482=CARTESIAN_POINT('Ctrl Pts',(-148.136615104019,-83.3998939012959,
-48.6322285684957));
#18483=CARTESIAN_POINT('Ctrl Pts',(-148.200188500854,-83.2869759397415,
-48.5882773642776));
#18484=CARTESIAN_POINT('Ctrl Pts',(-148.263281189795,-83.1746104678287,
-48.5424447848479));
#18485=CARTESIAN_POINT('Ctrl Pts',(-148.325806750807,-83.0629583612551,
-48.4946842709289));
#18486=CARTESIAN_POINT('Ctrl Pts',(-148.328437713,-83.0582602431345,-48.4926745951353));
#18487=CARTESIAN_POINT('Ctrl Pts',(-148.331067922545,-83.0535629380485,
-48.4906613522023));
#18488=CARTESIAN_POINT('Ctrl Pts',(-148.333697371916,-83.0488664605796,
-48.4886445330394));
#18489=CARTESIAN_POINT('Ctrl Pts',(-148.479392264376,-82.7886398186652,
-48.3768948053783));
#18490=CARTESIAN_POINT('Ctrl Pts',(-148.622808981178,-82.5308543489962,
-48.2541267340886));
#18491=CARTESIAN_POINT('Ctrl Pts',(-148.762663381336,-82.2779954776877,
-48.1187795814413));
#18492=CARTESIAN_POINT('Ctrl Pts',(-148.840976563632,-82.1364040593145,
-48.0429902875284));
#18493=CARTESIAN_POINT('Ctrl Pts',(-148.918172933796,-81.9963571587517,
-47.9632574413117));
#18494=CARTESIAN_POINT('Ctrl Pts',(-148.994029023493,-81.8582880066048,
-47.8793133555439));
#18495=CARTESIAN_POINT('Ctrl Pts',(-148.996712266487,-81.8534041128184,
-47.8763440174079));
#18496=CARTESIAN_POINT('Ctrl Pts',(-148.999393672824,-81.8485229853453,
-47.8733697901463));
#18497=CARTESIAN_POINT('Ctrl Pts',(-149.002073232327,-81.8436446453373,
-47.8703906395336));
#18498=CARTESIAN_POINT('Ctrl Pts',(-149.107681065302,-81.6513776267181,
-47.7529752061311));
#18499=CARTESIAN_POINT('Ctrl Pts',(-149.210443318177,-81.4633981454557,
-47.6279048759376));
#18500=CARTESIAN_POINT('Ctrl Pts',(-149.309720948425,-81.2810297213993,
-47.4931045485117));
#18501=CARTESIAN_POINT('Ctrl Pts',(-149.401996350024,-81.111524068145,-47.3678119290385));
#18502=CARTESIAN_POINT('Ctrl Pts',(-149.491261252891,-80.9468661107977,
-47.2341131033335));
#18503=CARTESIAN_POINT('Ctrl Pts',(-149.577013895448,-80.7880986852943,
-47.0903818425147));
#18504=CARTESIAN_POINT('Ctrl Pts',(-149.583521150904,-80.7760507744081,
-47.0794749362875));
#18505=CARTESIAN_POINT('Ctrl Pts',(-149.590008187584,-80.7640367723622,
-47.0685102812695));
#18506=CARTESIAN_POINT('Ctrl Pts',(-149.596474789369,-80.752057129177,-47.0574871779499));
#18507=CARTESIAN_POINT('Ctrl Pts',(-149.598641974416,-80.7480423306098,
-47.0537929494384));
#18508=CARTESIAN_POINT('Ctrl Pts',(-149.600807137209,-80.7440308818109,
-47.050091283938));
#18509=CARTESIAN_POINT('Ctrl Pts',(-149.602970226706,-80.7400228807506,
-47.0463821931637));
#18510=CARTESIAN_POINT('Ctrl Pts',(-149.665071318886,-80.6249554072859,
-46.9398962671819));
#18511=CARTESIAN_POINT('Ctrl Pts',(-149.72550325001,-80.5126559819617,-46.8272204519951));
#18512=CARTESIAN_POINT('Ctrl Pts',(-149.783030801752,-80.4054929778246,
-46.7086718150296));
#18513=CARTESIAN_POINT('Ctrl Pts',(-149.809543928151,-80.3561040122254,
-46.6540354729443));
#18514=CARTESIAN_POINT('Ctrl Pts',(-149.835440369712,-80.3078056559303,
-46.5981521261349));
#18515=CARTESIAN_POINT('Ctrl Pts',(-149.860600799428,-80.260826858675,-46.5410549251661));
#18516=CARTESIAN_POINT('Ctrl Pts',(-149.862244464557,-80.2577578566065,
-46.5373249142225));
#18517=CARTESIAN_POINT('Ctrl Pts',(-149.863885113163,-80.2546942576169,
-46.5335897131967));
#18518=CARTESIAN_POINT('Ctrl Pts',(-149.865522721631,-80.2516361085815,
-46.5298492852785));
#18519=CARTESIAN_POINT('Ctrl Pts',(-149.920874283176,-80.148269932952,-46.4034219187085));
#18520=CARTESIAN_POINT('Ctrl Pts',(-149.972772946679,-80.0510921736928,
-46.2709925001795));
#18521=CARTESIAN_POINT('Ctrl Pts',(-150.020328326584,-79.961871940831,-46.1310781770696));
#18522=CARTESIAN_POINT('Ctrl Pts',(-150.041423437799,-79.9222946997582,
-46.0690135229251));
#18523=CARTESIAN_POINT('Ctrl Pts',(-150.061664115444,-79.884282891071,-46.0054765146034));
#18524=CARTESIAN_POINT('Ctrl Pts',(-150.080973718749,-79.8479888765764,
-45.9403401621094));
#18525=CARTESIAN_POINT('Ctrl Pts',(-150.081910893431,-79.8462273783758,
-45.9371788262994));
#18526=CARTESIAN_POINT('Ctrl Pts',(-150.082845417364,-79.8444707888363,
-45.9340152250091));
#18527=CARTESIAN_POINT('Ctrl Pts',(-150.083777280819,-79.842719127427,-45.9308493494822));
#18528=CARTESIAN_POINT('Ctrl Pts',(-150.124316972743,-79.7665150295208,
-45.7931214259646));
#18529=CARTESIAN_POINT('Ctrl Pts',(-150.159836015379,-79.6996105779127,
-45.6510364734858));
#18530=CARTESIAN_POINT('Ctrl Pts',(-150.189536570941,-79.643601630539,-45.5038983003528));
#18531=CARTESIAN_POINT('Ctrl Pts',(-150.205994764956,-79.6125649679259,
-45.4223635090175));
#18532=CARTESIAN_POINT('Ctrl Pts',(-150.22066665991,-79.5848732537911,-45.3392772231722));
#18533=CARTESIAN_POINT('Ctrl Pts',(-150.233419649245,-79.5607919801431,
-45.2545226584932));
#18534=CARTESIAN_POINT('Ctrl Pts',(-150.233653158554,-79.5603510481059,
-45.252970788629));
#18535=CARTESIAN_POINT('Ctrl Pts',(-150.233885994755,-79.5599113833124,
-45.2514181977489));
#18536=CARTESIAN_POINT('Ctrl Pts',(-150.234118156878,-79.5594729876405,
-45.2498648923104));
#18537=CARTESIAN_POINT('Ctrl Pts',(-150.243593980634,-79.5415796290569,
-45.1864658831964));
#18538=CARTESIAN_POINT('Ctrl Pts',(-150.251930637624,-79.5258311439937,
-45.1219886580334));
#18539=CARTESIAN_POINT('Ctrl Pts',(-150.25908694937,-79.5123085902624,-45.0567119030525));
#18540=CARTESIAN_POINT('Ctrl Pts',(-150.266133192886,-79.4989940212598,
-44.9924391424681));
#18541=CARTESIAN_POINT('Ctrl Pts',(-150.272035277524,-79.4878371314994,
-44.9273898861929));
#18542=CARTESIAN_POINT('Ctrl Pts',(-150.276731655023,-79.4789572453975,
-44.8618164804335));
#18543=CARTESIAN_POINT('Ctrl Pts',(-150.281154338818,-79.4705948579246,
-44.8000645367055));
#18544=CARTESIAN_POINT('Ctrl Pts',(-150.284507727575,-79.4642518495708,
-44.7378467346804));
#18545=CARTESIAN_POINT('Ctrl Pts',(-150.286719886614,-79.4600667280322,
-44.6753785307951));
#18546=CARTESIAN_POINT('Ctrl Pts',(-150.28878458935,-79.4561605749315,-44.6170742817893));
#18547=CARTESIAN_POINT('Ctrl Pts',(-150.289855072332,-79.4541343313065,
-44.5585512837797));
#18548=CARTESIAN_POINT('Ctrl Pts',(-150.289855072464,-79.4541343310581,
-44.5));
#18549=CARTESIAN_POINT('',(-150.289855072464,-79.4541343310581,-37.5));
#18550=CARTESIAN_POINT('',(-150.289855072464,-79.4541343310581,115.));
#18551=CARTESIAN_POINT('',(-145.36231884058,-88.1464478086873,-32.5));
#18552=CARTESIAN_POINT('Ctrl Pts',(-150.289855072464,-79.4541343310581,
-37.5));
#18553=CARTESIAN_POINT('Ctrl Pts',(-150.289855068577,-79.4541343384106,
-37.2436476198539));
#18554=CARTESIAN_POINT('Ctrl Pts',(-150.270581238553,-79.4906188049207,
-36.9946184779967));
#18555=CARTESIAN_POINT('Ctrl Pts',(-150.234400310691,-79.5589401936912,
-36.751988357395));
#18556=CARTESIAN_POINT('Ctrl Pts',(-150.23399376631,-79.559707882038,-36.7492620615819));
#18557=CARTESIAN_POINT('Ctrl Pts',(-150.2335850823,-79.5604795994251,-36.7465365450195));
#18558=CARTESIAN_POINT('Ctrl Pts',(-150.233174261933,-79.5612553394198,
-36.7438118068126));
#18559=CARTESIAN_POINT('Ctrl Pts',(-150.211108362071,-79.6029217279729,
-36.597461223358));
#18560=CARTESIAN_POINT('Ctrl Pts',(-150.183223768892,-79.6555340182885,
-36.4560333918963));
#18561=CARTESIAN_POINT('Ctrl Pts',(-150.150657295691,-79.7168744976241,
-36.3199679230369));
#18562=CARTESIAN_POINT('Ctrl Pts',(-150.129869982242,-79.756028377234,-36.233116776054));
#18563=CARTESIAN_POINT('Ctrl Pts',(-150.107175698488,-79.7987372956008,
-36.1484502339904));
#18564=CARTESIAN_POINT('Ctrl Pts',(-150.082875014062,-79.8444151271605,
-36.0660801928029));
#18565=CARTESIAN_POINT('Ctrl Pts',(-150.081600916097,-79.8468100404559,
-36.0617614872067));
#18566=CARTESIAN_POINT('Ctrl Pts',(-150.080322360849,-79.8492131928936,
-36.0574489500027));
#18567=CARTESIAN_POINT('Ctrl Pts',(-150.079039391808,-79.8516244996438,
-36.0531426012594));
#18568=CARTESIAN_POINT('Ctrl Pts',(-150.044542112236,-79.9164612341789,
-35.9373507841183));
#18569=CARTESIAN_POINT('Ctrl Pts',(-150.006537123414,-79.9877842267191,
-35.8251345497657));
#18570=CARTESIAN_POINT('Ctrl Pts',(-149.96597080498,-80.0637685558382,-35.7172653705196));
#18571=CARTESIAN_POINT('Ctrl Pts',(-149.933351576501,-80.1248672773407,
-35.6305281574933));
#18572=CARTESIAN_POINT('Ctrl Pts',(-149.899077126288,-80.188978256752,-35.5466015582195));
#18573=CARTESIAN_POINT('Ctrl Pts',(-149.863649966461,-80.2551332464107,
-35.4658772780747));
#18574=CARTESIAN_POINT('Ctrl Pts',(-149.861515024356,-80.259119935537,-35.4610126017813));
#18575=CARTESIAN_POINT('Ctrl Pts',(-149.85937578758,-80.2631142503696,-35.4561592869359));
#18576=CARTESIAN_POINT('Ctrl Pts',(-149.857232364154,-80.267115982567,-35.4513174183969));
#18577=CARTESIAN_POINT('Ctrl Pts',(-149.804252858374,-80.3660277475268,
-35.3316398039859));
#18578=CARTESIAN_POINT('Ctrl Pts',(-149.748484158681,-80.4699094426787,
-35.2180933723342));
#18579=CARTESIAN_POINT('Ctrl Pts',(-149.690355248213,-80.57789654445,-35.1097499754482));
#18580=CARTESIAN_POINT('Ctrl Pts',(-149.661473306623,-80.6315510365229,
-35.0559184545164));
#18581=CARTESIAN_POINT('Ctrl Pts',(-149.63200898684,-80.6862185043787,-35.0033707290548));
#18582=CARTESIAN_POINT('Ctrl Pts',(-149.60201639041,-80.741790230842,-34.9519894923051));
#18583=CARTESIAN_POINT('Ctrl Pts',(-149.599223408299,-80.7469652025476,
-34.9472047489958));
#18584=CARTESIAN_POINT('Ctrl Pts',(-149.596425806469,-80.7521480873936,
-34.9424300694399));
#18585=CARTESIAN_POINT('Ctrl Pts',(-149.593623625112,-80.7573388040449,
-34.9376653528747));
#18586=CARTESIAN_POINT('Ctrl Pts',(-149.503321107799,-80.9246137661054,
-34.7841185815493));
#18587=CARTESIAN_POINT('Ctrl Pts',(-149.407759531995,-81.1009468141073,
-34.6404004213243));
#18588=CARTESIAN_POINT('Ctrl Pts',(-149.309404815744,-81.2816192446487,
-34.5068550549154));
#18589=CARTESIAN_POINT('Ctrl Pts',(-149.306147321137,-81.2876030905756,
-34.5024320508386));
#18590=CARTESIAN_POINT('Ctrl Pts',(-149.302886794892,-81.293591637219,-34.4980202481262));
#18591=CARTESIAN_POINT('Ctrl Pts',(-149.299623326396,-81.2995847135541,
-34.4936196571968));
#18592=CARTESIAN_POINT('Ctrl Pts',(-149.201294060242,-81.4801578671635,
-34.3610285574967));
#18593=CARTESIAN_POINT('Ctrl Pts',(-149.100390942177,-81.6646756184357,
-34.2385852650972));
#18594=CARTESIAN_POINT('Ctrl Pts',(-148.997297013874,-81.8523394986246,
-34.1242886774832));
#18595=CARTESIAN_POINT('Ctrl Pts',(-148.993783486671,-81.8587352404398,
-34.1203933542915));
#18596=CARTESIAN_POINT('Ctrl Pts',(-148.99026742009,-81.8651346268366,-34.1165075135219));
#18597=CARTESIAN_POINT('Ctrl Pts',(-148.986748829868,-81.8715376251531,
-34.112631076538));
#18598=CARTESIAN_POINT('Ctrl Pts',(-148.828989574134,-82.1586219928198,
-33.9388274293518));
#18599=CARTESIAN_POINT('Ctrl Pts',(-148.666197521396,-82.4528887056537,
-33.783734495542));
#18600=CARTESIAN_POINT('Ctrl Pts',(-148.499047679152,-82.7528397831901,
-33.6438439889596));
#18601=CARTESIAN_POINT('Ctrl Pts',(-148.443888609357,-82.851822960194,-33.5976804382634));
#18602=CARTESIAN_POINT('Ctrl Pts',(-148.388255041158,-82.9514250552998,
-33.5531719910385));
#18603=CARTESIAN_POINT('Ctrl Pts',(-148.332171389768,-83.0515919680529,
-33.5101914075093));
#18604=CARTESIAN_POINT('Ctrl Pts',(-148.328463625565,-83.0582141348389,
-33.5073499044134));
#18605=CARTESIAN_POINT('Ctrl Pts',(-148.324753888106,-83.0648387811287,
-33.504515085708));
#18606=CARTESIAN_POINT('Ctrl Pts',(-148.321042184227,-83.0714658916727,
-33.5016869147109));
#18607=CARTESIAN_POINT('Ctrl Pts',(-148.12752607943,-83.4169817680272,-33.3542353256577));
#18608=CARTESIAN_POINT('Ctrl Pts',(-147.928023778942,-83.7703038875428,
-33.224894934649));
#18609=CARTESIAN_POINT('Ctrl Pts',(-147.726117191057,-84.1248695150572,
-33.1128740238486));
#18610=CARTESIAN_POINT('Ctrl Pts',(-147.691851026728,-84.1850438966121,
-33.0938626236858));
#18611=CARTESIAN_POINT('Ctrl Pts',(-147.657515670366,-84.24525399004,-33.0753500432682));
#18612=CARTESIAN_POINT('Ctrl Pts',(-147.623128700903,-84.3054675885418,
-33.0573323830855));
#18613=CARTESIAN_POINT('Ctrl Pts',(-147.61966084937,-84.3115399997815,-33.0555153410065));
#18614=CARTESIAN_POINT('Ctrl Pts',(-147.616192453019,-84.3176124815102,
-33.0537033222403));
#18615=CARTESIAN_POINT('Ctrl Pts',(-147.612723530195,-84.323685000112,-33.0518963231388));
#18616=CARTESIAN_POINT('Ctrl Pts',(-147.414398058157,-84.6708634123572,
-32.948586457801));
#18617=CARTESIAN_POINT('Ctrl Pts',(-147.213653684205,-85.0194306298146,
-32.8611210656896));
#18618=CARTESIAN_POINT('Ctrl Pts',(-147.010609978545,-85.3690841819489,
-32.7880225830139));
#18619=CARTESIAN_POINT('Ctrl Pts',(-146.970506381792,-85.4381450031775,
-32.7735847452933));
#18620=CARTESIAN_POINT('Ctrl Pts',(-146.93031310346,-85.5072481928842,-32.7597072136142));
#18621=CARTESIAN_POINT('Ctrl Pts',(-146.89003109062,-85.5763914060563,-32.7463783719042));
#18622=CARTESIAN_POINT('Ctrl Pts',(-146.887290932544,-85.5810948287669,
-32.7454716859993));
#18623=CARTESIAN_POINT('Ctrl Pts',(-146.884550362083,-85.5857984397407,
-32.7445675390723));
#18624=CARTESIAN_POINT('Ctrl Pts',(-146.881809379355,-85.5905022385503,
-32.7436659274158));
#18625=CARTESIAN_POINT('Ctrl Pts',(-146.53441266257,-86.186669535143,-32.6293941641891));
#18626=CARTESIAN_POINT('Ctrl Pts',(-146.180413898998,-86.7858240638849,
-32.5551812134692));
#18627=CARTESIAN_POINT('Ctrl Pts',(-145.819603380665,-87.3878897179948,
-32.5213077161934));
#18628=CARTESIAN_POINT('Ctrl Pts',(-145.668377248418,-87.6402328610125,
-32.5071103529836));
#18629=CARTESIAN_POINT('Ctrl Pts',(-145.515954385683,-87.8930874107624,
-32.5000000002681));
#18630=CARTESIAN_POINT('Ctrl Pts',(-145.36231884058,-88.1464478086873,-32.5));
#18631=CARTESIAN_POINT('Origin',(0.,0.,-32.5));
#18632=CARTESIAN_POINT('',(-119.689439203101,-120.724637681159,115.));
#18633=CARTESIAN_POINT('',(-145.36231884058,-88.1464478086873,32.5));
#18634=CARTESIAN_POINT('Origin',(0.,0.,32.5));
#18635=CARTESIAN_POINT('',(-150.289855072464,-79.4541343310581,37.5));
#18636=CARTESIAN_POINT('Ctrl Pts',(-145.36231884058,-88.1464478086873,32.5));
#18637=CARTESIAN_POINT('Ctrl Pts',(-145.729245608041,-87.5413488275162,
32.5000000006552));
#18638=CARTESIAN_POINT('Ctrl Pts',(-146.089427497723,-86.9388521392574,
32.5405483724518));
#18639=CARTESIAN_POINT('Ctrl Pts',(-146.443059008805,-86.3390437439265,
32.6214654765202));
#18640=CARTESIAN_POINT('Ctrl Pts',(-146.591729818514,-86.0868773022792,
32.6554839703595));
#18641=CARTESIAN_POINT('Ctrl Pts',(-146.739242767653,-85.835186037667,32.6966380983294));
#18642=CARTESIAN_POINT('Ctrl Pts',(-146.885611849037,-85.5839764893769,
32.7449172165437));
#18643=CARTESIAN_POINT('Ctrl Pts',(-146.887215711036,-85.581223821639,32.7454462424984));
#18644=CARTESIAN_POINT('Ctrl Pts',(-146.888819435246,-85.5784712124141,
32.7459761381918));
#18645=CARTESIAN_POINT('Ctrl Pts',(-146.890423021642,-85.5757186617924,
32.7465069043797));
#18646=CARTESIAN_POINT('Ctrl Pts',(-147.136163003217,-85.1539068149984,
32.8278436340878));
#18647=CARTESIAN_POINT('Ctrl Pts',(-147.378654044698,-84.733492627337,32.9296159558605));
#18648=CARTESIAN_POINT('Ctrl Pts',(-147.617771548819,-84.3148475830954,
33.0545296220188));
#18649=CARTESIAN_POINT('Ctrl Pts',(-147.619992196193,-84.3109596911514,
33.0556896759668));
#18650=CARTESIAN_POINT('Ctrl Pts',(-147.622212556282,-84.307071941363,33.056851741427));
#18651=CARTESIAN_POINT('Ctrl Pts',(-147.624432625828,-84.303184339794,33.0580158203819));
#18652=CARTESIAN_POINT('Ctrl Pts',(-147.797445356911,-84.000218801635,33.1487339150158));
#18653=CARTESIAN_POINT('Ctrl Pts',(-147.968707326118,-83.6981287755313,
33.2516890856837));
#18654=CARTESIAN_POINT('Ctrl Pts',(-148.13661510402,-83.3998939012953,33.3677714315045));
#18655=CARTESIAN_POINT('Ctrl Pts',(-148.200188500854,-83.2869759397412,
33.4117226357226));
#18656=CARTESIAN_POINT('Ctrl Pts',(-148.263281189795,-83.1746104678285,
33.4575552151522));
#18657=CARTESIAN_POINT('Ctrl Pts',(-148.325806750807,-83.0629583612551,
33.5053157290711));
#18658=CARTESIAN_POINT('Ctrl Pts',(-148.328437713,-83.0582602431345,33.5073254048647));
#18659=CARTESIAN_POINT('Ctrl Pts',(-148.331067922545,-83.0535629380485,
33.5093386477977));
#18660=CARTESIAN_POINT('Ctrl Pts',(-148.333697371916,-83.0488664605796,
33.5113554669606));
#18661=CARTESIAN_POINT('Ctrl Pts',(-148.479392264378,-82.7886398186623,
33.6231051946229));
#18662=CARTESIAN_POINT('Ctrl Pts',(-148.622808981182,-82.5308543489905,
33.7458732659141));
#18663=CARTESIAN_POINT('Ctrl Pts',(-148.76266338134,-82.2779954776793,33.8812204185632));
#18664=CARTESIAN_POINT('Ctrl Pts',(-148.840976563635,-82.136404059309,33.9570097124747));
#18665=CARTESIAN_POINT('Ctrl Pts',(-148.918172933798,-81.996357158749,34.0367425586899));
#18666=CARTESIAN_POINT('Ctrl Pts',(-148.994029023493,-81.8582880066048,
34.1206866444561));
#18667=CARTESIAN_POINT('Ctrl Pts',(-148.996712266487,-81.8534041128184,
34.1236559825921));
#18668=CARTESIAN_POINT('Ctrl Pts',(-148.999393672824,-81.8485229853453,
34.1266302098537));
#18669=CARTESIAN_POINT('Ctrl Pts',(-149.002073232327,-81.8436446453373,
34.1296093604664));
#18670=CARTESIAN_POINT('Ctrl Pts',(-149.107681065302,-81.6513776267181,
34.2470247938689));
#18671=CARTESIAN_POINT('Ctrl Pts',(-149.210443318177,-81.4633981454557,
34.3720951240624));
#18672=CARTESIAN_POINT('Ctrl Pts',(-149.309720948425,-81.2810297213993,
34.5068954514883));
#18673=CARTESIAN_POINT('Ctrl Pts',(-149.401996350023,-81.1115240681461,
34.6321880709607));
#18674=CARTESIAN_POINT('Ctrl Pts',(-149.49126125289,-80.9468661107998,34.7658868966648));
#18675=CARTESIAN_POINT('Ctrl Pts',(-149.577013895446,-80.7880986852974,
34.9096181574825));
#18676=CARTESIAN_POINT('Ctrl Pts',(-149.583521150902,-80.7760507744102,
34.9205250637106));
#18677=CARTESIAN_POINT('Ctrl Pts',(-149.590008187584,-80.7640367723632,
34.9314897187296));
#18678=CARTESIAN_POINT('Ctrl Pts',(-149.596474789369,-80.752057129177,34.9425128220501));
#18679=CARTESIAN_POINT('Ctrl Pts',(-149.598641974416,-80.7480423306098,
34.9462070505616));
#18680=CARTESIAN_POINT('Ctrl Pts',(-149.600807137209,-80.7440308818109,
34.949908716062));
#18681=CARTESIAN_POINT('Ctrl Pts',(-149.602970226706,-80.7400228807506,
34.9536178068363));
#18682=CARTESIAN_POINT('Ctrl Pts',(-149.665071318885,-80.6249554072882,
35.060103732816));
#18683=CARTESIAN_POINT('Ctrl Pts',(-149.725503250007,-80.5126559819663,
35.1727795480004));
#18684=CARTESIAN_POINT('Ctrl Pts',(-149.783030801748,-80.4054929778311,
35.2913281849631));
#18685=CARTESIAN_POINT('Ctrl Pts',(-149.809543928148,-80.3561040122296,
35.3459645270507));
#18686=CARTESIAN_POINT('Ctrl Pts',(-149.835440369711,-80.3078056559324,
35.4018478738626));
#18687=CARTESIAN_POINT('Ctrl Pts',(-149.860600799428,-80.260826858675,35.4589450748339));
#18688=CARTESIAN_POINT('Ctrl Pts',(-149.862244464557,-80.2577578566065,
35.4626750857775));
#18689=CARTESIAN_POINT('Ctrl Pts',(-149.863885113163,-80.2546942576169,
35.4664102868033));
#18690=CARTESIAN_POINT('Ctrl Pts',(-149.865522721631,-80.2516361085815,
35.4701507147215));
#18691=CARTESIAN_POINT('Ctrl Pts',(-149.920874283176,-80.1482699329536,
35.5965780812897));
#18692=CARTESIAN_POINT('Ctrl Pts',(-149.972772946677,-80.0510921736956,
35.7290074998166));
#18693=CARTESIAN_POINT('Ctrl Pts',(-150.020328326582,-79.961871940835,35.8689218229242));
#18694=CARTESIAN_POINT('Ctrl Pts',(-150.041423437798,-79.9222946997607,
35.9309864770707));
#18695=CARTESIAN_POINT('Ctrl Pts',(-150.061664115444,-79.8842828910722,
35.9945234853944));
#18696=CARTESIAN_POINT('Ctrl Pts',(-150.080973718749,-79.8479888765764,
36.0596598378906));
#18697=CARTESIAN_POINT('Ctrl Pts',(-150.081910893431,-79.8462273783758,
36.0628211737006));
#18698=CARTESIAN_POINT('Ctrl Pts',(-150.082845417364,-79.8444707888363,
36.0659847749909));
#18699=CARTESIAN_POINT('Ctrl Pts',(-150.083777280819,-79.842719127427,36.0691506505178));
#18700=CARTESIAN_POINT('Ctrl Pts',(-150.124316972746,-79.7665150295156,
36.2068785740447));
#18701=CARTESIAN_POINT('Ctrl Pts',(-150.159836015384,-79.6996105779036,
36.3489635265334));
#18702=CARTESIAN_POINT('Ctrl Pts',(-150.189536570947,-79.6436016305276,
36.4961016996771));
#18703=CARTESIAN_POINT('Ctrl Pts',(-150.205994764959,-79.6125649679192,
36.5776364910029));
#18704=CARTESIAN_POINT('Ctrl Pts',(-150.220666659912,-79.5848732537881,
36.6607227768382));
#18705=CARTESIAN_POINT('Ctrl Pts',(-150.233419649245,-79.5607919801431,
36.7454773415068));
#18706=CARTESIAN_POINT('Ctrl Pts',(-150.233653158554,-79.5603510481059,
36.747029211371));
#18707=CARTESIAN_POINT('Ctrl Pts',(-150.233885994755,-79.5599113833124,
36.7485818022511));
#18708=CARTESIAN_POINT('Ctrl Pts',(-150.234118156878,-79.5594729876405,
36.7501351076896));
#18709=CARTESIAN_POINT('Ctrl Pts',(-150.243593980634,-79.541579629057,36.8135341168033));
#18710=CARTESIAN_POINT('Ctrl Pts',(-150.251930637624,-79.5258311439938,
36.8780113419661));
#18711=CARTESIAN_POINT('Ctrl Pts',(-150.25908694937,-79.5123085902626,36.9432880969467));
#18712=CARTESIAN_POINT('Ctrl Pts',(-150.266133192885,-79.49899402126,37.0075608575309));
#18713=CARTESIAN_POINT('Ctrl Pts',(-150.272035277523,-79.4878371314996,
37.0726101138059));
#18714=CARTESIAN_POINT('Ctrl Pts',(-150.276731655023,-79.4789572453977,
37.1381835195651));
#18715=CARTESIAN_POINT('Ctrl Pts',(-150.281154338818,-79.4705948579248,
37.1999354632931));
#18716=CARTESIAN_POINT('Ctrl Pts',(-150.284507727575,-79.4642518495709,
37.2621532653183));
#18717=CARTESIAN_POINT('Ctrl Pts',(-150.286719886614,-79.4600667280323,
37.3246214692037));
#18718=CARTESIAN_POINT('Ctrl Pts',(-150.28878458935,-79.4561605749315,37.3829257182099));
#18719=CARTESIAN_POINT('Ctrl Pts',(-150.289855072332,-79.4541343313065,
37.4414487162198));
#18720=CARTESIAN_POINT('Ctrl Pts',(-150.289855072464,-79.4541343310581,
37.5));
#18721=CARTESIAN_POINT('',(-150.289855072464,-79.4541343310581,44.5));
#18722=CARTESIAN_POINT('',(-150.289855072464,-79.4541343310581,115.));
#18723=CARTESIAN_POINT('',(-145.36231884058,-88.1464478086873,49.5));
#18724=CARTESIAN_POINT('Ctrl Pts',(-150.289855072464,-79.4541343310581,
44.5));
#18725=CARTESIAN_POINT('Ctrl Pts',(-150.289855068577,-79.4541343384106,
44.7563523801461));
#18726=CARTESIAN_POINT('Ctrl Pts',(-150.270581238553,-79.4906188049207,
45.0053815220034));
#18727=CARTESIAN_POINT('Ctrl Pts',(-150.23440031069,-79.5589401936918,45.2480116426047));
#18728=CARTESIAN_POINT('Ctrl Pts',(-150.233993766309,-79.5597078820386,
45.2507379384179));
#18729=CARTESIAN_POINT('Ctrl Pts',(-150.2335850823,-79.5604795994257,45.2534634549803));
#18730=CARTESIAN_POINT('Ctrl Pts',(-150.233174261933,-79.5612553394204,
45.2561881931872));
#18731=CARTESIAN_POINT('Ctrl Pts',(-150.211108362005,-79.6029217280976,
45.4025387770759));
#18732=CARTESIAN_POINT('Ctrl Pts',(-150.183223768725,-79.6555340186023,
45.5439666089425));
#18733=CARTESIAN_POINT('Ctrl Pts',(-150.1506572954,-79.7168744981717,45.6800320781738));
#18734=CARTESIAN_POINT('Ctrl Pts',(-150.129869982031,-79.7560283776325,
45.7668832247325));
#18735=CARTESIAN_POINT('Ctrl Pts',(-150.107175698374,-79.7987372958143,
45.8515497663918));
#18736=CARTESIAN_POINT('Ctrl Pts',(-150.082875014061,-79.8444151271613,
45.9339198071965));
#18737=CARTESIAN_POINT('Ctrl Pts',(-150.081600916097,-79.8468100404567,
45.9382385127928));
#18738=CARTESIAN_POINT('Ctrl Pts',(-150.080322360848,-79.8492131928944,
45.9425510499967));
#18739=CARTESIAN_POINT('Ctrl Pts',(-150.079039391808,-79.8516244996445,
45.94685739874));
#18740=CARTESIAN_POINT('Ctrl Pts',(-150.044542112121,-79.9164612343949,
46.0626492162668));
#18741=CARTESIAN_POINT('Ctrl Pts',(-150.006537123161,-79.9877842271942,
46.1748654509807));
#18742=CARTESIAN_POINT('Ctrl Pts',(-149.965970804575,-80.0637685565973,
46.2827346305569));
#18743=CARTESIAN_POINT('Ctrl Pts',(-149.933351576217,-80.1248672778719,
46.3694718432009));
#18744=CARTESIAN_POINT('Ctrl Pts',(-149.899077126141,-80.1889782570263,
46.4533984421142));
#18745=CARTESIAN_POINT('Ctrl Pts',(-149.863649966461,-80.2551332464111,
46.5341227219249));
#18746=CARTESIAN_POINT('Ctrl Pts',(-149.861515024356,-80.2591199355374,
46.5389873982183));
#18747=CARTESIAN_POINT('Ctrl Pts',(-149.85937578758,-80.2631142503699,46.5438407130638));
#18748=CARTESIAN_POINT('Ctrl Pts',(-149.857232364154,-80.2671159825673,
46.5486825816028));
#18749=CARTESIAN_POINT('Ctrl Pts',(-149.804252858279,-80.3660277477057,
46.6683601962307));
#18750=CARTESIAN_POINT('Ctrl Pts',(-149.748484158479,-80.4699094430547,
46.7819066280769));
#18751=CARTESIAN_POINT('Ctrl Pts',(-149.690355247898,-80.5778965450365,
46.8902500251402));
#18752=CARTESIAN_POINT('Ctrl Pts',(-149.661473306408,-80.6315510369212,
46.9440815458665));
#18753=CARTESIAN_POINT('Ctrl Pts',(-149.632008986731,-80.6862185045812,
46.9966292711324));
#18754=CARTESIAN_POINT('Ctrl Pts',(-149.60201639041,-80.741790230842,47.0480105076949));
#18755=CARTESIAN_POINT('Ctrl Pts',(-149.599223408299,-80.7469652025476,
47.0527952510041));
#18756=CARTESIAN_POINT('Ctrl Pts',(-149.596425806469,-80.7521480873936,
47.0575699305601));
#18757=CARTESIAN_POINT('Ctrl Pts',(-149.593623625112,-80.7573388040449,
47.0623346471253));
#18758=CARTESIAN_POINT('Ctrl Pts',(-149.503321107799,-80.9246137661054,
47.2158814184506));
#18759=CARTESIAN_POINT('Ctrl Pts',(-149.407759531995,-81.1009468141059,
47.3595995786781));
#18760=CARTESIAN_POINT('Ctrl Pts',(-149.309404815745,-81.2816192446479,
47.4931449450858));
#18761=CARTESIAN_POINT('Ctrl Pts',(-149.306147321137,-81.2876030905749,
47.4975679491626));
#18762=CARTESIAN_POINT('Ctrl Pts',(-149.302886794892,-81.2935916372183,
47.501979751875));
#18763=CARTESIAN_POINT('Ctrl Pts',(-149.299623326396,-81.2995847135535,
47.5063803428043));
#18764=CARTESIAN_POINT('Ctrl Pts',(-149.201294060241,-81.4801578671638,
47.6389714425028));
#18765=CARTESIAN_POINT('Ctrl Pts',(-149.100390942177,-81.6646756184357,
47.7614147349028));
#18766=CARTESIAN_POINT('Ctrl Pts',(-148.997297013874,-81.8523394986245,
47.8757113225169));
#18767=CARTESIAN_POINT('Ctrl Pts',(-148.993783486671,-81.8587352404397,
47.8796066457086));
#18768=CARTESIAN_POINT('Ctrl Pts',(-148.99026742009,-81.8651346268366,47.8834924864782));
#18769=CARTESIAN_POINT('Ctrl Pts',(-148.986748829868,-81.871537625153,47.8873689234621));
#18770=CARTESIAN_POINT('Ctrl Pts',(-148.828989572841,-82.1586219951734,
48.0611725720732));
#18771=CARTESIAN_POINT('Ctrl Pts',(-148.666197518726,-82.4528887104789,
48.2162655070009));
#18772=CARTESIAN_POINT('Ctrl Pts',(-148.499047675041,-82.7528397905676,
48.3561560144813));
#18773=CARTESIAN_POINT('Ctrl Pts',(-148.443888606593,-82.851822965143,48.4023195639484));
#18774=CARTESIAN_POINT('Ctrl Pts',(-148.388255039765,-82.9514250577883,
48.4468280100297));
#18775=CARTESIAN_POINT('Ctrl Pts',(-148.332171389768,-83.0515919680528,
48.4898085924912));
#18776=CARTESIAN_POINT('Ctrl Pts',(-148.328463625565,-83.0582141348388,
48.4926500955871));
#18777=CARTESIAN_POINT('Ctrl Pts',(-148.324753888106,-83.0648387811285,
48.4954849142925));
#18778=CARTESIAN_POINT('Ctrl Pts',(-148.321042184227,-83.0714658916725,
48.4983130852896));
#18779=CARTESIAN_POINT('Ctrl Pts',(-148.127526079489,-83.4169817679216,
48.6457646742983));
#18780=CARTESIAN_POINT('Ctrl Pts',(-147.928023779063,-83.7703038873281,
48.7751050652708));
#18781=CARTESIAN_POINT('Ctrl Pts',(-147.726117191241,-84.1248695147338,
48.8871259760477));
#18782=CARTESIAN_POINT('Ctrl Pts',(-147.691851026851,-84.1850438963965,
48.9061373762463));
#18783=CARTESIAN_POINT('Ctrl Pts',(-147.657515670427,-84.2452539899323,
48.9246499566981));
#18784=CARTESIAN_POINT('Ctrl Pts',(-147.623128700903,-84.3054675885421,
48.9426676169133));
#18785=CARTESIAN_POINT('Ctrl Pts',(-147.61966084937,-84.3115399997817,48.9444846589923));
#18786=CARTESIAN_POINT('Ctrl Pts',(-147.616192453019,-84.3176124815105,
48.9462966777585));
#18787=CARTESIAN_POINT('Ctrl Pts',(-147.612723530195,-84.3236850001122,
48.9481036768601));
#18788=CARTESIAN_POINT('Ctrl Pts',(-147.41439805748,-84.6708634135425,49.0514135425518));
#18789=CARTESIAN_POINT('Ctrl Pts',(-147.213653682834,-85.0194306321946,
49.1388789349076));
#18790=CARTESIAN_POINT('Ctrl Pts',(-147.010609976465,-85.3690841855301,
49.211977417735));
#18791=CARTESIAN_POINT('Ctrl Pts',(-146.970506380402,-85.4381450055664,
49.2264152551867));
#18792=CARTESIAN_POINT('Ctrl Pts',(-146.930313102763,-85.5072481940793,
49.2402927866165));
#18793=CARTESIAN_POINT('Ctrl Pts',(-146.89003109062,-85.5763914060563,49.253621628096));
#18794=CARTESIAN_POINT('Ctrl Pts',(-146.887290932544,-85.5810948287668,
49.254528314001));
#18795=CARTESIAN_POINT('Ctrl Pts',(-146.884550362083,-85.5857984397406,
49.2554324609279));
#18796=CARTESIAN_POINT('Ctrl Pts',(-146.881809379355,-85.5905022385503,
49.2563340725845));
#18797=CARTESIAN_POINT('Ctrl Pts',(-146.534412670951,-86.18666952076,49.3706058330548));
#18798=CARTESIAN_POINT('Ctrl Pts',(-146.180413916078,-86.7858240349752,
49.4448187829498));
#18799=CARTESIAN_POINT('Ctrl Pts',(-145.819603406779,-87.3878896744197,
49.4786922813549));
#18800=CARTESIAN_POINT('Ctrl Pts',(-145.668377265966,-87.6402328319036,
49.4928896461978));
#18801=CARTESIAN_POINT('Ctrl Pts',(-145.515954394526,-87.8930873961788,
49.4999999997319));
#18802=CARTESIAN_POINT('Ctrl Pts',(-145.36231884058,-88.1464478086873,49.5));
#18803=CARTESIAN_POINT('Origin',(0.,0.,49.5));
#18804=CARTESIAN_POINT('',(-119.689439203101,-120.724637681159,82.5));
#18805=CARTESIAN_POINT('',(-119.689439203101,-120.724637681159,115.));
#18806=CARTESIAN_POINT('',(-114.505594583524,-125.652173913043,87.5));
#18807=CARTESIAN_POINT('Ctrl Pts',(-114.505594583524,-125.652173913043,
87.5));
#18808=CARTESIAN_POINT('Ctrl Pts',(-114.875320870893,-125.315245971011,
87.4999999999648));
#18809=CARTESIAN_POINT('Ctrl Pts',(-115.240344827216,-124.979614114477,
87.4659613720207));
#18810=CARTESIAN_POINT('Ctrl Pts',(-115.600645981712,-124.645458541841,
87.3949999559647));
#18811=CARTESIAN_POINT('Ctrl Pts',(-115.815592858116,-124.446109481549,
87.3526661068053));
#18812=CARTESIAN_POINT('Ctrl Pts',(-116.028858884767,-124.247285605303,
87.2971925583144));
#18813=CARTESIAN_POINT('Ctrl Pts',(-116.240439697973,-124.049023288465,
87.2279752537405));
#18814=CARTESIAN_POINT('Ctrl Pts',(-116.245828883255,-124.043973339257,
87.2262122163769));
#18815=CARTESIAN_POINT('Ctrl Pts',(-116.251215926061,-124.038924730883,
87.2244403150215));
#18816=CARTESIAN_POINT('Ctrl Pts',(-116.25660079453,-124.033877495354,87.2226595463959));
#18817=CARTESIAN_POINT('Ctrl Pts',(-116.416321749011,-123.884171094794,
87.1698400455657));
#18818=CARTESIAN_POINT('Ctrl Pts',(-116.574127438346,-123.735675041936,
87.1092235235697));
#18819=CARTESIAN_POINT('Ctrl Pts',(-116.729307012311,-123.589109583791,
87.0406588491595));
#18820=CARTESIAN_POINT('Ctrl Pts',(-116.845631220869,-123.479242605265,
86.9892620623144));
#18821=CARTESIAN_POINT('Ctrl Pts',(-116.960479920838,-123.370460219089,
86.9333980875197));
#18822=CARTESIAN_POINT('Ctrl Pts',(-117.073550031386,-123.263067798316,
86.8729844025496));
#18823=CARTESIAN_POINT('Ctrl Pts',(-117.079344844513,-123.257563965281,
86.8698882172442));
#18824=CARTESIAN_POINT('Ctrl Pts',(-117.085135613102,-123.252063194138,
86.866779947454));
#18825=CARTESIAN_POINT('Ctrl Pts',(-117.090922329314,-123.24656549557,86.8636595351634));
#18826=CARTESIAN_POINT('Ctrl Pts',(-117.252833947861,-123.092740555707,
86.7763507773263));
#18827=CARTESIAN_POINT('Ctrl Pts',(-117.41152726411,-122.94136441611,86.6795632238393));
#18828=CARTESIAN_POINT('Ctrl Pts',(-117.56661345365,-122.792879292928,86.5721870844521));
#18829=CARTESIAN_POINT('Ctrl Pts',(-117.663683594914,-122.699940831253,
86.5049791850918));
#18830=CARTESIAN_POINT('Ctrl Pts',(-117.759340859086,-122.608134753002,
86.4336238696885));
#18831=CARTESIAN_POINT('Ctrl Pts',(-117.853493006743,-122.517566847009,
86.3578587588989));
#18832=CARTESIAN_POINT('Ctrl Pts',(-117.859134880481,-122.512139751579,
86.3533186905155));
#18833=CARTESIAN_POINT('Ctrl Pts',(-117.864772463519,-122.506716022107,
86.3487614273767));
#18834=CARTESIAN_POINT('Ctrl Pts',(-117.870405487109,-122.50129592327,86.3441871089973));
#18835=CARTESIAN_POINT('Ctrl Pts',(-117.971986956633,-122.403554169484,
86.2616974876393));
#18836=CARTESIAN_POINT('Ctrl Pts',(-118.07218659958,-122.306895851518,86.1735699087692));
#18837=CARTESIAN_POINT('Ctrl Pts',(-118.16934447046,-122.212953361598,86.0806804467646));
#18838=CARTESIAN_POINT('Ctrl Pts',(-118.186308138277,-122.196551096106,
86.0644620389012));
#18839=CARTESIAN_POINT('Ctrl Pts',(-118.203179139119,-122.180231567871,
86.0480985650011));
#18840=CARTESIAN_POINT('Ctrl Pts',(-118.219948731942,-122.164003379953,
86.0315948052611));
#18841=CARTESIAN_POINT('Ctrl Pts',(-118.225239204071,-122.158883710274,
86.0263881981678));
#18842=CARTESIAN_POINT('Ctrl Pts',(-118.2305200644,-122.153772676115,86.0211674735436));
#18843=CARTESIAN_POINT('Ctrl Pts',(-118.235791265575,-122.148670330441,
86.0159325934032));
#18844=CARTESIAN_POINT('Ctrl Pts',(-118.348386205055,-122.039682211169,
85.9041134855647));
#18845=CARTESIAN_POINT('Ctrl Pts',(-118.456626331103,-121.93460772812,85.7857889099975));
#18846=CARTESIAN_POINT('Ctrl Pts',(-118.560193282322,-121.833823583021,
85.6604137446068));
#18847=CARTESIAN_POINT('Ctrl Pts',(-118.564867100718,-121.829275348417,
85.6547557547994));
#18848=CARTESIAN_POINT('Ctrl Pts',(-118.569531415015,-121.824735838064,
85.649083428181));
#18849=CARTESIAN_POINT('Ctrl Pts',(-118.57418617698,-121.820205105343,85.6433966843365));
#18850=CARTESIAN_POINT('Ctrl Pts',(-118.656113089353,-121.7404611903,85.5433062031976));
#18851=CARTESIAN_POINT('Ctrl Pts',(-118.735109022985,-121.663408950081,
85.438709891701));
#18852=CARTESIAN_POINT('Ctrl Pts',(-118.81085074319,-121.589398131885,85.3292725022672));
#18853=CARTESIAN_POINT('Ctrl Pts',(-118.830778159308,-121.569926110818,
85.3004798581036));
#18854=CARTESIAN_POINT('Ctrl Pts',(-118.850480457644,-121.550664485438,
85.2713523136863));
#18855=CARTESIAN_POINT('Ctrl Pts',(-118.869952060987,-121.531619330202,
85.2418842081897));
#18856=CARTESIAN_POINT('Ctrl Pts',(-118.873852582751,-121.527804233869,
85.2359812024218));
#18857=CARTESIAN_POINT('Ctrl Pts',(-118.87774476105,-121.523996924348,85.2300626384257));
#18858=CARTESIAN_POINT('Ctrl Pts',(-118.881628379448,-121.520197619565,
85.2241287426542));
#18859=CARTESIAN_POINT('Ctrl Pts',(-118.953933356783,-121.449462388129,
85.1136518225954));
#18860=CARTESIAN_POINT('Ctrl Pts',(-119.023372190228,-121.381403002907,
84.9976861670382));
#18861=CARTESIAN_POINT('Ctrl Pts',(-119.088533293315,-121.317439625798,
84.8776565982512));
#18862=CARTESIAN_POINT('Ctrl Pts',(-119.107675671495,-121.298649103596,
84.8423955101238));
#18863=CARTESIAN_POINT('Ctrl Pts',(-119.126449080996,-121.280211875355,
84.8067838787667));
#18864=CARTESIAN_POINT('Ctrl Pts',(-119.144818331366,-121.262163368406,
84.7708581772729));
#18865=CARTESIAN_POINT('Ctrl Pts',(-119.147770180269,-121.259263061406,
84.7650850923405));
#18866=CARTESIAN_POINT('Ctrl Pts',(-119.150711776641,-121.256372617005,
84.7593040201353));
#18867=CARTESIAN_POINT('Ctrl Pts',(-119.153643085904,-121.253492073365,
84.7535149461629));
#18868=CARTESIAN_POINT('Ctrl Pts',(-119.217477211424,-121.190763453585,
84.6274482498874));
#18869=CARTESIAN_POINT('Ctrl Pts',(-119.276475877676,-121.132687812754,
84.497494707205));
#18870=CARTESIAN_POINT('Ctrl Pts',(-119.330291692485,-121.079649407418,
84.3634783756072));
#18871=CARTESIAN_POINT('Ctrl Pts',(-119.344664771969,-121.065483957758,
84.3276854141313));
#18872=CARTESIAN_POINT('Ctrl Pts',(-119.358668331276,-121.051677644484,
84.2916027835783));
#18873=CARTESIAN_POINT('Ctrl Pts',(-119.37229615525,-121.038237390605,84.2552274353945));
#18874=CARTESIAN_POINT('Ctrl Pts',(-119.374201887271,-121.036357888622,
84.2501406610181));
#18875=CARTESIAN_POINT('Ctrl Pts',(-119.376100550482,-121.034485269244,
84.2450470253995));
#18876=CARTESIAN_POINT('Ctrl Pts',(-119.377992089409,-121.032619589192,
84.2399466200188));
#18877=CARTESIAN_POINT('Ctrl Pts',(-119.432704267988,-120.978655370584,
84.0924189715063));
#18878=CARTESIAN_POINT('Ctrl Pts',(-119.481511542447,-120.930442075982,
83.9390510932854));
#18879=CARTESIAN_POINT('Ctrl Pts',(-119.523061427328,-120.889361770029,
83.7819751614297));
#18880=CARTESIAN_POINT('Ctrl Pts',(-119.53066769299,-120.88184146711,83.7532202979645));
#18881=CARTESIAN_POINT('Ctrl Pts',(-119.538030846413,-120.874560108483,
83.7243411856524));
#18882=CARTESIAN_POINT('Ctrl Pts',(-119.545142732111,-120.867526032261,
83.6953509136308));
#18883=CARTESIAN_POINT('Ctrl Pts',(-119.546090881023,-120.866588256825,
83.6914859619103));
#18884=CARTESIAN_POINT('Ctrl Pts',(-119.547034430282,-120.865655009876,
83.6876198631647));
#18885=CARTESIAN_POINT('Ctrl Pts',(-119.547973377994,-120.864726293782,
83.6837526181086));
#18886=CARTESIAN_POINT('Ctrl Pts',(-119.593937460371,-120.819263077397,
83.4944402974945));
#18887=CARTESIAN_POINT('Ctrl Pts',(-119.62890424618,-120.784628102355,83.3022686788512));
#18888=CARTESIAN_POINT('Ctrl Pts',(-119.65264519197,-120.761105073466,83.1071682749086));
#18889=CARTESIAN_POINT('Ctrl Pts',(-119.676892336666,-120.737080492046,
82.9079079856867));
#18890=CARTESIAN_POINT('Ctrl Pts',(-119.689439200918,-120.724637683323,
82.7055895150371));
#18891=CARTESIAN_POINT('Ctrl Pts',(-119.689439203101,-120.724637681159,
82.5));
#18892=CARTESIAN_POINT('',(-102.653719754201,-135.507246376812,87.5));
#18893=CARTESIAN_POINT('Origin',(0.,0.,87.5));
#18894=CARTESIAN_POINT('',(-95.8022538025509,-140.434782608696,82.5));
#18895=CARTESIAN_POINT('Ctrl Pts',(-102.653719754201,-135.507246376812,
87.5));
#18896=CARTESIAN_POINT('Ctrl Pts',(-102.215883490062,-135.838929901929,
87.4999999991685));
#18897=CARTESIAN_POINT('Ctrl Pts',(-101.781087350657,-136.164971110003,
87.4669218367414));
#18898=CARTESIAN_POINT('Ctrl Pts',(-101.349415497286,-136.485515662914,
87.4008783684644));
#18899=CARTESIAN_POINT('Ctrl Pts',(-101.07973591123,-136.68577037414,87.3596188444822));
#18900=CARTESIAN_POINT('Ctrl Pts',(-100.811275778686,-136.88387961001,87.3054922341186));
#18901=CARTESIAN_POINT('Ctrl Pts',(-100.544056427545,-137.079877141377,
87.2385159157322));
#18902=CARTESIAN_POINT('Ctrl Pts',(-100.541162556084,-137.081999710944,
87.2377905908054));
#18903=CARTESIAN_POINT('Ctrl Pts',(-100.538268831608,-137.084122031661,
87.2370637322218));
#18904=CARTESIAN_POINT('Ctrl Pts',(-100.535375254373,-137.086244103409,
87.2363353381554));
#18905=CARTESIAN_POINT('Ctrl Pts',(-100.190565643195,-137.339118201716,
87.1495371453096));
#18906=CARTESIAN_POINT('Ctrl Pts',(-99.8478512789412,-137.588453369916,
87.040933511602));
#18907=CARTESIAN_POINT('Ctrl Pts',(-99.5077977395583,-137.833951510589,
86.9074976668159));
#18908=CARTESIAN_POINT('Ctrl Pts',(-99.5037755731161,-137.836855272111,
86.9059193824726));
#18909=CARTESIAN_POINT('Ctrl Pts',(-99.4997536170413,-137.839758608548,
86.9043375053786));
#18910=CARTESIAN_POINT('Ctrl Pts',(-99.4957318889749,-137.842661507683,
86.9027520347699));
#18911=CARTESIAN_POINT('Ctrl Pts',(-99.2674376143156,-138.007445213001,
86.8127524483652));
#18912=CARTESIAN_POINT('Ctrl Pts',(-99.0398204570979,-138.170861151964,
86.711145683115));
#18913=CARTESIAN_POINT('Ctrl Pts',(-98.8161737755042,-138.33062666086,86.597820472154));
#18914=CARTESIAN_POINT('Ctrl Pts',(-98.7076262937751,-138.408169254089,
86.5428177948124));
#18915=CARTESIAN_POINT('Ctrl Pts',(-98.600013904115,-138.484852125992,86.4850552618045));
#18916=CARTESIAN_POINT('Ctrl Pts',(-98.4937108917853,-138.56041611792,86.4245237415767));
#18917=CARTESIAN_POINT('Ctrl Pts',(-98.4889708281906,-138.563785525046,
86.4218246341001));
#18918=CARTESIAN_POINT('Ctrl Pts',(-98.4842329483831,-138.56715301161,86.419119965262));
#18919=CARTESIAN_POINT('Ctrl Pts',(-98.479497264693,-138.570518570128,86.4164097092555));
#18920=CARTESIAN_POINT('Ctrl Pts',(-98.2490703748719,-138.73427849005,86.2845352212039));
#18921=CARTESIAN_POINT('Ctrl Pts',(-98.0238750005084,-138.8934512373,86.1394754931963));
#18922=CARTESIAN_POINT('Ctrl Pts',(-97.8050966305876,-139.047339894881,
85.9780962529129));
#18923=CARTESIAN_POINT('Ctrl Pts',(-97.7156206980972,-139.110277246236,
85.9120954045925));
#18924=CARTESIAN_POINT('Ctrl Pts',(-97.6272183327067,-139.172330541299,
85.8433644738521));
#18925=CARTESIAN_POINT('Ctrl Pts',(-97.5399718160535,-139.233451074562,
85.7716868356771));
#18926=CARTESIAN_POINT('Ctrl Pts',(-97.5352562713784,-139.236754548629,
85.7678127657659));
#18927=CARTESIAN_POINT('Ctrl Pts',(-97.5305452293931,-139.240054504138,
85.7639310032341));
#18928=CARTESIAN_POINT('Ctrl Pts',(-97.5258387376046,-139.243350910624,
85.7600415156019));
#18929=CARTESIAN_POINT('Ctrl Pts',(-97.3552183240805,-139.362852710079,
85.6190392536152));
#18930=CARTESIAN_POINT('Ctrl Pts',(-97.1907405919816,-139.47757645948,85.4680354210839));
#18931=CARTESIAN_POINT('Ctrl Pts',(-97.0346910654179,-139.586057153202,
85.3056163231383));
#18932=CARTESIAN_POINT('Ctrl Pts',(-96.9159928871056,-139.668572371353,
85.1820731668481));
#18933=CARTESIAN_POINT('Ctrl Pts',(-96.8021704778946,-139.747475893107,
85.0519259141839));
#18934=CARTESIAN_POINT('Ctrl Pts',(-96.694215926304,-139.822132033515,84.9145642707921));
#18935=CARTESIAN_POINT('Ctrl Pts',(-96.6906380099125,-139.824606347239,
84.9100117209624));
#18936=CARTESIAN_POINT('Ctrl Pts',(-96.6870657587802,-139.827076536154,
84.9054498746293));
#18937=CARTESIAN_POINT('Ctrl Pts',(-96.6834992847061,-139.82954252561,84.9008787661799));
#18938=CARTESIAN_POINT('Ctrl Pts',(-96.5933790288425,-139.891854937294,
84.7853726796454));
#18939=CARTESIAN_POINT('Ctrl Pts',(-96.5068951547278,-139.951522102754,
84.6638795752373));
#18940=CARTESIAN_POINT('Ctrl Pts',(-96.4259038292281,-140.007303114121,
84.5370163776214));
#18941=CARTESIAN_POINT('Ctrl Pts',(-96.3961160047755,-140.027818829404,
84.4903573232502));
#18942=CARTESIAN_POINT('Ctrl Pts',(-96.3670708290736,-140.047809094726,
84.4429721152884));
#18943=CARTESIAN_POINT('Ctrl Pts',(-96.3388592767016,-140.067213127358,
84.3948922769621));
#18944=CARTESIAN_POINT('Ctrl Pts',(-96.3362565453866,-140.069003297665,
84.390456544423));
#18945=CARTESIAN_POINT('Ctrl Pts',(-96.3336613068006,-140.070788207782,
84.3860158118469));
#18946=CARTESIAN_POINT('Ctrl Pts',(-96.3310735989047,-140.072567833443,
84.3815700581723));
#18947=CARTESIAN_POINT('Ctrl Pts',(-96.2565223686416,-140.123838412584,
84.2534889844106));
#18948=CARTESIAN_POINT('Ctrl Pts',(-96.18818677241,-140.170746863762,84.1211671345774));
#18949=CARTESIAN_POINT('Ctrl Pts',(-96.126962800212,-140.212720695597,83.9840977199587));
#18950=CARTESIAN_POINT('Ctrl Pts',(-96.1019843048262,-140.229845412064,
83.9281753807562));
#18951=CARTESIAN_POINT('Ctrl Pts',(-96.0781891189942,-140.246149048065,
83.8714630194104));
#18952=CARTESIAN_POINT('Ctrl Pts',(-96.0556361395659,-140.261594051371,
83.8139272219729));
#18953=CARTESIAN_POINT('Ctrl Pts',(-96.0542034790336,-140.262575183231,
83.8102723050498));
#18954=CARTESIAN_POINT('Ctrl Pts',(-96.0527757857576,-140.263552881361,
83.8066133446794));
#18955=CARTESIAN_POINT('Ctrl Pts',(-96.0513530943973,-140.264527122689,
83.802950400001));
#18956=CARTESIAN_POINT('Ctrl Pts',(-95.9866237488953,-140.308852972491,
83.6362944279056));
#18957=CARTESIAN_POINT('Ctrl Pts',(-95.9322125151014,-140.346047836819,
83.4612414093815));
#18958=CARTESIAN_POINT('Ctrl Pts',(-95.8913844101215,-140.373937837985,
83.2831693720156));
#18959=CARTESIAN_POINT('Ctrl Pts',(-95.883045620544,-140.379634131044,83.2467996886822));
#18960=CARTESIAN_POINT('Ctrl Pts',(-95.8752733682718,-140.384942326837,
83.2103039208797));
#18961=CARTESIAN_POINT('Ctrl Pts',(-95.8680953540231,-140.38984398165,83.1737276630787));
#18962=CARTESIAN_POINT('Ctrl Pts',(-95.8676809810245,-140.390126944783,
83.1716161858517));
#18963=CARTESIAN_POINT('Ctrl Pts',(-95.8672684958815,-140.390408616667,
83.1695042863138));
#18964=CARTESIAN_POINT('Ctrl Pts',(-95.8668579005401,-140.390688996011,
83.1673919642828));
#18965=CARTESIAN_POINT('Ctrl Pts',(-95.8468264218082,-140.404367701805,
83.0643393244232));
#18966=CARTESIAN_POINT('Ctrl Pts',(-95.8312774654238,-140.414980545424,
82.9601876791363));
#18967=CARTESIAN_POINT('Ctrl Pts',(-95.8204649814164,-140.422358778653,
82.855032721006));
#18968=CARTESIAN_POINT('Ctrl Pts',(-95.8099639220234,-140.429524501655,
82.7529064695304));
#18969=CARTESIAN_POINT('Ctrl Pts',(-95.8039305392802,-140.433639185389,
82.649833883227));
#18970=CARTESIAN_POINT('Ctrl Pts',(-95.8025570944415,-140.434575788992,
82.5459117712175));
#18971=CARTESIAN_POINT('Ctrl Pts',(-95.802355077537,-140.434713551904,82.5306261020837));
#18972=CARTESIAN_POINT('Ctrl Pts',(-95.8022538025544,-140.434782608693,
82.5153220699784));
#18973=CARTESIAN_POINT('Ctrl Pts',(-95.8022538025544,-140.434782608693,
82.5));
#18974=CARTESIAN_POINT('',(-95.8022538025509,-140.434782608696,-82.5));
#18975=CARTESIAN_POINT('',(-95.802253802551,-140.434782608696,115.));
#18976=CARTESIAN_POINT('',(-102.653719754201,-135.507246376812,-87.5));
#18977=CARTESIAN_POINT('Ctrl Pts',(-95.8022538025509,-140.434782608696,
-82.5));
#18978=CARTESIAN_POINT('Ctrl Pts',(-95.802253806658,-140.434782605894,-82.7267635628216));
#18979=CARTESIAN_POINT('Ctrl Pts',(-95.82442316008,-140.419665963906,-82.9488530674831));
#18980=CARTESIAN_POINT('Ctrl Pts',(-95.8667225776694,-140.39078140277,-83.1666939397165));
#18981=CARTESIAN_POINT('Ctrl Pts',(-95.8671957348732,-140.390458302857,
-83.1691306866946));
#18982=CARTESIAN_POINT('Ctrl Pts',(-95.8676714126208,-140.390133479021,
-83.1715669081132));
#18983=CARTESIAN_POINT('Ctrl Pts',(-95.8681496080969,-140.389806933124,
-83.1740026044675));
#18984=CARTESIAN_POINT('Ctrl Pts',(-95.9022176054039,-140.366542880454,
-83.347528497089));
#18985=CARTESIAN_POINT('Ctrl Pts',(-95.9496913058974,-140.334107437353,
-83.5193033103441));
#18986=CARTESIAN_POINT('Ctrl Pts',(-96.0075075764083,-140.294541978644,
-83.6842311536406));
#18987=CARTESIAN_POINT('Ctrl Pts',(-96.0214298424351,-140.285014542219,
-83.7239460866395));
#18988=CARTESIAN_POINT('Ctrl Pts',(-96.0359516723967,-140.275073772703,
-83.763263842758));
#18989=CARTESIAN_POINT('Ctrl Pts',(-96.0510300136253,-140.264748363786,
-83.8021130045776));
#18990=CARTESIAN_POINT('Ctrl Pts',(-96.0526816582041,-140.263617343775,
-83.8063684466409));
#18991=CARTESIAN_POINT('Ctrl Pts',(-96.0543400150297,-140.262481684736,
-83.8106183997866));
#18992=CARTESIAN_POINT('Ctrl Pts',(-96.0560050279566,-140.261341424076,
-83.8148627669174));
#18993=CARTESIAN_POINT('Ctrl Pts',(-96.1087379306465,-140.22522803811,-83.9492868277003));
#18994=CARTESIAN_POINT('Ctrl Pts',(-96.1682453864427,-140.18443183692,-84.0791983701216));
#18995=CARTESIAN_POINT('Ctrl Pts',(-96.2337564928184,-140.139445304685,
-84.2050184597015));
#18996=CARTESIAN_POINT('Ctrl Pts',(-96.2645815930236,-140.118277682266,
-84.2642208924444));
#18997=CARTESIAN_POINT('Ctrl Pts',(-96.2967352970674,-140.096182731474,
-84.3225177941468));
#18998=CARTESIAN_POINT('Ctrl Pts',(-96.3301343379528,-140.073213779952,
-84.379954552556));
#18999=CARTESIAN_POINT('Ctrl Pts',(-96.3331813229761,-140.071118329022,
-84.3851944917284));
#19000=CARTESIAN_POINT('Ctrl Pts',(-96.3362387534725,-140.069015548404,
-84.3904274269311));
#19001=CARTESIAN_POINT('Ctrl Pts',(-96.339306565948,-140.066905478751,-84.395653391359));
#19002=CARTESIAN_POINT('Ctrl Pts',(-96.4117861971074,-140.017053321434,
-84.519121164313));
#19003=CARTESIAN_POINT('Ctrl Pts',(-96.4899842015251,-139.963182743773,
-84.6383213996312));
#19004=CARTESIAN_POINT('Ctrl Pts',(-96.5721307818922,-139.90648063707,-84.7523713002298));
#19005=CARTESIAN_POINT('Ctrl Pts',(-96.6081754743616,-139.881600599589,
-84.8024146930877));
#19006=CARTESIAN_POINT('Ctrl Pts',(-96.6449798262798,-139.856175797233,
-84.8514667730734));
#19007=CARTESIAN_POINT('Ctrl Pts',(-96.6823922460858,-139.830307960496,
-84.8994546030547));
#19008=CARTESIAN_POINT('Ctrl Pts',(-96.6866911658693,-139.827335585128,
-84.9049687032585));
#19009=CARTESIAN_POINT('Ctrl Pts',(-96.6909982721163,-139.824357251049,
-84.9104689623343));
#19010=CARTESIAN_POINT('Ctrl Pts',(-96.6953133447443,-139.821373105703,
-84.9159552790218));
#19011=CARTESIAN_POINT('Ctrl Pts',(-96.8598715687415,-139.707570697129,
-85.1251796903365));
#19012=CARTESIAN_POINT('Ctrl Pts',(-97.0374177596496,-139.584350181588,
-85.3170893229325));
#19013=CARTESIAN_POINT('Ctrl Pts',(-97.2253643375751,-139.453317353096,
-85.4947229550121));
#19014=CARTESIAN_POINT('Ctrl Pts',(-97.32204057764,-139.385916492046,-85.5860944066665));
#19015=CARTESIAN_POINT('Ctrl Pts',(-97.4214682282139,-139.316448809721,
-85.6736891853026));
#19016=CARTESIAN_POINT('Ctrl Pts',(-97.5232920470755,-139.245134572953,
-85.757925116709));
#19017=CARTESIAN_POINT('Ctrl Pts',(-97.5293253469245,-139.240909037329,
-85.7629162930164));
#19018=CARTESIAN_POINT('Ctrl Pts',(-97.5353667088673,-139.236677264113,
-85.7678953452707));
#19019=CARTESIAN_POINT('Ctrl Pts',(-97.5414160595539,-139.232439298911,
-85.7728623680754));
#19020=CARTESIAN_POINT('Ctrl Pts',(-97.7162996213869,-139.109921943276,
-85.916456397384));
#19021=CARTESIAN_POINT('Ctrl Pts',(-97.895291385601,-138.984032327335,-86.0478104717196));
#19022=CARTESIAN_POINT('Ctrl Pts',(-98.0778068955091,-138.855116179076,
-86.1688889209447));
#19023=CARTESIAN_POINT('Ctrl Pts',(-98.2081021472136,-138.763084756681,
-86.2553251203982));
#19024=CARTESIAN_POINT('Ctrl Pts',(-98.3401938137772,-138.669510448868,
-86.3365230931734));
#19025=CARTESIAN_POINT('Ctrl Pts',(-98.473875270995,-138.57451383921,-86.4131838583186));
#19026=CARTESIAN_POINT('Ctrl Pts',(-98.4804799835183,-138.569820403706,
-86.4169713867174));
#19027=CARTESIAN_POINT('Ctrl Pts',(-98.4870884834129,-138.565123562489,
-86.4207477533706));
#19028=CARTESIAN_POINT('Ctrl Pts',(-98.4937007396705,-138.560423334432,
-86.4245130392829));
#19029=CARTESIAN_POINT('Ctrl Pts',(-98.7840182381348,-138.354055281161,
-86.589831554546));
#19030=CARTESIAN_POINT('Ctrl Pts',(-99.0816753104982,-138.141093446353,
-86.7335191028593));
#19031=CARTESIAN_POINT('Ctrl Pts',(-99.3855316162202,-137.922137712459,
-86.8583876011185));
#19032=CARTESIAN_POINT('Ctrl Pts',(-99.4178327914482,-137.898861817259,
-86.8716616361369));
#19033=CARTESIAN_POINT('Ctrl Pts',(-99.4502040159161,-137.875518191501,
-86.8847230529014));
#19034=CARTESIAN_POINT('Ctrl Pts',(-99.4826439161488,-137.852107558311,
-86.8975752625188));
#19035=CARTESIAN_POINT('Ctrl Pts',(-99.48920062357,-137.847375833759,-86.9001729332136));
#19036=CARTESIAN_POINT('Ctrl Pts',(-99.4957601913218,-137.842641332283,
-86.9027620700696));
#19037=CARTESIAN_POINT('Ctrl Pts',(-99.5023226100945,-137.83790405835,-86.9053427012605));
#19038=CARTESIAN_POINT('Ctrl Pts',(-99.7610782418026,-137.65111373735,-87.0070967765687));
#19039=CARTESIAN_POINT('Ctrl Pts',(-100.023540548839,-137.460524429142,
-87.0951230471669));
#19040=CARTESIAN_POINT('Ctrl Pts',(-100.286778083675,-137.268209582455,
-87.1698025082003));
#19041=CARTESIAN_POINT('Ctrl Pts',(-100.367689288363,-137.209097853065,
-87.1927567011173));
#19042=CARTESIAN_POINT('Ctrl Pts',(-100.448673514677,-137.149823232022,
-87.2144496897515));
#19043=CARTESIAN_POINT('Ctrl Pts',(-100.529644945651,-137.09044635394,-87.23489188421));
#19044=CARTESIAN_POINT('Ctrl Pts',(-100.535236887058,-137.08634574686,-87.2363036358892));
#19045=CARTESIAN_POINT('Ctrl Pts',(-100.54082877009,-137.082244650117,-87.237709423426));
#19046=CARTESIAN_POINT('Ctrl Pts',(-100.546420565381,-137.078143084482,
-87.2391092499));
#19047=CARTESIAN_POINT('Ctrl Pts',(-101.006759432587,-136.740485859902,
-87.3543485424286));
#19048=CARTESIAN_POINT('Ctrl Pts',(-101.469785375605,-136.39729021652,-87.4312211202132));
#19049=CARTESIAN_POINT('Ctrl Pts',(-101.935255327548,-136.048534047702,
-87.470101040684));
#19050=CARTESIAN_POINT('Ctrl Pts',(-102.174111258821,-135.869569800617,
-87.490052273998));
#19051=CARTESIAN_POINT('Ctrl Pts',(-102.413610624815,-135.689141411486,
-87.4999999996522));
#19052=CARTESIAN_POINT('Ctrl Pts',(-102.653719754201,-135.507246376812,
-87.5000000000001));
#19053=CARTESIAN_POINT('',(-114.505594583524,-125.652173913043,-87.5));
#19054=CARTESIAN_POINT('Origin',(0.,0.,-87.5));
#19055=CARTESIAN_POINT('',(-119.689439203101,-120.724637681159,-82.5));
#19056=CARTESIAN_POINT('Ctrl Pts',(-119.689439203101,-120.724637681159,
-82.5));
#19057=CARTESIAN_POINT('Ctrl Pts',(-119.689439202152,-120.7246376821,-82.7035326184388));
#19058=CARTESIAN_POINT('Ctrl Pts',(-119.677137855384,-120.736837058147,
-82.9047280297057));
#19059=CARTESIAN_POINT('Ctrl Pts',(-119.653068783703,-120.760685368386,
-83.1036884565072));
#19060=CARTESIAN_POINT('Ctrl Pts',(-119.653066214652,-120.760687913874,
-83.1037096928655));
#19061=CARTESIAN_POINT('Ctrl Pts',(-119.653063645461,-120.7606904595,-83.1037309292184));
#19062=CARTESIAN_POINT('Ctrl Pts',(-119.65306107613,-120.760693005266,-83.1037521655657));
#19063=CARTESIAN_POINT('Ctrl Pts',(-119.641919852122,-120.771732040813,
-83.1958379461839));
#19064=CARTESIAN_POINT('Ctrl Pts',(-119.628149514844,-120.785373482746,
-83.2877525621625));
#19065=CARTESIAN_POINT('Ctrl Pts',(-119.611957511397,-120.801406080513,
-83.3788351080295));
#19066=CARTESIAN_POINT('Ctrl Pts',(-119.594967539087,-120.818228791367,
-83.4744063532567));
#19067=CARTESIAN_POINT('Ctrl Pts',(-119.575311134826,-120.837684355012,
-83.5690634421961));
#19068=CARTESIAN_POINT('Ctrl Pts',(-119.553189137567,-120.859567147534,
-83.6620443506994));
#19069=CARTESIAN_POINT('Ctrl Pts',(-119.55083740086,-120.861893454956,-83.6719289290666));
#19070=CARTESIAN_POINT('Ctrl Pts',(-119.548457767033,-120.86424722548,-83.6817945487908));
#19071=CARTESIAN_POINT('Ctrl Pts',(-119.546050454752,-120.866628234349,
-83.6916402803605));
#19072=CARTESIAN_POINT('Ctrl Pts',(-119.545706019787,-120.866968905858,
-83.6930489942345));
#19073=CARTESIAN_POINT('Ctrl Pts',(-119.545361019709,-120.867310133486,
-83.6944572963284));
#19074=CARTESIAN_POINT('Ctrl Pts',(-119.545015455303,-120.867651916433,
-83.695865183348));
#19075=CARTESIAN_POINT('Ctrl Pts',(-119.498574793915,-120.913584384681,
-83.8850721826734));
#19076=CARTESIAN_POINT('Ctrl Pts',(-119.442053836954,-120.969435426432,
-84.0677448259361));
#19077=CARTESIAN_POINT('Ctrl Pts',(-119.376325844471,-121.034263033589,
-84.2444400249407));
#19078=CARTESIAN_POINT('Ctrl Pts',(-119.375341514619,-121.035233879443,
-84.2470861784687));
#19079=CARTESIAN_POINT('Ctrl Pts',(-119.374355124208,-121.036206734212,
-84.2497309822518));
#19080=CARTESIAN_POINT('Ctrl Pts',(-119.373366676025,-121.037181594878,
-84.2523744389033));
#19081=CARTESIAN_POINT('Ctrl Pts',(-119.316775771429,-121.092994583215,
-84.4037183391141));
#19082=CARTESIAN_POINT('Ctrl Pts',(-119.253023740241,-121.155791267692,
-84.5514088438984));
#19083=CARTESIAN_POINT('Ctrl Pts',(-119.183533814918,-121.224111669973,
-84.6934551425812));
#19084=CARTESIAN_POINT('Ctrl Pts',(-119.172587065958,-121.234874183951,
-84.7158316981047));
#19085=CARTESIAN_POINT('Ctrl Pts',(-119.161497891799,-121.245773805399,
-84.7380680949191));
#19086=CARTESIAN_POINT('Ctrl Pts',(-119.150271823512,-121.256804856299,
-84.7601564357346));
#19087=CARTESIAN_POINT('Ctrl Pts',(-119.148539861699,-121.25850673076,-84.7635642328206));
#19088=CARTESIAN_POINT('Ctrl Pts',(-119.146804666256,-121.260211709207,
-84.7669684593406));
#19089=CARTESIAN_POINT('Ctrl Pts',(-119.14506625839,-121.261919769914,-84.7703690853655));
#19090=CARTESIAN_POINT('Ctrl Pts',(-119.003325690235,-121.401185991481,
-85.0476381166482));
#19091=CARTESIAN_POINT('Ctrl Pts',(-118.842142596216,-121.559065359909,
-85.2991641553159));
#19092=CARTESIAN_POINT('Ctrl Pts',(-118.664609127849,-121.732125899566,
-85.5295567869234));
#19093=CARTESIAN_POINT('Ctrl Pts',(-118.633782041256,-121.762176302405,
-85.5695623907698));
#19094=CARTESIAN_POINT('Ctrl Pts',(-118.602462012018,-121.792684378039,
-85.6089309023198));
#19095=CARTESIAN_POINT('Ctrl Pts',(-118.570665287738,-121.82363207749,-85.6476865935965));
#19096=CARTESIAN_POINT('Ctrl Pts',(-118.567733597814,-121.826485486471,
-85.6512599072689));
#19097=CARTESIAN_POINT('Ctrl Pts',(-118.564797840986,-121.829342646821,
-85.6548280160802));
#19098=CARTESIAN_POINT('Ctrl Pts',(-118.561858031783,-121.832203542636,
-85.6583909367595));
#19099=CARTESIAN_POINT('Ctrl Pts',(-118.462775020542,-121.928626865597,
-85.778475229769));
#19100=CARTESIAN_POINT('Ctrl Pts',(-118.358568312162,-122.029796767798,
-85.8929376096802));
#19101=CARTESIAN_POINT('Ctrl Pts',(-118.251586150404,-122.133379331252,
-86.0001705886231));
#19102=CARTESIAN_POINT('Ctrl Pts',(-118.244181406579,-122.140548772723,
-86.0075926926972));
#19103=CARTESIAN_POINT('Ctrl Pts',(-118.236763379045,-122.147729760661,
-86.0149801731508));
#19104=CARTESIAN_POINT('Ctrl Pts',(-118.229332851436,-122.154921516527,
-86.0223325018978));
#19105=CARTESIAN_POINT('Ctrl Pts',(-118.226055490992,-122.158093562638,
-86.025575371406));
#19106=CARTESIAN_POINT('Ctrl Pts',(-118.222775639178,-122.161267761231,
-86.0288114700423));
#19107=CARTESIAN_POINT('Ctrl Pts',(-118.219493362288,-122.164444046394,
-86.0320407520766));
#19108=CARTESIAN_POINT('Ctrl Pts',(-118.104628229969,-122.27559993839,-86.1450512994916));
#19109=CARTESIAN_POINT('Ctrl Pts',(-117.986476048706,-122.389622505763,
-86.2501973510142));
#19110=CARTESIAN_POINT('Ctrl Pts',(-117.865390836685,-122.506120837556,
-86.3482582753084));
#19111=CARTESIAN_POINT('Ctrl Pts',(-117.861984025646,-122.509398593743,
-86.3510172830667));
#19112=CARTESIAN_POINT('Ctrl Pts',(-117.858574879434,-122.512678322681,
-86.3537706967463));
#19113=CARTESIAN_POINT('Ctrl Pts',(-117.855163404827,-122.515960016733,
-86.3565185352217));
#19114=CARTESIAN_POINT('Ctrl Pts',(-117.634786734593,-122.727953037703,
-86.5340252041163));
#19115=CARTESIAN_POINT('Ctrl Pts',(-117.404749948821,-122.948091205422,
-86.688414031018));
#19116=CARTESIAN_POINT('Ctrl Pts',(-117.165977845125,-123.175215067974,
-86.8223776503798));
#19117=CARTESIAN_POINT('Ctrl Pts',(-117.138194040773,-123.201643469212,
-86.837965815551));
#19118=CARTESIAN_POINT('Ctrl Pts',(-117.110291974294,-123.228166441777,
-86.8532774790446));
#19119=CARTESIAN_POINT('Ctrl Pts',(-117.082273113258,-123.25478214762,-86.8683169246712));
#19120=CARTESIAN_POINT('Ctrl Pts',(-117.079074540411,-123.257820539291,
-86.8700337954016));
#19121=CARTESIAN_POINT('Ctrl Pts',(-117.075874453949,-123.260860131433,
-86.8717471117034));
#19122=CARTESIAN_POINT('Ctrl Pts',(-117.072672856275,-123.263900921107,
-86.8734568798947));
#19123=CARTESIAN_POINT('Ctrl Pts',(-116.860769282127,-123.465161124843,
-86.9866210022035));
#19124=CARTESIAN_POINT('Ctrl Pts',(-116.644679584752,-123.669347667652,
-87.0827876682341));
#19125=CARTESIAN_POINT('Ctrl Pts',(-116.426318424243,-123.874581795949,
-87.1633254347002));
#19126=CARTESIAN_POINT('Ctrl Pts',(-116.366869236994,-123.930457126958,
-87.1852519748784));
#19127=CARTESIAN_POINT('Ctrl Pts',(-116.307251767595,-123.986410045268,
-87.2060203735688));
#19128=CARTESIAN_POINT('Ctrl Pts',(-116.247504799008,-124.042402536954,
-87.2256588635441));
#19129=CARTESIAN_POINT('Ctrl Pts',(-116.245124621172,-124.044633145315,
-87.2264412145098));
#19130=CARTESIAN_POINT('Ctrl Pts',(-116.242744233986,-124.046863820072,
-87.227221773433));
#19131=CARTESIAN_POINT('Ctrl Pts',(-116.24036363979,-124.049094558926,-87.228000542122));
#19132=CARTESIAN_POINT('Ctrl Pts',(-115.831177222972,-124.432523217204,
-87.3618585385571));
#19133=CARTESIAN_POINT('Ctrl Pts',(-115.413668066505,-124.8199443176,-87.4448575175416));
#19134=CARTESIAN_POINT('Ctrl Pts',(-114.988112144685,-125.210757527825,
-87.4801920420612));
#19135=CARTESIAN_POINT('Ctrl Pts',(-114.828401684543,-125.357429103603,
-87.4934530328749));
#19136=CARTESIAN_POINT('Ctrl Pts',(-114.667557747887,-125.504578468743,
-87.4999999998164));
#19137=CARTESIAN_POINT('Ctrl Pts',(-114.505594583524,-125.652173913044,
-87.5));
#19138=CARTESIAN_POINT('',(-119.689439203101,-120.724637681159,115.));
#19139=CARTESIAN_POINT('Origin',(-180.,-140.,85.));
#19140=CARTESIAN_POINT('',(-168.964466094067,-140.,-82.5));
#19141=CARTESIAN_POINT('',(-97.2111104761179,-140.,-82.5));
#19142=CARTESIAN_POINT('',(-180.,-140.,-82.5));
#19143=CARTESIAN_POINT('',(-97.2111104761179,-140.,82.5));
#19144=CARTESIAN_POINT('',(-97.2111104761179,-140.,85.));
#19145=CARTESIAN_POINT('',(-168.964466094067,-140.,82.5));
#19146=CARTESIAN_POINT('',(-170.,-140.,82.5));
#19147=CARTESIAN_POINT('',(-177.5,-140.,73.9644660940671));
#19148=CARTESIAN_POINT('',(-178.232233047034,-140.,73.2322330470335));
#19149=CARTESIAN_POINT('',(-177.5,-140.,-73.9644660940673));
#19150=CARTESIAN_POINT('',(-177.5,-140.,85.));
#19151=CARTESIAN_POINT('',(-168.232233047034,-140.,-83.2322330470337));
#19152=CARTESIAN_POINT('Origin',(-115.217186218029,-125.,85.));
#19153=CARTESIAN_POINT('',(-168.964466094067,-125.,-82.5));
#19154=CARTESIAN_POINT('',(-177.5,-125.,-73.9644660940673));
#19155=CARTESIAN_POINT('',(-178.232233047034,-125.,-73.2322330470336));
#19156=CARTESIAN_POINT('',(-177.5,-125.,73.9644660940672));
#19157=CARTESIAN_POINT('',(-177.5,-125.,85.));
#19158=CARTESIAN_POINT('',(-168.964466094067,-125.,82.5));
#19159=CARTESIAN_POINT('',(-168.232233047034,-125.,83.2322330470337));
#19160=CARTESIAN_POINT('',(-121.449578014911,-125.,82.5));
#19161=CARTESIAN_POINT('',(-115.217186218029,-125.,82.5));
#19162=CARTESIAN_POINT('',(-121.449578014911,-125.,47.));
#19163=CARTESIAN_POINT('',(-147.5,-125.,49.5));
#19164=CARTESIAN_POINT('',(-150.,-125.,49.5));
#19165=CARTESIAN_POINT('',(-152.5,-125.,44.5));
#19166=CARTESIAN_POINT('Origin',(-147.5,-125.,44.5));
#19167=CARTESIAN_POINT('',(-152.5,-125.,37.5));
#19168=CARTESIAN_POINT('',(-152.5,-125.,35.));
#19169=CARTESIAN_POINT('',(-147.5,-125.,32.5));
#19170=CARTESIAN_POINT('Origin',(-147.5,-125.,37.5));
#19171=CARTESIAN_POINT('',(-115.217186218029,-125.,32.5));
#19172=CARTESIAN_POINT('',(-121.449578014911,-125.,-35.));
#19173=CARTESIAN_POINT('',(-147.5,-125.,-32.5));
#19174=CARTESIAN_POINT('',(-115.217186218029,-125.,-32.5));
#19175=CARTESIAN_POINT('',(-152.5,-125.,-37.5));
#19176=CARTESIAN_POINT('Origin',(-147.5,-125.,-37.5));
#19177=CARTESIAN_POINT('',(-152.5,-125.,-44.5));
#19178=CARTESIAN_POINT('',(-152.5,-125.,85.));
#19179=CARTESIAN_POINT('',(-147.5,-125.,-49.5));
#19180=CARTESIAN_POINT('Origin',(-147.5,-125.,-44.5));
#19181=CARTESIAN_POINT('',(-115.217186218029,-125.,-49.5));
#19182=CARTESIAN_POINT('',(-121.449578014911,-125.,-82.5));
#19183=CARTESIAN_POINT('',(-121.449578014911,-125.,-85.));
#19184=CARTESIAN_POINT('',(-115.217186218029,-125.,-82.5));
#19185=CARTESIAN_POINT('Origin',(115.217186218029,-125.,85.));
#19186=CARTESIAN_POINT('',(147.5,-125.,49.5));
#19187=CARTESIAN_POINT('',(115.217186218029,-125.,49.5));
#19188=CARTESIAN_POINT('',(168.964466094067,-125.,82.5));
#19189=CARTESIAN_POINT('',(115.217186218029,-125.,82.5));
#19190=CARTESIAN_POINT('',(177.5,-125.,73.9644660940673));
#19191=CARTESIAN_POINT('',(140.840826156048,-125.,110.623639938019));
#19192=CARTESIAN_POINT('',(177.5,-125.,-73.9644660940672));
#19193=CARTESIAN_POINT('',(177.5,-125.,85.));
#19194=CARTESIAN_POINT('',(168.964466094067,-125.,-82.5));
#19195=CARTESIAN_POINT('',(225.840826156048,-125.,-25.623639938019));
#19196=CARTESIAN_POINT('',(115.217186218029,-125.,-82.5));
#19197=CARTESIAN_POINT('',(147.5,-125.,-49.5));
#19198=CARTESIAN_POINT('',(115.217186218029,-125.,-49.5));
#19199=CARTESIAN_POINT('',(152.5,-125.,-44.5));
#19200=CARTESIAN_POINT('Origin',(147.5,-125.,-44.5));
#19201=CARTESIAN_POINT('',(152.5,-125.,-37.5));
#19202=CARTESIAN_POINT('',(152.5,-125.,85.));
#19203=CARTESIAN_POINT('',(147.5,-125.,-32.5));
#19204=CARTESIAN_POINT('Origin',(147.5,-125.,-37.5));
#19205=CARTESIAN_POINT('',(115.217186218029,-125.,-32.5));
#19206=CARTESIAN_POINT('',(147.5,-125.,32.5));
#19207=CARTESIAN_POINT('',(150.,-125.,32.5));
#19208=CARTESIAN_POINT('',(152.5,-125.,37.5));
#19209=CARTESIAN_POINT('Origin',(147.5,-125.,37.5));
#19210=CARTESIAN_POINT('',(152.5,-125.,44.5));
#19211=CARTESIAN_POINT('',(152.5,-125.,47.));
#19212=CARTESIAN_POINT('Origin',(147.5,-125.,44.5));
#19213=CARTESIAN_POINT('Origin',(0.,0.,-105.));
#19214=CARTESIAN_POINT('Origin',(-115.,0.,-105.));
#19215=CARTESIAN_POINT('',(-96.695242233189,174.040040919032,-44.9999999999999));
#19216=CARTESIAN_POINT('Origin',(-115.,0.,-44.9999999999999));
#19217=CARTESIAN_POINT('',(-96.695242233189,174.040040919032,45.0000000000001));
#19218=CARTESIAN_POINT('Origin',(-115.,0.,45.0000000000001));
#19219=CARTESIAN_POINT('',(-96.695242233189,174.040040919032,-105.));
#19220=CARTESIAN_POINT('Origin',(-115.000000000001,175.,80.0000000000001));
#19221=CARTESIAN_POINT('',(-93.0342906798268,208.848049102839,80.0000000000001));
#19222=CARTESIAN_POINT('',(-14.5652173913043,184.425742352699,80.));
#19223=CARTESIAN_POINT('Origin',(-115.,0.,80.0000000000001));
#19224=CARTESIAN_POINT('',(65.4347826086958,173.041293409847,80.));
#19225=CARTESIAN_POINT('Origin',(-3.78485122031303E-15,0.,80.));
#19226=CARTESIAN_POINT('',(-108.033967922038,249.902929948988,80.0000000000001));
#19227=CARTESIAN_POINT('Origin',(-115.,0.,80.0000000000001));
#19228=CARTESIAN_POINT('',(-108.033967922038,209.585728186396,80.0000000000001));
#19229=CARTESIAN_POINT('',(-108.033967922038,175.,80.0000000000001));
#19230=CARTESIAN_POINT('Origin',(-107.155103814224,74.5885889652995,80.0000000000001));
#19231=CARTESIAN_POINT('Origin',(-115.,0.,-105.));
#19232=CARTESIAN_POINT('',(-107.058723431124,284.889340141846,-44.9999999999999));
#19233=CARTESIAN_POINT('Origin',(-115.,0.,-44.9999999999999));
#19234=CARTESIAN_POINT('',(-115.000000000001,285.,-45.1798442476466));
#19235=CARTESIAN_POINT('Origin',(-109.23990359688,206.681571026642,-172.26199221829));
#19236=CARTESIAN_POINT('',(-115.000000000001,285.,45.1798442476468));
#19237=CARTESIAN_POINT('',(-115.000000000001,285.,2.44375389117379E-28));
#19238=CARTESIAN_POINT('',(-107.058723431124,284.889340141846,45.0000000000001));
#19239=CARTESIAN_POINT('Origin',(-109.239903596884,206.681571026862,172.261992218181));
#19240=CARTESIAN_POINT('Origin',(-115.,0.,45.0000000000001));
#19241=CARTESIAN_POINT('Origin',(-115.000000000001,175.,-79.9999999999999));
#19242=CARTESIAN_POINT('',(-108.033967922038,249.902929948988,-79.9999999999999));
#19243=CARTESIAN_POINT('',(65.4347826086956,173.041293409847,-80.));
#19244=CARTESIAN_POINT('Origin',(-115.,0.,-79.9999999999999));
#19245=CARTESIAN_POINT('',(-14.5652173913044,184.425742352699,-80.));
#19246=CARTESIAN_POINT('Origin',(3.78485122031304E-15,0.,-80.));
#19247=CARTESIAN_POINT('',(-93.0342906798268,208.848049102839,-79.9999999999999));
#19248=CARTESIAN_POINT('Origin',(-115.,0.,-79.9999999999999));
#19249=CARTESIAN_POINT('',(-108.033967922038,209.585728186396,-79.9999999999999));
#19250=CARTESIAN_POINT('Origin',(-107.155103814224,74.5885889652995,-79.9999999999999));
#19251=CARTESIAN_POINT('',(-108.033967922039,285.,-79.9999999999999));
#19252=CARTESIAN_POINT('Origin',(-365.,-1.26634813746307E-12,8.80937834756918E-14));
#19253=CARTESIAN_POINT('',(-365.000000000001,249.999999999999,-115.));
#19254=CARTESIAN_POINT('',(-365.000000000001,159.722601683408,-115.));
#19255=CARTESIAN_POINT('',(-365.000000000001,284.999999999999,-115.));
#19256=CARTESIAN_POINT('',(-365.000000000001,124.999999999999,-80.6196334903569));
#19257=CARTESIAN_POINT('Origin',(-365.000000000001,160.693136595148,-79.658664428181));
#19258=CARTESIAN_POINT('',(-365.000000000001,124.999999999999,80.6196334903571));
#19259=CARTESIAN_POINT('',(-365.000000000001,124.999999999999,-115.));
#19260=CARTESIAN_POINT('',(-365.000000000001,159.722601683408,115.));
#19261=CARTESIAN_POINT('Origin',(-365.000000000001,160.693136595149,79.6586644281792));
#19262=CARTESIAN_POINT('',(-365.000000000001,249.999999999999,115.));
#19263=CARTESIAN_POINT('',(-365.000000000001,284.999999999999,115.));
#19264=CARTESIAN_POINT('',(-365.000000000001,284.999999999999,79.65866442818));
#19265=CARTESIAN_POINT('Origin',(-365.000000000001,249.999999999999,79.6586644281791));
#19266=CARTESIAN_POINT('',(-365.000000000001,284.999999999999,-79.6586644281798));
#19267=CARTESIAN_POINT('',(-365.000000000001,284.999999999999,-115.));
#19268=CARTESIAN_POINT('Origin',(-365.000000000001,250.,-79.6586644281799));
#19269=CARTESIAN_POINT('',(-365.000000000001,249.999999999999,-104.902475550908));
#19270=CARTESIAN_POINT('',(-365.000000000001,159.999897372477,-104.902475550908));
#19271=CARTESIAN_POINT('',(-365.,-1.26634813746307E-12,-104.902475550908));
#19272=CARTESIAN_POINT('',(-365.000000000001,274.999999999999,-79.6586644281798));
#19273=CARTESIAN_POINT('Origin',(-365.000000000001,249.999999999997,-79.6586644281774));
#19274=CARTESIAN_POINT('',(-365.000000000001,274.999999999999,79.65866442818));
#19275=CARTESIAN_POINT('',(-365.000000000001,274.999999999999,8.8093783475692E-14));
#19276=CARTESIAN_POINT('',(-365.000000000001,250.,104.902475550909));
#19277=CARTESIAN_POINT('Origin',(-365.000000000001,249.999999999998,79.6586644281787));
#19278=CARTESIAN_POINT('',(-365.000000000001,159.999897372477,104.902475550909));
#19279=CARTESIAN_POINT('',(-365.,-1.26634813746307E-12,104.902475550909));
#19280=CARTESIAN_POINT('',(-365.000000000001,135.198039027185,80.3450709011636));
#19281=CARTESIAN_POINT('Origin',(-365.000000000001,160.693136595147,79.6586644281815));
#19282=CARTESIAN_POINT('',(-365.000000000001,135.198039027185,-80.3450709011634));
#19283=CARTESIAN_POINT('',(-365.000000000001,135.198039027185,8.80937834756919E-14));
#19284=CARTESIAN_POINT('Origin',(-365.,160.693136595149,-79.6586644281788));
#19285=CARTESIAN_POINT('Origin',(-1.01252339845814E-12,285.,2.44375389117379E-28));
#19286=CARTESIAN_POINT('',(-126.751426934183,285.,-46.3038641989653));
#19287=CARTESIAN_POINT('Origin',(-108.033967922039,285.,-180.));
#19288=CARTESIAN_POINT('',(3.92135447228731,285.,-28.0096748020595));
#19289=CARTESIAN_POINT('',(-126.751426934183,285.,46.3038641989655));
#19290=CARTESIAN_POINT('',(3.92135447228733,285.,28.0096748020595));
#19291=CARTESIAN_POINT('Origin',(-108.033967922038,285.,180.));
#19292=CARTESIAN_POINT('Origin',(8.77402903099257,3.04410282779297E-14,
62.6716359356611));
#19293=CARTESIAN_POINT('',(-128.778107499175,206.966980183574,81.9289350498845));
#19294=CARTESIAN_POINT('',(-35.4836922769749,225.625863228014,68.8677169187765));
#19295=CARTESIAN_POINT('',(-121.898752375479,208.15873578029,80.965825332567));
#19296=CARTESIAN_POINT('Origin',(-102.313983178497,72.0502950009906,78.2239576449902));
#19297=CARTESIAN_POINT('',(-121.898752375479,250.,80.965825332567));
#19298=CARTESIAN_POINT('',(-121.898752375479,285.,80.965825332567));
#19299=CARTESIAN_POINT('',(8.77402903099168,250.,62.6716359356611));
#19300=CARTESIAN_POINT('Origin',(8.77402903099253,3.04410282779296E-14,
-62.671635935661));
#19301=CARTESIAN_POINT('',(-121.898752375479,250.,-80.9658253325669));
#19302=CARTESIAN_POINT('',(-121.898752375479,208.15873578029,-80.9658253325669));
#19303=CARTESIAN_POINT('',(-121.898752375479,175.,-80.9658253325669));
#19304=CARTESIAN_POINT('',(-128.778107499175,206.966980183574,-81.9289350498844));
#19305=CARTESIAN_POINT('Origin',(-102.313983154048,72.050294857119,-78.2239576415826));
#19306=CARTESIAN_POINT('',(-35.4836922769749,225.625863228014,-68.8677169187764));
#19307=CARTESIAN_POINT('',(8.77402903099165,250.,-62.671635935661));
#19308=CARTESIAN_POINT('Origin',(-38.0769230769238,190.384615384616,9.1899731971482E-15));
#19309=CARTESIAN_POINT('',(-126.766717328043,172.646656534391,-47.2669739162828));
#19310=CARTESIAN_POINT('',(-33.4723021058426,191.305539578832,-34.2057557851748));
#19311=CARTESIAN_POINT('',(-126.766717328043,172.646656534391,47.2669739162829));
#19312=CARTESIAN_POINT('',(-126.766717328043,172.646656534391,80.));
#19313=CARTESIAN_POINT('',(-33.4723021058425,191.305539578832,34.2057557851749));
#19314=CARTESIAN_POINT('Origin',(-108.033967922037,-3.74818120714568E-13,
180.));
#19315=CARTESIAN_POINT('Ctrl Pts',(-121.898752375479,208.15873578029,80.965825332567));
#19316=CARTESIAN_POINT('Ctrl Pts',(-119.963682399492,208.541997665569,80.6949155359288));
#19317=CARTESIAN_POINT('Ctrl Pts',(-118.016904254303,208.849389003878,80.4801212165123));
#19318=CARTESIAN_POINT('Ctrl Pts',(-116.058201668433,209.079632070727,80.3224566800619));
#19319=CARTESIAN_POINT('Ctrl Pts',(-115.706309545742,209.120996554602,80.294131344299));
#19320=CARTESIAN_POINT('Ctrl Pts',(-115.35403253681,209.159870880317,80.2676500224512));
#19321=CARTESIAN_POINT('Ctrl Pts',(-115.001369373232,209.19624749802,80.2430187053663));
#19322=CARTESIAN_POINT('Ctrl Pts',(-113.243049246847,209.37761528928,80.12021103776));
#19323=CARTESIAN_POINT('Ctrl Pts',(-111.475122526152,209.496902484032,80.0433849490804));
#19324=CARTESIAN_POINT('Ctrl Pts',(-109.697347830952,209.55244226832,80.0138248285002));
#19325=CARTESIAN_POINT('Ctrl Pts',(-109.143844976527,209.569734352194,80.004621406288));
#19326=CARTESIAN_POINT('Ctrl Pts',(-108.589387464291,209.580846699948,80.0000000000001));
#19327=CARTESIAN_POINT('Ctrl Pts',(-108.033967922038,209.585728186396,80.0000000000001));
#19328=CARTESIAN_POINT('',(-113.193991683492,250.,80.1332179612198));
#19329=CARTESIAN_POINT('Origin',(-109.82357655303,202.360240296963,145.359472475069));
#19330=CARTESIAN_POINT('Origin',(-108.033967922038,250.,180.));
#19331=CARTESIAN_POINT('Origin',(-107.155103814224,74.5885889652995,-105.));
#19332=CARTESIAN_POINT('',(-121.670898717897,173.529438457885,-46.3038641989653));
#19333=CARTESIAN_POINT('',(-107.806114264457,174.586469869815,-44.9999999999999));
#19334=CARTESIAN_POINT('Ctrl Pts',(-121.670898717897,173.529438457885,-46.3038641989653));
#19335=CARTESIAN_POINT('Ctrl Pts',(-119.700296307634,173.818549179804,-45.9314203435801));
#19336=CARTESIAN_POINT('Ctrl Pts',(-117.717862072481,174.049330964995,-45.6375988479542));
#19337=CARTESIAN_POINT('Ctrl Pts',(-115.723382153899,174.220839876011,-45.4237707689551));
#19338=CARTESIAN_POINT('Ctrl Pts',(-115.407063289645,174.248040703373,-45.3898582414514));
#19339=CARTESIAN_POINT('Ctrl Pts',(-115.090441431131,174.273750575165,-45.3579578799593));
#19340=CARTESIAN_POINT('Ctrl Pts',(-114.773515715655,174.297965656261,-45.3280752522696));
#19341=CARTESIAN_POINT('Ctrl Pts',(-112.980668894128,174.434950220962,-45.1590294113797));
#19342=CARTESIAN_POINT('Ctrl Pts',(-111.178090500797,174.524105770559,-45.0545447965882));
#19343=CARTESIAN_POINT('Ctrl Pts',(-109.365535898701,174.564165311637,-45.0164029276363));
#19344=CARTESIAN_POINT('Ctrl Pts',(-108.846548544408,174.575635528984,-45.0054817958634));
#19345=CARTESIAN_POINT('Ctrl Pts',(-108.326743269188,174.583080448762,-44.9999999999999));
#19346=CARTESIAN_POINT('Ctrl Pts',(-107.806114264457,174.586469869815,-44.9999999999999));
#19347=CARTESIAN_POINT('Origin',(-107.155103814224,74.5885889652995,-44.9999999999999));
#19348=CARTESIAN_POINT('',(-107.806114264457,174.586469869815,45.0000000000001));
#19349=CARTESIAN_POINT('Origin',(-107.155103814224,74.5885889652995,45.0000000000001));
#19350=CARTESIAN_POINT('',(-121.670898717897,173.529438457885,46.3038641989655));
#19351=CARTESIAN_POINT('Ctrl Pts',(-107.806114264457,174.586469869815,45.));
#19352=CARTESIAN_POINT('Ctrl Pts',(-109.624402314666,174.574632373745,45.));
#19353=CARTESIAN_POINT('Ctrl Pts',(-111.432643308778,174.51333051059,45.0668606225803));
#19354=CARTESIAN_POINT('Ctrl Pts',(-113.231083127889,174.403839947209,45.1987882647131));
#19355=CARTESIAN_POINT('Ctrl Pts',(-113.74602899258,174.37248959996,45.2365630031463));
#19356=CARTESIAN_POINT('Ctrl Pts',(-114.260171286305,174.337188339623,45.2796724887734));
#19357=CARTESIAN_POINT('Ctrl Pts',(-114.773515715654,174.297965656261,45.3280752522816));
#19358=CARTESIAN_POINT('Ctrl Pts',(-116.77182207048,174.145282714882,45.5164936793255));
#19359=CARTESIAN_POINT('Ctrl Pts',(-118.758048443814,173.933174431027,45.785126873589));
#19360=CARTESIAN_POINT('Ctrl Pts',(-120.732409349687,173.662589501794,46.1325970502785));
#19361=CARTESIAN_POINT('Ctrl Pts',(-121.045537318146,173.619675509253,46.1877048222179));
#19362=CARTESIAN_POINT('Ctrl Pts',(-121.358366825477,173.575290589482,46.2447956712981));
#19363=CARTESIAN_POINT('Ctrl Pts',(-121.670898717897,173.529438457885,46.3038641989655));
#19364=CARTESIAN_POINT('Origin',(-107.172158244333,71.1720523181789,43.5636022494356));
#19365=CARTESIAN_POINT('Origin',(-107.172158244267,71.1720523177554,-43.5636022494229));
#19366=CARTESIAN_POINT('Origin',(-108.033967922038,-3.74818120714567E-13,
-180.));
#19367=CARTESIAN_POINT('Ctrl Pts',(-108.033967922038,209.585728186396,-79.9999999999999));
#19368=CARTESIAN_POINT('Ctrl Pts',(-109.817898725999,209.570049526606,-79.9999999999999));
#19369=CARTESIAN_POINT('Ctrl Pts',(-111.591905506614,209.490096075732,-80.0476722982013));
#19370=CARTESIAN_POINT('Ctrl Pts',(-113.356231010759,209.347547495565,-80.1417226834948));
#19371=CARTESIAN_POINT('Ctrl Pts',(-113.905546550713,209.303165577319,-80.1710048868405));
#19372=CARTESIAN_POINT('Ctrl Pts',(-114.453923591632,209.252715618219,-80.204783040216));
#19373=CARTESIAN_POINT('Ctrl Pts',(-115.001369373232,209.19624749802,-80.2430187053662));
#19374=CARTESIAN_POINT('Ctrl Pts',(-116.964363679643,208.993767906125,-80.3801215848005));
#19375=CARTESIAN_POINT('Ctrl Pts',(-118.915394248576,208.713906143843,-80.574539846874));
#19376=CARTESIAN_POINT('Ctrl Pts',(-120.85467810225,208.357947311172,-80.8252534637792));
#19377=CARTESIAN_POINT('Ctrl Pts',(-121.203081595339,208.293997260506,-80.8702956063874));
#19378=CARTESIAN_POINT('Ctrl Pts',(-121.551105938358,208.227590979612,-80.9171548313701));
#19379=CARTESIAN_POINT('Ctrl Pts',(-121.898752375479,208.15873578029,-80.9658253325669));
#19380=CARTESIAN_POINT('',(-113.193991683492,250.,-80.1332179612197));
#19381=CARTESIAN_POINT('Origin',(-108.033967922038,250.,-180.));
#19382=CARTESIAN_POINT('Origin',(-109.823576553026,202.360240296967,-145.359472475138));
#19383=CARTESIAN_POINT('Origin',(-40.3363668356791,225.625863228014,-34.2057557851748));
#19384=CARTESIAN_POINT('Origin',(-133.630782057879,206.966980183574,-47.2669739162828));
#19385=CARTESIAN_POINT('Ctrl Pts',(-121.670898717897,173.529438457885,-46.3038641989654));
#19386=CARTESIAN_POINT('Ctrl Pts',(-117.014194117273,174.212632196936,-80.2819871764181));
#19387=CARTESIAN_POINT('Ctrl Pts',(-121.898752375479,208.15873578029,-80.9658253325669));
#19388=CARTESIAN_POINT('Ctrl Pts',(-123.376736606944,173.279171828244,-46.6262675599635));
#19389=CARTESIAN_POINT('Ctrl Pts',(-118.752370779928,174.039540392877,-80.5253319092667));
#19390=CARTESIAN_POINT('Ctrl Pts',(-124.201633525808,207.820875830255,-81.288228693613));
#19391=CARTESIAN_POINT('Ctrl Pts',(-125.076099494733,172.984780101053,-46.9474471457602));
#19392=CARTESIAN_POINT('Ctrl Pts',(-120.48990998314,173.820474755941,-80.7685873976411));
#19393=CARTESIAN_POINT('Ctrl Pts',(-126.495773409627,207.423447001444,-81.6094082773477));
#19394=CARTESIAN_POINT('Ctrl Pts',(-126.766717328043,172.646656534391,-47.2669739162828));
#19395=CARTESIAN_POINT('Ctrl Pts',(-122.224200046663,173.555159990667,-81.0113880065327));
#19396=CARTESIAN_POINT('Ctrl Pts',(-128.778107499175,206.966980183574,-81.9289350498844));
#19397=CARTESIAN_POINT('Origin',(-126.751426934183,208.15873578029,-46.3038641989653));
#19398=CARTESIAN_POINT('Ctrl Pts',(-107.806114264457,174.586469869815,-44.9999999999999));
#19399=CARTESIAN_POINT('Ctrl Pts',(-107.806114264457,174.586469869815,-79.9999999999999));
#19400=CARTESIAN_POINT('Ctrl Pts',(-108.033967922038,209.585728186396,-79.9999999999999));
#19401=CARTESIAN_POINT('Ctrl Pts',(-110.140392035471,174.571273155555,-44.9999999999671));
#19402=CARTESIAN_POINT('Ctrl Pts',(-109.323233110512,174.576593058387,-79.9946819508194));
#19403=CARTESIAN_POINT('Ctrl Pts',(-110.368245901835,209.565212620414,-79.9999999999999));
#19404=CARTESIAN_POINT('Ctrl Pts',(-112.462776734628,174.47452037898,-45.1101978466298));
#19405=CARTESIAN_POINT('Ctrl Pts',(-110.831769330981,174.542829711498,-80.0133399190488));
#19406=CARTESIAN_POINT('Ctrl Pts',(-112.690630392213,209.434596373781,-80.0816280345504));
#19407=CARTESIAN_POINT('Ctrl Pts',(-117.084254696684,174.121410933542,-45.5459526578601));
#19408=CARTESIAN_POINT('Ctrl Pts',(-113.886869252213,174.421832152824,-80.1038421118365));
#19409=CARTESIAN_POINT('Ctrl Pts',(-117.312108354263,208.957898622415,-80.4044093761828));
#19410=CARTESIAN_POINT('Ctrl Pts',(-119.383361285263,173.865047302734,-45.8715196243769));
#19411=CARTESIAN_POINT('Ctrl Pts',(-115.428565673966,174.334921360029,-80.1754126412373));
#19412=CARTESIAN_POINT('Ctrl Pts',(-119.611215134969,208.611807682755,-80.6455701188955));
#19413=CARTESIAN_POINT('Ctrl Pts',(-121.670898717897,173.529438457885,-46.3038641989653));
#19414=CARTESIAN_POINT('Ctrl Pts',(-117.014194117273,174.212632196936,-80.2819871764181));
#19415=CARTESIAN_POINT('Ctrl Pts',(-121.898752375479,208.15873578029,-80.9658253325669));
#19416=CARTESIAN_POINT('Origin',(-108.033967922038,209.585728186396,-44.9999999999999));
#19417=CARTESIAN_POINT('Origin',(-107.155103814224,74.5885889652995,-44.9999999999999));
#19418=CARTESIAN_POINT('Origin',(-93.0342906798268,208.848049102839,-44.9999999999999));
#19419=CARTESIAN_POINT('Origin',(-115.,0.,-44.9999999999999));
#19420=CARTESIAN_POINT('Ctrl Pts',(-14.5652173913044,184.425742352699,-80.));
#19421=CARTESIAN_POINT('Ctrl Pts',(-16.5344677033485,184.565305142146,-80.));
#19422=CARTESIAN_POINT('Ctrl Pts',(-18.5002973477175,184.673702607589,-79.9714170458664));
#19423=CARTESIAN_POINT('Ctrl Pts',(-20.462612886933,184.751448877997,-79.9131822068492));
#19424=CARTESIAN_POINT('Ctrl Pts',(-22.3952938122587,184.82802103514,-79.8558268221983));
#19425=CARTESIAN_POINT('Ctrl Pts',(-24.324565992262,184.87486103494,-79.7697082616294));
#19426=CARTESIAN_POINT('Ctrl Pts',(-26.2503475316718,184.892497907978,-79.6538362317921));
#19427=CARTESIAN_POINT('Ctrl Pts',(-26.5018085199062,184.894800861575,-79.6387061173241));
#19428=CARTESIAN_POINT('Ctrl Pts',(-26.7532096955271,184.896605367196,-79.6230686927859));
#19429=CARTESIAN_POINT('Ctrl Pts',(-27.0045509729748,184.897912683916,-79.6069217821172));
#19430=CARTESIAN_POINT('Ctrl Pts',(-28.9907477845154,184.90824361057,-79.4793225958153));
#19431=CARTESIAN_POINT('Ctrl Pts',(-30.9732260056195,184.887510891604,-79.319970845809));
#19432=CARTESIAN_POINT('Ctrl Pts',(-32.951755848961,184.836136694374,-79.1264843643942));
#19433=CARTESIAN_POINT('Ctrl Pts',(-34.58712483348,184.793672958465,-78.966556632349));
#19434=CARTESIAN_POINT('Ctrl Pts',(-36.2197964305512,184.730275751757,-78.78330862021));
#19435=CARTESIAN_POINT('Ctrl Pts',(-37.8496463618853,184.646200267918,-78.5754154614948));
#19436=CARTESIAN_POINT('Ctrl Pts',(-38.3445529765253,184.620670608848,-78.512288361626));
#19437=CARTESIAN_POINT('Ctrl Pts',(-38.8391670257304,184.59323304001,-78.4468923527209));
#19438=CARTESIAN_POINT('Ctrl Pts',(-39.3334992489681,184.563894543215,-78.3791893119185));
#19439=CARTESIAN_POINT('Ctrl Pts',(-40.9140488305578,184.470089311321,-78.1627194809377));
#19440=CARTESIAN_POINT('Ctrl Pts',(-42.4916983624513,184.356837819108,-77.9225453086862));
#19441=CARTESIAN_POINT('Ctrl Pts',(-44.0666753706419,184.224296659025,-77.6566322107026));
#19442=CARTESIAN_POINT('Ctrl Pts',(-44.5304989103894,184.18526389238,-77.5783220171376));
#19443=CARTESIAN_POINT('Ctrl Pts',(-44.9940906480806,184.144557963664,-77.4977792877235));
#19444=CARTESIAN_POINT('Ctrl Pts',(-45.4574563428166,184.102182331615,-77.4149513693389));
#19445=CARTESIAN_POINT('Ctrl Pts',(-46.4756789541978,184.00906402956,-77.2329412198805));
#19446=CARTESIAN_POINT('Ctrl Pts',(-47.4928067767693,183.907882722016,-77.0398762547174));
#19447=CARTESIAN_POINT('Ctrl Pts',(-48.5088764533298,183.798668678686,-76.8350434911382));
#19448=CARTESIAN_POINT('Ctrl Pts',(-48.7905784132376,183.768389446105,-76.7782542843696));
#19449=CARTESIAN_POINT('Ctrl Pts',(-49.072205880457,183.73748883725,-76.7205542596092));
#19450=CARTESIAN_POINT('Ctrl Pts',(-49.353594996623,183.705990252679,-76.6619665200221));
#19451=CARTESIAN_POINT('Ctrl Pts',(-50.0860997232609,183.623993967981,-76.509452461357));
#19452=CARTESIAN_POINT('Ctrl Pts',(-50.817661700711,183.537867720617,-76.3507823667154));
#19453=CARTESIAN_POINT('Ctrl Pts',(-51.5454344349616,183.447993539071,-76.1863137058566));
#19454=CARTESIAN_POINT('Ctrl Pts',(-52.5893488086163,183.319078363329,-75.9504004997055));
#19455=CARTESIAN_POINT('Ctrl Pts',(-53.6275144052881,183.182241566705,-75.7021915460668));
#19456=CARTESIAN_POINT('Ctrl Pts',(-54.6599414688518,183.0377363009,-75.4409038988655));
#19457=CARTESIAN_POINT('Ctrl Pts',(-55.6097700716653,182.904792057609,-75.2005203505914));
#19458=CARTESIAN_POINT('Ctrl Pts',(-56.5547414352707,182.765357070629,-74.9490668063843));
#19459=CARTESIAN_POINT('Ctrl Pts',(-57.4948450401202,182.619621548287,-74.6858999615784));
#19460=CARTESIAN_POINT('Ctrl Pts',(-58.4547719007016,182.470813010893,-74.4171839159847));
#19461=CARTESIAN_POINT('Ctrl Pts',(-59.4096299264397,182.315431591912,-74.136266643455));
#19462=CARTESIAN_POINT('Ctrl Pts',(-60.3592589587275,182.153712006982,-73.8422126425771));
#19463=CARTESIAN_POINT('Ctrl Pts',(-60.4364200749712,182.140571650835,-73.8183195915306));
#19464=CARTESIAN_POINT('Ctrl Pts',(-60.5135466547183,182.127389446893,-73.7943397839875));
#19465=CARTESIAN_POINT('Ctrl Pts',(-60.5906386047577,182.114165520119,-73.7702727046069));
#19466=CARTESIAN_POINT('Ctrl Pts',(-61.4871617108446,181.960380904474,-73.4903901390501));
#19467=CARTESIAN_POINT('Ctrl Pts',(-62.378843094726,181.800977623905,-73.1987553513707));
#19468=CARTESIAN_POINT('Ctrl Pts',(-63.2654994241718,181.636164462385,-72.8945617944821));
#19469=CARTESIAN_POINT('Ctrl Pts',(-64.1932340557345,181.463715597361,-72.5762751167111));
#19470=CARTESIAN_POINT('Ctrl Pts',(-65.1154789896928,181.285337902937,-72.2442595652156));
#19471=CARTESIAN_POINT('Ctrl Pts',(-66.0318123592137,181.101342645502,-71.8972293164849));
#19472=CARTESIAN_POINT('Ctrl Pts',(-66.8326026625298,180.940547870466,-71.5939570933133));
#19473=CARTESIAN_POINT('Ctrl Pts',(-67.6288742820847,180.775468201812,-71.2792231566612));
#19474=CARTESIAN_POINT('Ctrl Pts',(-68.4204040726826,180.606290606281,-70.9520943939504));
#19475=CARTESIAN_POINT('Ctrl Pts',(-68.5608266260415,180.576277396143,-70.8940596153702));
#19476=CARTESIAN_POINT('Ctrl Pts',(-68.7010998749578,180.546135213193,-70.835634617901));
#19477=CARTESIAN_POINT('Ctrl Pts',(-68.841222488813,180.515865104335,-70.7768140396236));
#19478=CARTESIAN_POINT('Ctrl Pts',(-69.5818936550052,180.355860975009,-70.4658955867758));
#19479=CARTESIAN_POINT('Ctrl Pts',(-70.3183392970407,180.192289767342,-70.1438963096542));
#19480=CARTESIAN_POINT('Ctrl Pts',(-71.050229845743,180.025357594668,-69.8097965221065));
#19481=CARTESIAN_POINT('Ctrl Pts',(-71.1460330992753,180.003506451366,-69.7660634165099));
#19482=CARTESIAN_POINT('Ctrl Pts',(-71.2417582683773,179.981597725142,-69.7221229124221));
#19483=CARTESIAN_POINT('Ctrl Pts',(-71.3374045811306,179.959631883187,-69.6779726643808));
#19484=CARTESIAN_POINT('Ctrl Pts',(-71.407777809868,179.943470181017,-69.6454884481597));
#19485=CARTESIAN_POINT('Ctrl Pts',(-71.4781084628288,179.927277560157,-69.612890661583));
#19486=CARTESIAN_POINT('Ctrl Pts',(-71.5483972204143,179.911053977661,-69.5801779008149));
#19487=CARTESIAN_POINT('Ctrl Pts',(-71.9837167618859,179.810576422841,-69.3775778761874));
#19488=CARTESIAN_POINT('Ctrl Pts',(-72.4175547523421,179.708871552097,-69.1704715579982));
#19489=CARTESIAN_POINT('Ctrl Pts',(-72.8489072435447,179.606229298099,-68.9591086722214));
#19490=CARTESIAN_POINT('Ctrl Pts',(-73.2108088745924,179.520113186812,-68.7817767345008));
#19491=CARTESIAN_POINT('Ctrl Pts',(-73.5709606302885,179.433337187436,-68.601448242336));
#19492=CARTESIAN_POINT('Ctrl Pts',(-73.9287415278322,179.346076081554,-68.4182667355679));
#19493=CARTESIAN_POINT('Ctrl Pts',(-74.0152614109623,179.324974282283,-68.3739691146888));
#19494=CARTESIAN_POINT('Ctrl Pts',(-74.1016508240775,179.303841974661,-68.329500240179));
#19495=CARTESIAN_POINT('Ctrl Pts',(-74.1878981569291,179.282682307813,-68.2848633631352));
#19496=CARTESIAN_POINT('Ctrl Pts',(-74.9520405519443,179.095209861207,-67.8893852770014));
#19497=CARTESIAN_POINT('Ctrl Pts',(-75.7068985668535,178.905157510695,-67.4799676364347));
#19498=CARTESIAN_POINT('Ctrl Pts',(-76.4510161725052,178.71327515797,-67.0555357540613));
#19499=CARTESIAN_POINT('Ctrl Pts',(-76.9578846194199,178.582571208248,-66.7664267108056));
#19500=CARTESIAN_POINT('Ctrl Pts',(-77.4598402991781,178.450997227197,-66.4703085533318));
#19501=CARTESIAN_POINT('Ctrl Pts',(-77.9566463445384,178.318729280589,-66.1666611079086));
#19502=CARTESIAN_POINT('Ctrl Pts',(-78.3570807339144,178.212118994889,-65.921915939187));
#19503=CARTESIAN_POINT('Ctrl Pts',(-78.7541689603514,178.105058023274,-65.6722787015837));
#19504=CARTESIAN_POINT('Ctrl Pts',(-79.1477690647678,177.997644212194,-65.4174609479341));
#19505=CARTESIAN_POINT('Ctrl Pts',(-79.5939502217359,177.875880986106,-65.1286020811207));
#19506=CARTESIAN_POINT('Ctrl Pts',(-80.03566857104,177.753656057224,-64.833103516267));
#19507=CARTESIAN_POINT('Ctrl Pts',(-80.4725490551237,177.63117690159,-64.5303986499002));
#19508=CARTESIAN_POINT('Ctrl Pts',(-80.7344890850065,177.557742186936,-64.3489061716813));
#19509=CARTESIAN_POINT('Ctrl Pts',(-80.9946892979568,177.48421632754,-64.1648225373259));
#19510=CARTESIAN_POINT('Ctrl Pts',(-81.2530623554429,177.410646455889,-63.9780198133583));
#19511=CARTESIAN_POINT('Ctrl Pts',(-81.6419444022845,177.299915087256,-63.696859593485));
#19512=CARTESIAN_POINT('Ctrl Pts',(-82.0267334585135,177.189095393788,-63.4095470563223));
#19513=CARTESIAN_POINT('Ctrl Pts',(-82.4071387809341,177.078326593046,-63.1155673632256));
#19514=CARTESIAN_POINT('Ctrl Pts',(-82.7804815138832,176.969614321275,-62.8270456849435));
#19515=CARTESIAN_POINT('Ctrl Pts',(-83.1496018524829,176.860950988961,-62.5321021503129));
#19516=CARTESIAN_POINT('Ctrl Pts',(-83.5141887379417,176.752482541153,-62.2302206105805));
#19517=CARTESIAN_POINT('Ctrl Pts',(-83.5514766168838,176.741389003475,-62.1993458787748));
#19518=CARTESIAN_POINT('Ctrl Pts',(-83.5887172775307,176.730297571654,-62.1683985707106));
#19519=CARTESIAN_POINT('Ctrl Pts',(-83.6259104466999,176.719208410275,-62.1373780905463));
#19520=CARTESIAN_POINT('Ctrl Pts',(-83.9558178441684,176.620846360133,-61.8622231062355));
#19521=CARTESIAN_POINT('Ctrl Pts',(-84.2819553798721,176.522676464612,-61.5812821073024));
#19522=CARTESIAN_POINT('Ctrl Pts',(-84.604034142111,176.424851647322,-61.2940527224133));
#19523=CARTESIAN_POINT('Ctrl Pts',(-84.6228412574001,176.41913937184,-61.2772805635833));
#19524=CARTESIAN_POINT('Ctrl Pts',(-84.6416345369846,176.413428270688,-61.260486939101));
#19525=CARTESIAN_POINT('Ctrl Pts',(-84.6604139206614,176.407718374571,-61.2436717431479));
#19526=CARTESIAN_POINT('Ctrl Pts',(-84.8808984780687,176.340679757123,-61.0462482759436));
#19527=CARTESIAN_POINT('Ctrl Pts',(-85.0996941313493,176.273736013823,-60.8456211532969));
#19528=CARTESIAN_POINT('Ctrl Pts',(-85.3158922454133,176.207191546391,-60.6423925159304));
#19529=CARTESIAN_POINT('Ctrl Pts',(-85.4300515625353,176.172054001399,-60.5350814852035));
#19530=CARTESIAN_POINT('Ctrl Pts',(-85.5434859458774,176.137028005454,-60.4270455100516));
#19531=CARTESIAN_POINT('Ctrl Pts',(-85.6560566970487,176.102159964998,-60.3183761224715));
#19532=CARTESIAN_POINT('Ctrl Pts',(-85.6581590166629,176.101508785499,-60.3163466629308));
#19533=CARTESIAN_POINT('Ctrl Pts',(-85.6602610537763,176.100857655553,-60.3143169678148));
#19534=CARTESIAN_POINT('Ctrl Pts',(-85.6623628082838,176.100206575221,-60.3122870370121));
#19535=CARTESIAN_POINT('Ctrl Pts',(-85.9655775819481,176.006276872874,-60.0194340864486));
#19536=CARTESIAN_POINT('Ctrl Pts',(-86.2628725546031,175.913391296893,-59.7217178015255));
#19537=CARTESIAN_POINT('Ctrl Pts',(-86.5539294847292,175.821739230135,-59.4187834172871));
#19538=CARTESIAN_POINT('Ctrl Pts',(-86.839402798911,175.731845410264,-59.1216605052483));
#19539=CARTESIAN_POINT('Ctrl Pts',(-87.1188751736362,175.643138147991,-58.8195178119657));
#19540=CARTESIAN_POINT('Ctrl Pts',(-87.3920035701138,175.555813880903,-58.5120004904891));
#19541=CARTESIAN_POINT('Ctrl Pts',(-87.426799101105,175.544689097538,-58.4728239397248));
#19542=CARTESIAN_POINT('Ctrl Pts',(-87.4614916119104,175.533586784895,-58.4335601321732));
#19543=CARTESIAN_POINT('Ctrl Pts',(-87.4960803413495,175.522507371371,-58.3942083096898));
#19544=CARTESIAN_POINT('Ctrl Pts',(-87.7552552800019,175.439488816853,-58.0993432960449));
#19545=CARTESIAN_POINT('Ctrl Pts',(-88.0086095980277,175.357753517098,-57.7995395611124));
#19546=CARTESIAN_POINT('Ctrl Pts',(-88.25573352756,175.277510566065,-57.4944372405943));
#19547=CARTESIAN_POINT('Ctrl Pts',(-88.4979680292567,175.198855248083,-57.1953714693554));
#19548=CARTESIAN_POINT('Ctrl Pts',(-88.734216305342,175.12163374876,-56.8912147377849));
#19549=CARTESIAN_POINT('Ctrl Pts',(-88.9640500525986,175.046061324727,-56.5816081863863));
#19550=CARTESIAN_POINT('Ctrl Pts',(-89.0160581643391,175.028960358831,-56.5115486224061));
#19551=CARTESIAN_POINT('Ctrl Pts',(-89.067737641556,175.011943911971,-56.4412099156939));
#19552=CARTESIAN_POINT('Ctrl Pts',(-89.1190832067734,174.995014617266,-56.370587759921));
#19553=CARTESIAN_POINT('Ctrl Pts',(-89.2169920966178,174.962732794223,-56.2359210785657));
#19554=CARTESIAN_POINT('Ctrl Pts',(-89.3136877484593,174.930767566929,-56.1002241654811));
#19555=CARTESIAN_POINT('Ctrl Pts',(-89.4091250351677,174.899139899188,-55.963463250108));
#19556=CARTESIAN_POINT('Ctrl Pts',(-89.5843332274473,174.841076361527,-55.7123912259186));
#19557=CARTESIAN_POINT('Ctrl Pts',(-89.7552435157444,174.784171529238,-55.4578272928341));
#19558=CARTESIAN_POINT('Ctrl Pts',(-89.9216547016079,174.728529608786,-55.1994155525535));
#19559=CARTESIAN_POINT('Ctrl Pts',(-90.0842201292001,174.674173571701,-54.9469757010161));
#19560=CARTESIAN_POINT('Ctrl Pts',(-90.2424920738752,174.621022683459,-54.6908638683083));
#19561=CARTESIAN_POINT('Ctrl Pts',(-90.3962399116234,174.569189839793,-54.4307284026853));
#19562=CARTESIAN_POINT('Ctrl Pts',(-90.4338181432748,174.556521130854,-54.3671474708747));
#19563=CARTESIAN_POINT('Ctrl Pts',(-90.4711259025328,174.543931237885,-54.3033260766955));
#19564=CARTESIAN_POINT('Ctrl Pts',(-90.5081594097971,174.531421964099,-54.2392588953588));
#19565=CARTESIAN_POINT('Ctrl Pts',(-90.6258211678479,174.491677871404,-54.0357065519191));
#19566=CARTESIAN_POINT('Ctrl Pts',(-90.7408707175398,174.452693862087,-53.829342570037));
#19567=CARTESIAN_POINT('Ctrl Pts',(-90.8528197264801,174.414652822771,-53.6206616697916));
#19568=CARTESIAN_POINT('Ctrl Pts',(-90.8770642398965,174.406414371204,-53.5754681755962));
#19569=CARTESIAN_POINT('Ctrl Pts',(-90.9011631887087,174.398220198498,-53.530166131445));
#19570=CARTESIAN_POINT('Ctrl Pts',(-90.9251113671707,174.390072250981,-53.484760763727));
#19571=CARTESIAN_POINT('Ctrl Pts',(-90.9870859608341,174.36898648292,-53.3672579140252));
#19572=CARTESIAN_POINT('Ctrl Pts',(-91.0479909645711,174.348231072408,-53.2491784445003));
#19573=CARTESIAN_POINT('Ctrl Pts',(-91.1077374489716,174.327839629328,-53.1306240306533));
#19574=CARTESIAN_POINT('Ctrl Pts',(-91.2675020972162,174.273312040576,-52.8136044701529));
#19575=CARTESIAN_POINT('Ctrl Pts',(-91.4188853491734,174.221422147604,-52.4935170045305));
#19576=CARTESIAN_POINT('Ctrl Pts',(-91.5616044369495,174.172333458547,-52.1701322125482));
#19577=CARTESIAN_POINT('Ctrl Pts',(-91.5858008658025,174.164011019055,-52.1153059294401));
#19578=CARTESIAN_POINT('Ctrl Pts',(-91.6097481465213,174.155769142893,-52.0603848529147));
#19579=CARTESIAN_POINT('Ctrl Pts',(-91.6334447650117,174.147608685332,-52.0053678440317));
#19580=CARTESIAN_POINT('Ctrl Pts',(-91.7693244902838,174.100815480134,-51.6898926189329));
#19581=CARTESIAN_POINT('Ctrl Pts',(-91.896975170158,174.056697446588,-51.3712649984069));
#19582=CARTESIAN_POINT('Ctrl Pts',(-92.0160413151778,174.015428122255,-51.0492598743207));
#19583=CARTESIAN_POINT('Ctrl Pts',(-92.0460469028125,174.005027933959,-50.9681120974444));
#19584=CARTESIAN_POINT('Ctrl Pts',(-92.0755070693359,173.99480875918,-50.8867497863239));
#19585=CARTESIAN_POINT('Ctrl Pts',(-92.1044156446447,173.984773576468,-50.8051692644594));
#19586=CARTESIAN_POINT('Ctrl Pts',(-92.2246834254259,173.943024401988,-50.4657714140016));
#19587=CARTESIAN_POINT('Ctrl Pts',(-92.3353783621527,173.904467096425,-50.1226731650209));
#19588=CARTESIAN_POINT('Ctrl Pts',(-92.4360240236092,173.86933179434,-49.7756598162833));
#19589=CARTESIAN_POINT('Ctrl Pts',(-92.441460980855,173.867433757878,-49.756913884134));
#19590=CARTESIAN_POINT('Ctrl Pts',(-92.4468686004058,173.865545712799,-49.7381565249075));
#19591=CARTESIAN_POINT('Ctrl Pts',(-92.4522468032086,173.863667697162,-49.7193877041164));
#19592=CARTESIAN_POINT('Ctrl Pts',(-92.5472941682945,173.830478090055,-49.3876919634805));
#19593=CARTESIAN_POINT('Ctrl Pts',(-92.6331595635202,173.800418977058,-49.0524173856645));
#19594=CARTESIAN_POINT('Ctrl Pts',(-92.7093120482644,173.773713629046,-48.7133594415447));
#19595=CARTESIAN_POINT('Ctrl Pts',(-92.7651362071759,173.7541370703,-48.4648104333761));
#19596=CARTESIAN_POINT('Ctrl Pts',(-92.8157399774473,173.736363111541,-48.2142281953996));
#19597=CARTESIAN_POINT('Ctrl Pts',(-92.8608978789791,173.720486412539,-47.9615295291183));
#19598=CARTESIAN_POINT('Ctrl Pts',(-92.8951771189541,173.7084344536,-47.7697066602743));
#19599=CARTESIAN_POINT('Ctrl Pts',(-92.9261641075478,173.697529207677,-47.5775127333407));
#19600=CARTESIAN_POINT('Ctrl Pts',(-92.9538384701856,173.687784900467,-47.3849592374246));
#19601=CARTESIAN_POINT('Ctrl Pts',(-93.011917690001,173.667334862727,-46.9808539302176));
#19602=CARTESIAN_POINT('Ctrl Pts',(-93.0554077638896,173.651998516184,-46.5751636385015));
#19603=CARTESIAN_POINT('Ctrl Pts',(-93.0840095834533,173.641905099212,-46.1679806000269));
#19604=CARTESIAN_POINT('Ctrl Pts',(-93.1112639346017,173.632287196064,-45.7799804769057));
#19605=CARTESIAN_POINT('Ctrl Pts',(-93.1249999999199,173.627429788604,-45.3906249750178));
#19606=CARTESIAN_POINT('Ctrl Pts',(-93.125,173.627429788614,-45.));
#19607=CARTESIAN_POINT('Origin',(-40.3363668356791,225.625863228014,34.2057557851749));
#19608=CARTESIAN_POINT('Origin',(-133.630782057879,206.966980183574,47.2669739162829));
#19609=CARTESIAN_POINT('Ctrl Pts',(-126.766717328043,172.646656534391,47.2669739162829));
#19610=CARTESIAN_POINT('Ctrl Pts',(-122.224200046663,173.555159990667,81.0113880065328));
#19611=CARTESIAN_POINT('Ctrl Pts',(-128.778107499175,206.966980183574,81.9289350498845));
#19612=CARTESIAN_POINT('Ctrl Pts',(-125.076099494732,172.984780101054,46.9474471457708));
#19613=CARTESIAN_POINT('Ctrl Pts',(-120.489909983146,173.820474755958,80.7685873976232));
#19614=CARTESIAN_POINT('Ctrl Pts',(-126.495773409643,207.423447001473,81.6094082773501));
#19615=CARTESIAN_POINT('Ctrl Pts',(-123.376736606944,173.279171828244,46.6262675599665));
#19616=CARTESIAN_POINT('Ctrl Pts',(-118.752370779924,174.039540392876,80.5253319092848));
#19617=CARTESIAN_POINT('Ctrl Pts',(-124.201633525813,207.820875830352,81.2882286936138));
#19618=CARTESIAN_POINT('Ctrl Pts',(-121.670898717897,173.529438457885,46.3038641989655));
#19619=CARTESIAN_POINT('Ctrl Pts',(-117.014194117273,174.212632196936,80.2819871764182));
#19620=CARTESIAN_POINT('Ctrl Pts',(-121.898752375479,208.15873578029,80.9658253325671));
#19621=CARTESIAN_POINT('Origin',(-126.751426934183,208.15873578029,46.3038641989655));
#19622=CARTESIAN_POINT('Ctrl Pts',(-108.033967922038,209.585728186396,80.0000000000001));
#19623=CARTESIAN_POINT('Ctrl Pts',(-107.806114264457,174.586469869815,80.0000000000001));
#19624=CARTESIAN_POINT('Ctrl Pts',(-107.806114264457,174.586469869815,45.));
#19625=CARTESIAN_POINT('Ctrl Pts',(-110.368245901848,209.565212620413,80.0000000000001));
#19626=CARTESIAN_POINT('Ctrl Pts',(-109.323233110512,174.576593058387,79.9946819507977));
#19627=CARTESIAN_POINT('Ctrl Pts',(-110.140392035487,174.571273155555,44.9999999999672));
#19628=CARTESIAN_POINT('Ctrl Pts',(-112.690630392194,209.434596373781,80.0816280345492));
#19629=CARTESIAN_POINT('Ctrl Pts',(-110.831769330981,174.542829711498,80.0133399191142));
#19630=CARTESIAN_POINT('Ctrl Pts',(-112.462776734607,174.474520378982,45.1101978466734));
#19631=CARTESIAN_POINT('Ctrl Pts',(-117.312108354281,208.957898622415,80.4044093761842));
#19632=CARTESIAN_POINT('Ctrl Pts',(-113.886869252213,174.421832152824,80.1038421117714));
#19633=CARTESIAN_POINT('Ctrl Pts',(-117.084254696706,174.121410933541,45.5459526578167));
#19634=CARTESIAN_POINT('Ctrl Pts',(-119.611215134957,208.611807682767,80.645570118894));
#19635=CARTESIAN_POINT('Ctrl Pts',(-115.428565673973,174.334921359983,80.1754126411297));
#19636=CARTESIAN_POINT('Ctrl Pts',(-119.383361285288,173.865047302731,45.8715196241861));
#19637=CARTESIAN_POINT('Ctrl Pts',(-121.898752375479,208.15873578029,80.965825332567));
#19638=CARTESIAN_POINT('Ctrl Pts',(-117.014194117272,174.212632196936,80.2819871764181));
#19639=CARTESIAN_POINT('Ctrl Pts',(-121.670898717897,173.529438457885,46.3038641989654));
#19640=CARTESIAN_POINT('Origin',(-108.033967922038,209.585728186396,45.));
#19641=CARTESIAN_POINT('Origin',(-107.155103814224,74.5885889652995,45.0000000000001));
#19642=CARTESIAN_POINT('Origin',(-93.0342906798268,208.848049102839,45.0000000000001));
#19643=CARTESIAN_POINT('Origin',(-115.,0.,45.0000000000001));
#19644=CARTESIAN_POINT('Ctrl Pts',(-93.125,173.627429788614,45.0000000000001));
#19645=CARTESIAN_POINT('Ctrl Pts',(-93.1249999998108,173.62742978859,45.5703854531217));
#19646=CARTESIAN_POINT('Ctrl Pts',(-93.0957247306423,173.637782029819,46.1351652243981));
#19647=CARTESIAN_POINT('Ctrl Pts',(-93.038653950843,173.657902731047,46.6946224880328));
#19648=CARTESIAN_POINT('Ctrl Pts',(-93.0151077973288,173.666204091596,46.9254422991599));
#19649=CARTESIAN_POINT('Ctrl Pts',(-92.986829698282,173.676168463279,47.155356013543));
#19650=CARTESIAN_POINT('Ctrl Pts',(-92.9539212025254,173.687755741858,47.384383122678));
#19651=CARTESIAN_POINT('Ctrl Pts',(-92.9273987437467,173.697094458545,47.5689665234563));
#19652=CARTESIAN_POINT('Ctrl Pts',(-92.8978677052669,173.707487484341,47.7529742044882));
#19653=CARTESIAN_POINT('Ctrl Pts',(-92.8653667429934,173.718915089093,47.9364143980648));
#19654=CARTESIAN_POINT('Ctrl Pts',(-92.8078734084644,173.739130216795,48.2609152028896));
#19655=CARTESIAN_POINT('Ctrl Pts',(-92.7410476493066,173.762598797023,48.5838620304402));
#19656=CARTESIAN_POINT('Ctrl Pts',(-92.6651291805777,173.789202135506,48.9050632039656));
#19657=CARTESIAN_POINT('Ctrl Pts',(-92.6008395531292,173.811730497162,49.177064261517));
#19658=CARTESIAN_POINT('Ctrl Pts',(-92.530030351504,173.836506504464,49.4478136279032));
#19659=CARTESIAN_POINT('Ctrl Pts',(-92.4528745253981,173.863448838665,49.7171990214557));
#19660=CARTESIAN_POINT('Ctrl Pts',(-92.3606101775622,173.895666974608,50.0393350014215));
#19661=CARTESIAN_POINT('Ctrl Pts',(-92.2592673536355,173.930983612063,50.3595200750698));
#19662=CARTESIAN_POINT('Ctrl Pts',(-92.1491224618084,173.969248257698,50.6775593968402));
#19663=CARTESIAN_POINT('Ctrl Pts',(-92.1374506250882,173.973303086648,50.7112613958408));
#19664=CARTESIAN_POINT('Ctrl Pts',(-92.1256799934841,173.977391005235,50.7449393065516));
#19665=CARTESIAN_POINT('Ctrl Pts',(-92.1138109280872,173.981511824407,50.7785929019537));
#19666=CARTESIAN_POINT('Ctrl Pts',(-92.0044728350165,174.019472901806,51.088610567473));
#19667=CARTESIAN_POINT('Ctrl Pts',(-91.8874014722842,174.060011293566,51.3948244481383));
#19668=CARTESIAN_POINT('Ctrl Pts',(-91.7630218111992,174.102936771868,51.697462505704));
#19669=CARTESIAN_POINT('Ctrl Pts',(-91.7213243161257,174.117327267101,51.7989200012811));
#19670=CARTESIAN_POINT('Ctrl Pts',(-91.6788050567026,174.131986213741,51.8999755541278));
#19671=CARTESIAN_POINT('Ctrl Pts',(-91.6354788602119,174.1469069512,52.0006375683561));
#19672=CARTESIAN_POINT('Ctrl Pts',(-91.5019434891281,174.192894053112,52.3108872674477));
#19673=CARTESIAN_POINT('Ctrl Pts',(-91.3607375382183,174.24136675191,52.6173978737244));
#19674=CARTESIAN_POINT('Ctrl Pts',(-91.2122219564331,174.292145465175,52.9204043353714));
#19675=CARTESIAN_POINT('Ctrl Pts',(-91.1788225996643,174.303564983183,52.9885468211238));
#19676=CARTESIAN_POINT('Ctrl Pts',(-91.145053372545,174.31510121109,53.05651205668));
#19677=CARTESIAN_POINT('Ctrl Pts',(-91.1109180542637,174.326752250885,53.1243026631603));
#19678=CARTESIAN_POINT('Ctrl Pts',(-91.0521049058449,174.346826308115,53.2411018963612));
#19679=CARTESIAN_POINT('Ctrl Pts',(-90.9921666735604,174.367253920307,53.3574364564119));
#19680=CARTESIAN_POINT('Ctrl Pts',(-90.9312096089697,174.387995830875,53.4731771255933));
#19681=CARTESIAN_POINT('Ctrl Pts',(-90.8246553600374,174.424253132909,53.6754942837171));
#19682=CARTESIAN_POINT('Ctrl Pts',(-90.7149851721648,174.461470136965,53.8759974934974));
#19683=CARTESIAN_POINT('Ctrl Pts',(-90.6027342996058,174.499449100598,54.074036380043));
#19684=CARTESIAN_POINT('Ctrl Pts',(-90.5725830611701,174.509650471527,54.1272307789074));
#19685=CARTESIAN_POINT('Ctrl Pts',(-90.5422454352643,174.519906887338,54.1802475882314));
#19686=CARTESIAN_POINT('Ctrl Pts',(-90.5117313782821,174.530214666933,54.233074650745));
#19687=CARTESIAN_POINT('Ctrl Pts',(-90.3527342599104,174.583924576873,54.5083363347816));
#19688=CARTESIAN_POINT('Ctrl Pts',(-90.1886986672789,174.63911456029,54.7790268575882));
#19689=CARTESIAN_POINT('Ctrl Pts',(-90.0199441738519,174.695636393522,55.0455065671526));
#19690=CARTESIAN_POINT('Ctrl Pts',(-89.8474021802967,174.753426794164,55.3179671067002));
#19691=CARTESIAN_POINT('Ctrl Pts',(-89.6699270040715,174.81260956482,55.5860256574295));
#19692=CARTESIAN_POINT('Ctrl Pts',(-89.4878140788683,174.87304413341,55.8500453507872));
#19693=CARTESIAN_POINT('Ctrl Pts',(-89.4637239539776,174.881038493522,55.8849702051295));
#19694=CARTESIAN_POINT('Ctrl Pts',(-89.4395526126323,174.889054782192,55.9198243558653));
#19695=CARTESIAN_POINT('Ctrl Pts',(-89.4153006812224,174.897092695787,55.9546086161183));
#19696=CARTESIAN_POINT('Ctrl Pts',(-89.319261936399,174.928923197019,56.0923558593315));
#19697=CARTESIAN_POINT('Ctrl Pts',(-89.2219626997243,174.961090994622,56.2290004746553));
#19698=CARTESIAN_POINT('Ctrl Pts',(-89.1234500151856,174.993574426559,56.3645787456421));
#19699=CARTESIAN_POINT('Ctrl Pts',(-88.899087950989,175.067555253247,56.6733574666893));
#19700=CARTESIAN_POINT('Ctrl Pts',(-88.6684301573737,175.143173436595,56.9766043214186));
#19701=CARTESIAN_POINT('Ctrl Pts',(-88.4319084098773,175.220215129991,57.2746888173799));
#19702=CARTESIAN_POINT('Ctrl Pts',(-88.190557746909,175.298829735092,57.578859116654));
#19703=CARTESIAN_POINT('Ctrl Pts',(-87.9431011781495,175.378926632654,57.8776540776403));
#19704=CARTESIAN_POINT('Ctrl Pts',(-87.6899520658236,175.460298134701,58.1714442031506));
#19705=CARTESIAN_POINT('Ctrl Pts',(-87.6281678364518,175.48015787468,58.2431473836789));
#19706=CARTESIAN_POINT('Ctrl Pts',(-87.5660443165453,175.50009362537,58.3145523435447));
#19707=CARTESIAN_POINT('Ctrl Pts',(-87.5035871237125,175.520102532267,58.3856642785872));
#19708=CARTESIAN_POINT('Ctrl Pts',(-87.2350633724273,175.606127319733,58.6913975767498));
#19709=CARTESIAN_POINT('Ctrl Pts',(-86.9603723263989,175.693503929557,58.9917147375286));
#19710=CARTESIAN_POINT('Ctrl Pts',(-86.6798569195729,175.782039633885,59.2869796049606));
#19711=CARTESIAN_POINT('Ctrl Pts',(-86.3937700864287,175.872333780499,59.5881088435223));
#19712=CARTESIAN_POINT('Ctrl Pts',(-86.1016251709388,175.96383360254,59.8839830696031));
#19713=CARTESIAN_POINT('Ctrl Pts',(-85.8037404597079,176.056353351122,60.1749661075604));
#19714=CARTESIAN_POINT('Ctrl Pts',(-85.7621131907888,176.0692823277,60.2156289167454));
#19715=CARTESIAN_POINT('Ctrl Pts',(-85.7203737644335,176.082231249576,60.2561961763065));
#19716=CARTESIAN_POINT('Ctrl Pts',(-85.6785229814522,176.095199636747,60.2966688461824));
#19717=CARTESIAN_POINT('Ctrl Pts',(-85.6755866033166,176.096109538207,60.2995085317138));
#19718=CARTESIAN_POINT('Ctrl Pts',(-85.6726496819324,176.097019533954,60.3023477467889));
#19719=CARTESIAN_POINT('Ctrl Pts',(-85.6697122175902,176.097929623816,60.3051864917303));
#19720=CARTESIAN_POINT('Ctrl Pts',(-85.4253294684895,176.173644674843,60.5413562667317));
#19721=CARTESIAN_POINT('Ctrl Pts',(-85.1768557609506,176.250107482301,60.7745219435438));
#19722=CARTESIAN_POINT('Ctrl Pts',(-84.9250673075622,176.327042272143,61.0043417974612));
#19723=CARTESIAN_POINT('Ctrl Pts',(-84.6640070957159,176.406810078268,61.2426244468155));
#19724=CARTESIAN_POINT('Ctrl Pts',(-84.3993834390816,176.48708530926,61.4773104469835));
#19725=CARTESIAN_POINT('Ctrl Pts',(-84.1320102189896,176.567577409112,61.7080365871725));
#19726=CARTESIAN_POINT('Ctrl Pts',(-83.9689546335988,176.616664922275,61.8487432212944));
#19727=CARTESIAN_POINT('Ctrl Pts',(-83.8048754731111,176.665833414535,61.9879774868914));
#19728=CARTESIAN_POINT('Ctrl Pts',(-83.6399487552332,176.71501976099,62.1256597309597));
#19729=CARTESIAN_POINT('Ctrl Pts',(-83.603725747223,176.72582260388,62.1558990099189));
#19730=CARTESIAN_POINT('Ctrl Pts',(-83.5674583869559,176.736627418291,62.1860681891631));
#19731=CARTESIAN_POINT('Ctrl Pts',(-83.5311469089632,176.747434063254,62.2161678518087));
#19732=CARTESIAN_POINT('Ctrl Pts',(-83.1608098696161,176.857649926731,62.5231512236161));
#19733=CARTESIAN_POINT('Ctrl Pts',(-82.7858618806584,176.968045925943,62.822898654204));
#19734=CARTESIAN_POINT('Ctrl Pts',(-82.4066290249949,177.078471627047,63.1159641240302));
#19735=CARTESIAN_POINT('Ctrl Pts',(-82.0307904452302,177.187908976824,63.4064065482892));
#19736=CARTESIAN_POINT('Ctrl Pts',(-81.6507431062853,177.29737565131,63.6902859085264));
#19737=CARTESIAN_POINT('Ctrl Pts',(-81.2667672330688,177.406739868464,63.9681105627763));
#19738=CARTESIAN_POINT('Ctrl Pts',(-80.8367583674063,177.529215227576,64.2792422581777));
#19739=CARTESIAN_POINT('Ctrl Pts',(-80.4017673145224,177.651546575252,64.5827722310067));
#19740=CARTESIAN_POINT('Ctrl Pts',(-79.9621900595459,177.773520712408,64.8792981054518));
#19741=CARTESIAN_POINT('Ctrl Pts',(-79.6949806088862,177.847666136939,65.0595497338513));
#19742=CARTESIAN_POINT('Ctrl Pts',(-79.4260757287456,177.921679850411,65.2372125436568));
#19743=CARTESIAN_POINT('Ctrl Pts',(-79.1555577084484,177.99551638268,65.4124146719346));
#19744=CARTESIAN_POINT('Ctrl Pts',(-78.6678978020531,178.128620700001,65.7282496517351));
#19745=CARTESIAN_POINT('Ctrl Pts',(-78.174974935409,178.261158296907,66.0360692211114));
#19746=CARTESIAN_POINT('Ctrl Pts',(-77.6770538946029,178.392947212377,66.3364299472173));
#19747=CARTESIAN_POINT('Ctrl Pts',(-77.2752739443468,178.499289663414,66.5787955186708));
#19748=CARTESIAN_POINT('Ctrl Pts',(-76.8702388268825,178.605144922234,66.8163038125245));
#19749=CARTESIAN_POINT('Ctrl Pts',(-76.4620699385986,178.710422801494,67.0492309684832));
#19750=CARTESIAN_POINT('Ctrl Pts',(-75.7676341385142,178.88953671834,67.4455202510635));
#19751=CARTESIAN_POINT('Ctrl Pts',(-75.0640159311286,179.067016755113,67.8286240092616));
#19752=CARTESIAN_POINT('Ctrl Pts',(-74.3523513864555,179.242262974854,68.1994629803233));
#19753=CARTESIAN_POINT('Ctrl Pts',(-74.3001475880404,179.255118074067,68.2266656884457));
#19754=CARTESIAN_POINT('Ctrl Pts',(-74.2479004819618,179.267961168359,68.2538023873426));
#19755=CARTESIAN_POINT('Ctrl Pts',(-74.1956105112451,179.280792028091,68.2808734338598));
#19756=CARTESIAN_POINT('Ctrl Pts',(-74.1106840385824,179.301631199414,68.3248407274056));
#19757=CARTESIAN_POINT('Ctrl Pts',(-74.0256241492911,179.32244285591,68.3686431530313));
#19758=CARTESIAN_POINT('Ctrl Pts',(-73.9404393252445,179.343224564154,68.4122787524547));
#19759=CARTESIAN_POINT('Ctrl Pts',(-73.4939121922517,179.452159420861,68.6410105638429));
#19760=CARTESIAN_POINT('Ctrl Pts',(-73.0437861609672,179.560317898584,68.865252552359));
#19761=CARTESIAN_POINT('Ctrl Pts',(-72.5909626258734,179.6674285339,69.0848598562164));
#19762=CARTESIAN_POINT('Ctrl Pts',(-72.2477173132217,179.748619595445,69.2513246528342));
#19763=CARTESIAN_POINT('Ctrl Pts',(-71.9029207067315,179.829208827108,69.4151263648389));
#19764=CARTESIAN_POINT('Ctrl Pts',(-71.5569461393784,179.909080577907,69.5761985292671));
#19765=CARTESIAN_POINT('Ctrl Pts',(-71.4878049613763,179.925042522687,69.6083879450301));
#19766=CARTESIAN_POINT('Ctrl Pts',(-71.418625045659,179.94097409477,69.6404652116115));
#19767=CARTESIAN_POINT('Ctrl Pts',(-71.3494059445144,179.956875294743,69.6724315951806));
#19768=CARTESIAN_POINT('Ctrl Pts',(-70.620066360206,180.12442116556,70.0092511799283));
#19769=CARTESIAN_POINT('Ctrl Pts',(-69.8860898581444,180.288658175961,70.3338945491597));
#19770=CARTESIAN_POINT('Ctrl Pts',(-69.1478094783436,180.449378512452,70.6473765849958));
#19771=CARTESIAN_POINT('Ctrl Pts',(-69.047516772658,180.471211785889,70.6899619799461));
#19772=CARTESIAN_POINT('Ctrl Pts',(-68.9471446035588,180.492980167431,70.7323413329162));
#19773=CARTESIAN_POINT('Ctrl Pts',(-68.8466937699905,180.514683141084,70.7745171247771));
#19774=CARTESIAN_POINT('Ctrl Pts',(-68.0582330320637,180.685034565894,71.1055642131092));
#19775=CARTESIAN_POINT('Ctrl Pts',(-67.2649492078607,180.851347580507,71.4241092502634));
#19776=CARTESIAN_POINT('Ctrl Pts',(-66.4670699960451,181.013433614092,71.7310838367989));
#19777=CARTESIAN_POINT('Ctrl Pts',(-66.3245219996644,181.04239168066,71.7859274918314));
#19778=CARTESIAN_POINT('Ctrl Pts',(-66.1818272575054,181.071214828723,71.8404017138963));
#19779=CARTESIAN_POINT('Ctrl Pts',(-66.0389869830734,181.099901984681,71.8945116652855));
#19780=CARTESIAN_POINT('Ctrl Pts',(-65.1193399688903,181.284598194672,72.2428871877396));
#19781=CARTESIAN_POINT('Ctrl Pts',(-64.1936684744158,181.463650393234,72.5761611402097));
#19782=CARTESIAN_POINT('Ctrl Pts',(-63.2624005133239,181.63674053216,72.8956249559814));
#19783=CARTESIAN_POINT('Ctrl Pts',(-62.376972362934,181.801310653719,73.1993638016555));
#19784=CARTESIAN_POINT('Ctrl Pts',(-61.486474404333,181.960496756059,73.4906000796016));
#19785=CARTESIAN_POINT('Ctrl Pts',(-60.5910895271308,182.114088224847,73.7701318404769));
#19786=CARTESIAN_POINT('Ctrl Pts',(-59.5604150468438,182.290886841063,74.0918998976549));
#19787=CARTESIAN_POINT('Ctrl Pts',(-58.5232783791325,182.460276659765,74.3981595579253));
#19788=CARTESIAN_POINT('Ctrl Pts',(-57.4800356321375,182.621919491696,74.6900461765216));
#19789=CARTESIAN_POINT('Ctrl Pts',(-56.6637510422464,182.748396817469,74.9184326660917));
#19790=CARTESIAN_POINT('Ctrl Pts',(-55.8437232434193,182.870134019457,75.1380109600897));
#19791=CARTESIAN_POINT('Ctrl Pts',(-55.0200356674394,182.986992560819,75.3491798901418));
#19792=CARTESIAN_POINT('Ctrl Pts',(-54.0818398570834,183.120096661338,75.5897053165653));
#19793=CARTESIAN_POINT('Ctrl Pts',(-53.138916039872,183.246879328694,75.8193215249152));
#19794=CARTESIAN_POINT('Ctrl Pts',(-52.1914100346049,183.367125045976,76.0385873974286));
#19795=CARTESIAN_POINT('Ctrl Pts',(-51.9664874968378,183.39566942642,76.0906375545963));
#19796=CARTESIAN_POINT('Ctrl Pts',(-51.7412873445566,183.423847988172,76.1421089209594));
#19797=CARTESIAN_POINT('Ctrl Pts',(-51.5158017905921,183.451658932195,76.1930106956108));
#19798=CARTESIAN_POINT('Ctrl Pts',(-50.7914095839582,183.54100403992,76.3565371309545));
#19799=CARTESIAN_POINT('Ctrl Pts',(-50.0648491243609,183.626445028928,76.5139745559305));
#19800=CARTESIAN_POINT('Ctrl Pts',(-49.3379841963483,183.707748524837,76.6652222472324));
#19801=CARTESIAN_POINT('Ctrl Pts',(-49.0517710051111,183.739762908977,76.7247781326885));
#19802=CARTESIAN_POINT('Ctrl Pts',(-48.765428864529,183.771145312749,76.7833912188635));
#19803=CARTESIAN_POINT('Ctrl Pts',(-48.4790950286481,183.801877303775,76.8410480177466));
#19804=CARTESIAN_POINT('Ctrl Pts',(-47.465412426358,183.910675080124,77.0451653332976));
#19805=CARTESIAN_POINT('Ctrl Pts',(-46.4501431481726,184.011533733904,77.2376834765327));
#19806=CARTESIAN_POINT('Ctrl Pts',(-45.4334520952105,184.104382640783,77.4192426182608));
#19807=CARTESIAN_POINT('Ctrl Pts',(-43.9614743671191,184.23881042256,77.6821061618874));
#19808=CARTESIAN_POINT('Ctrl Pts',(-42.4865233282392,184.35644859137,77.9220388612771));
#19809=CARTESIAN_POINT('Ctrl Pts',(-41.0090296046946,184.457102613407,78.1405824168399));
#19810=CARTESIAN_POINT('Ctrl Pts',(-40.4460861266667,184.495453047212,78.2238502286137));
#19811=CARTESIAN_POINT('Ctrl Pts',(-39.882773587587,184.531338201069,78.3040134129349));
#19812=CARTESIAN_POINT('Ctrl Pts',(-39.3191160265197,184.564748496546,78.3811587995839));
#19813=CARTESIAN_POINT('Ctrl Pts',(-38.8279492645467,184.593861965041,78.4483826822721));
#19814=CARTESIAN_POINT('Ctrl Pts',(-38.3365224616305,184.621097710092,78.5133267944161));
#19815=CARTESIAN_POINT('Ctrl Pts',(-37.8448477983021,184.646448347107,78.5760264393378));
#19816=CARTESIAN_POINT('Ctrl Pts',(-35.8495579567748,184.749325050514,78.8304710424678));
#19817=CARTESIAN_POINT('Ctrl Pts',(-33.8497806197686,184.821222887997,79.0480140922849));
#19818=CARTESIAN_POINT('Ctrl Pts',(-31.8457500386124,184.861652872759,79.2310642129745));
#19819=CARTESIAN_POINT('Ctrl Pts',(-30.2338968514672,184.894170939303,79.3782924654847));
#19820=CARTESIAN_POINT('Ctrl Pts',(-28.6192924766604,184.906332737617,79.5032079101486));
#19821=CARTESIAN_POINT('Ctrl Pts',(-27.0020640562796,184.897899772955,79.6070815377235));
#19822=CARTESIAN_POINT('Ctrl Pts',(-26.7516674121844,184.896594090947,79.623164366486));
#19823=CARTESIAN_POINT('Ctrl Pts',(-26.5012074979132,184.89479493717,79.6387417725125));
#19824=CARTESIAN_POINT('Ctrl Pts',(-26.2506843886171,184.892501020704,79.6538158669559));
#19825=CARTESIAN_POINT('Ctrl Pts',(-24.2925620301514,184.874571460701,79.7716370190483));
#19826=CARTESIAN_POINT('Ctrl Pts',(-22.3305986235038,184.826447634977,79.8587103330367));
#19827=CARTESIAN_POINT('Ctrl Pts',(-20.364880005263,184.747551715547,79.9160570352638));
#19828=CARTESIAN_POINT('Ctrl Pts',(-18.4352480461297,184.670104167273,79.9723509668274));
#19829=CARTESIAN_POINT('Ctrl Pts',(-16.5019975076899,184.563003946033,80.));
#19830=CARTESIAN_POINT('Ctrl Pts',(-14.5652173913043,184.425742352699,80.));
#19831=CARTESIAN_POINT('Origin',(3.92135447228743,250.,-28.0096748020595));
#19832=CARTESIAN_POINT('Origin',(-126.751426934183,250.,-46.3038641989653));
#19833=CARTESIAN_POINT('Origin',(-108.033967922038,250.,-180.));
#19834=CARTESIAN_POINT('Origin',(-115.000000000001,250.,-45.1798442476466));
#19835=CARTESIAN_POINT('Ctrl Pts',(-108.033967922038,249.902929948988,-79.9999999999999));
#19836=CARTESIAN_POINT('Ctrl Pts',(-107.058723431124,284.889340141846,-79.9999999999999));
#19837=CARTESIAN_POINT('Ctrl Pts',(-107.058723431124,284.889340141846,-44.9999999999999));
#19838=CARTESIAN_POINT('Ctrl Pts',(-109.754786521379,249.96768639131,-79.9999999999999));
#19839=CARTESIAN_POINT('Ctrl Pts',(-109.104754181425,284.946373149815,-79.9832218312162));
#19840=CARTESIAN_POINT('Ctrl Pts',(-109.707063739997,284.963162499786,-44.9999999999515));
#19841=CARTESIAN_POINT('Ctrl Pts',(-111.474797972355,250.000000000097,-80.0443888208499));
#19842=CARTESIAN_POINT('Ctrl Pts',(-111.151224324472,284.983237668963,-80.027670071346));
#19843=CARTESIAN_POINT('Ctrl Pts',(-112.354160313521,285.,-45.0599248824912));
#19844=CARTESIAN_POINT('Ctrl Pts',(-113.193991683492,250.,-80.1332179612197));
#19845=CARTESIAN_POINT('Ctrl Pts',(-113.193991683492,285.,-80.1332179612197));
#19846=CARTESIAN_POINT('Ctrl Pts',(-115.000000000001,285.,-45.1798442476466));
#19847=CARTESIAN_POINT('Origin',(-108.033967922038,249.902929948988,-44.9999999999999));
#19848=CARTESIAN_POINT('Origin',(-115.,0.,-44.9999999999999));
#19849=CARTESIAN_POINT('Ctrl Pts',(170.,0.,-45.));
#19850=CARTESIAN_POINT('Ctrl Pts',(170.,1.10014726515156,-45.2609231886251));
#19851=CARTESIAN_POINT('Ctrl Pts',(169.99070766613,2.20035818324513,-45.521861500102));
#19852=CARTESIAN_POINT('Ctrl Pts',(169.972146497345,3.29972358349869,-45.7825844101657));
#19853=CARTESIAN_POINT('Ctrl Pts',(169.953585328561,4.39908898375224,-46.0433073202294));
#19854=CARTESIAN_POINT('Ctrl Pts',(169.925755342586,5.4976087048996,-46.303814771838));
#19855=CARTESIAN_POINT('Ctrl Pts',(169.888733367566,6.59437588114246,-46.5638770533837));
#19856=CARTESIAN_POINT('Ctrl Pts',(169.830507889234,8.31929178364157,-46.9728841560716));
#19857=CARTESIAN_POINT('Ctrl Pts',(169.749525512653,10.040940545513,-47.3810433083307));
#19858=CARTESIAN_POINT('Ctrl Pts',(169.645957717126,11.7593577335116,-47.7883060136141));
#19859=CARTESIAN_POINT('Ctrl Pts',(169.617820820864,12.2262106379944,-47.8989495629087));
#19860=CARTESIAN_POINT('Ctrl Pts',(169.588016647507,12.6928250667316,-48.0095269576643));
#19861=CARTESIAN_POINT('Ctrl Pts',(169.556547977067,13.1592018092437,-48.1200372424757));
#19862=CARTESIAN_POINT('Ctrl Pts',(169.439189829893,14.8984907471084,-48.5321703922921));
#19863=CARTESIAN_POINT('Ctrl Pts',(169.298685536974,16.6344752969574,-48.9433703105389));
#19864=CARTESIAN_POINT('Ctrl Pts',(169.13514695613,18.3671801914865,-49.353583556718));
#19865=CARTESIAN_POINT('Ctrl Pts',(168.971189618771,20.1043218461985,-49.7648471939953));
#19866=CARTESIAN_POINT('Ctrl Pts',(168.784079857552,21.8381673450186,-50.1751192500177));
#19867=CARTESIAN_POINT('Ctrl Pts',(168.573878051586,23.5687409239769,-50.5843439701539));
#19868=CARTESIAN_POINT('Ctrl Pts',(168.467429473832,24.44512300515,-50.7915800081133));
#19869=CARTESIAN_POINT('Ctrl Pts',(168.355058055932,25.3206659538579,-50.9985474099555));
#19870=CARTESIAN_POINT('Ctrl Pts',(168.236766577472,26.1953724560961,-51.205238561613));
#19871=CARTESIAN_POINT('Ctrl Pts',(168.005816599942,27.9031323866398,-51.6087783385501));
#19872=CARTESIAN_POINT('Ctrl Pts',(167.752307699827,29.6076802919403,-52.0112562037791));
#19873=CARTESIAN_POINT('Ctrl Pts',(167.476221608132,31.3090471360765,-52.41262057382));
#19874=CARTESIAN_POINT('Ctrl Pts',(167.195655370704,33.0380226560489,-52.8204980241076));
#19875=CARTESIAN_POINT('Ctrl Pts',(166.891773307017,34.7637133896723,-53.2272257253356));
#19876=CARTESIAN_POINT('Ctrl Pts',(166.564503212267,36.4861388550054,-53.6327416763463));
#19877=CARTESIAN_POINT('Ctrl Pts',(166.243285658137,38.1767097443699,-54.0307580060799));
#19878=CARTESIAN_POINT('Ctrl Pts',(165.899536888957,39.8641352719207,-54.4276071116183));
#19879=CARTESIAN_POINT('Ctrl Pts',(165.533140039383,41.5484171429918,-54.8232207088668));
#19880=CARTESIAN_POINT('Ctrl Pts',(165.156387442808,43.2803031268083,-55.2300158278135));
#19881=CARTESIAN_POINT('Ctrl Pts',(164.755688530513,45.0088656611518,-55.6355048330746));
#19882=CARTESIAN_POINT('Ctrl Pts',(164.330865112352,46.7340834604885,-56.0396004742571));
#19883=CARTESIAN_POINT('Ctrl Pts',(163.90604169419,48.4593012598251,-56.4436961154396));
#19884=CARTESIAN_POINT('Ctrl Pts',(163.45709360351,50.1811746454788,-56.8463985627328));
#19885=CARTESIAN_POINT('Ctrl Pts',(162.983793115997,51.8996540346802,-57.247604850381));
#19886=CARTESIAN_POINT('Ctrl Pts',(162.743229120032,52.7731039460092,-57.4515255948328));
#19887=CARTESIAN_POINT('Ctrl Pts',(162.496214958299,53.6462315733819,-57.6551905253493));
#19888=CARTESIAN_POINT('Ctrl Pts',(162.24298557228,54.5180618389271,-57.8583595275675));
#19889=CARTESIAN_POINT('Ctrl Pts',(161.989773057244,55.389834020243,-58.0615149939917));
#19890=CARTESIAN_POINT('Ctrl Pts',(161.730346187712,56.2603088858134,-58.2641745489658));
#19891=CARTESIAN_POINT('Ctrl Pts',(161.464989360853,57.1285269958721,-58.4661036377234));
#19892=CARTESIAN_POINT('Ctrl Pts',(161.351122831121,57.501085653638,-58.5527528672197));
#19893=CARTESIAN_POINT('Ctrl Pts',(161.236165016502,57.8732289727676,-58.6392676671293));
#19894=CARTESIAN_POINT('Ctrl Pts',(161.120141148337,58.2448821043678,-58.7256298498529));
#19895=CARTESIAN_POINT('Ctrl Pts',(160.604746227511,59.8958194448209,-59.109263243839));
#19896=CARTESIAN_POINT('Ctrl Pts',(160.068164227368,61.5375939752252,-59.4900027127986));
#19897=CARTESIAN_POINT('Ctrl Pts',(159.510544723069,63.1702864707303,-59.8677910350757));
#19898=CARTESIAN_POINT('Ctrl Pts',(159.357543388526,63.6182696004155,-59.9714497432759));
#19899=CARTESIAN_POINT('Ctrl Pts',(159.202957931221,64.065568921102,-60.0748862162546));
#19900=CARTESIAN_POINT('Ctrl Pts',(159.046790785211,64.512185956635,-60.1780991408196));
#19901=CARTESIAN_POINT('Ctrl Pts',(158.473786608197,66.1509008427348,-60.5568051517102));
#19902=CARTESIAN_POINT('Ctrl Pts',(157.879492825345,67.7804313129569,-60.9325012513163));
#19903=CARTESIAN_POINT('Ctrl Pts',(157.263999454076,69.400834013756,-61.3051178093134));
#19904=CARTESIAN_POINT('Ctrl Pts',(156.646365385725,71.0268725044679,-61.6790303344413));
#19905=CARTESIAN_POINT('Ctrl Pts',(156.007383843491,72.6437198968175,-62.0498420154008));
#19906=CARTESIAN_POINT('Ctrl Pts',(155.347098296672,74.2514158971068,-62.417468623946));
#19907=CARTESIAN_POINT('Ctrl Pts',(154.999559111842,75.0976215426612,-62.6109677130468));
#19908=CARTESIAN_POINT('Ctrl Pts',(154.646117068505,75.9412915600981,-62.8035841611313));
#19909=CARTESIAN_POINT('Ctrl Pts',(154.286773495438,76.782429413302,-62.9953039280719));
#19910=CARTESIAN_POINT('Ctrl Pts',(153.622311759971,78.3377763280565,-63.3498127007693));
#19911=CARTESIAN_POINT('Ctrl Pts',(152.937691679161,79.8844384046647,-63.7012418382629));
#19912=CARTESIAN_POINT('Ctrl Pts',(152.232871611383,81.4224500704914,-64.0495114541217));
#19913=CARTESIAN_POINT('Ctrl Pts',(151.495567436294,83.0313464035976,-64.4138322979342));
#19914=CARTESIAN_POINT('Ctrl Pts',(150.736158474361,84.6307770714895,-64.7746960106424));
#19915=CARTESIAN_POINT('Ctrl Pts',(149.954550021439,86.2207499804614,-65.1319884530789));
#19916=CARTESIAN_POINT('Ctrl Pts',(149.207970829692,87.7394652461946,-65.4732681589137));
#19917=CARTESIAN_POINT('Ctrl Pts',(148.441136834072,89.249551468873,-65.8112895102483));
#19918=CARTESIAN_POINT('Ctrl Pts',(147.653928142943,90.7509847859831,-66.1459310078955));
#19919=CARTESIAN_POINT('Ctrl Pts',(146.867822914329,92.2503134828016,-66.4801034249128));
#19920=CARTESIAN_POINT('Ctrl Pts',(146.061399808802,93.741013693034,-66.8109055943775));
#19921=CARTESIAN_POINT('Ctrl Pts',(145.234506851664,95.223028803549,-67.1381929309409));
#19922=CARTESIAN_POINT('Ctrl Pts',(144.40981406396,96.7011006172698,-67.4646094321829));
#19923=CARTESIAN_POINT('Ctrl Pts',(143.564759931134,98.1705336376485,-67.787529909235));
#19924=CARTESIAN_POINT('Ctrl Pts',(142.699165309371,99.6312365631214,-68.1067854529431));
#19925=CARTESIAN_POINT('Ctrl Pts',(142.57208263001,99.8456903465111,-68.1536571049555));
#19926=CARTESIAN_POINT('Ctrl Pts',(142.444557159281,100.059955890433,-68.2004497132391));
#19927=CARTESIAN_POINT('Ctrl Pts',(142.316588284338,100.274032839058,-68.247162694269));
#19928=CARTESIAN_POINT('Ctrl Pts',(141.487458133348,101.661070529399,-68.5498233297682));
#19929=CARTESIAN_POINT('Ctrl Pts',(140.639691681384,103.040221704901,-68.8491578079982));
#19930=CARTESIAN_POINT('Ctrl Pts',(139.77305998302,104.411420051739,-69.1450170053095));
#19931=CARTESIAN_POINT('Ctrl Pts',(139.453130089157,104.917618177652,-69.2542377986095));
#19932=CARTESIAN_POINT('Ctrl Pts',(139.130628954756,105.422732104968,-69.362984704975));
#19933=CARTESIAN_POINT('Ctrl Pts',(138.805544276616,105.926757191782,-69.4712492655195));
#19934=CARTESIAN_POINT('Ctrl Pts',(138.20270440341,106.861425725427,-69.6720160144317));
#19935=CARTESIAN_POINT('Ctrl Pts',(137.591646601873,107.79130568966,-69.8709000606912));
#19936=CARTESIAN_POINT('Ctrl Pts',(136.972927262067,108.715551339406,-70.0676789932748));
#19937=CARTESIAN_POINT('Ctrl Pts',(136.354207922262,109.639796989153,-70.2644579258585));
#19938=CARTESIAN_POINT('Ctrl Pts',(135.727827192656,110.558408197228,-70.4591316805119));
#19939=CARTESIAN_POINT('Ctrl Pts',(135.094388092976,111.470576450946,-70.6514912337012));
#19940=CARTESIAN_POINT('Ctrl Pts',(134.118891433214,112.875316204291,-70.9477250811292));
#19941=CARTESIAN_POINT('Ctrl Pts',(133.125836160857,114.265989764737,-71.2387250091251));
#19942=CARTESIAN_POINT('Ctrl Pts',(132.115279202864,115.642677372998,-71.5243588974733));
#19943=CARTESIAN_POINT('Ctrl Pts',(131.100057726306,117.025719481967,-71.8113112118284));
#19944=CARTESIAN_POINT('Ctrl Pts',(130.067172320333,118.394646372545,-72.0928479988192));
#19945=CARTESIAN_POINT('Ctrl Pts',(129.01664787406,119.74950996065,-72.3688065526259));
#19946=CARTESIAN_POINT('Ctrl Pts',(128.396773300342,120.54896350226,-72.5316392135045));
#19947=CARTESIAN_POINT('Ctrl Pts',(127.770756687264,121.34352001057,-72.6925291275462));
#19948=CARTESIAN_POINT('Ctrl Pts',(127.138598490159,122.133185094108,-72.851437859478));
#19949=CARTESIAN_POINT('Ctrl Pts',(126.121677576623,123.403479368257,-73.107066298032));
#19950=CARTESIAN_POINT('Ctrl Pts',(125.08890734821,124.66109427067,-73.3575491477337));
#19951=CARTESIAN_POINT('Ctrl Pts',(124.040215967679,125.906056570587,-73.6027362667229));
#19952=CARTESIAN_POINT('Ctrl Pts',(122.990840610091,127.151830859297,-73.848083301553));
#19953=CARTESIAN_POINT('Ctrl Pts',(121.92552299743,128.384936090349,-74.0881278349307));
#19954=CARTESIAN_POINT('Ctrl Pts',(120.844170049389,129.605365540767,-74.3226855021703));
#19955=CARTESIAN_POINT('Ctrl Pts',(119.763137083678,130.825433854834,-74.5571737616287));
#19956=CARTESIAN_POINT('Ctrl Pts',(118.66607793164,132.03283390954,-74.7861785321864));
#19957=CARTESIAN_POINT('Ctrl Pts',(117.552883524561,133.22752491456,-75.009479697586));
#19958=CARTESIAN_POINT('Ctrl Pts',(116.440807254544,134.42101592407,-75.2325565703488));
#19959=CARTESIAN_POINT('Ctrl Pts',(115.312627779448,135.601823387615,-75.4499414111029));
#19960=CARTESIAN_POINT('Ctrl Pts',(114.16822546943,136.769872585367,-75.6613770385435));
#19961=CARTESIAN_POINT('Ctrl Pts',(113.026415571553,137.935275803733,-75.8723337013029));
#19962=CARTESIAN_POINT('Ctrl Pts',(111.868455902192,139.087978438965,-76.0773681795067));
#19963=CARTESIAN_POINT('Ctrl Pts',(110.694222039097,140.227872886939,-76.2761857732088));
#19964=CARTESIAN_POINT('Ctrl Pts',(110.16402252702,140.742567190288,-76.3659574911657));
#19965=CARTESIAN_POINT('Ctrl Pts',(109.63050502821,141.25464974426,-76.4544611843318));
#19966=CARTESIAN_POINT('Ctrl Pts',(109.093658009703,141.764108460991,-76.5416670048306));
#19967=CARTESIAN_POINT('Ctrl Pts',(108.281664476563,142.534676554184,-76.6735678254667));
#19968=CARTESIAN_POINT('Ctrl Pts',(107.461568433179,143.299677084708,-76.80258103617));
#19969=CARTESIAN_POINT('Ctrl Pts',(106.634043305536,144.058369920031,-76.9284826090685));
#19970=CARTESIAN_POINT('Ctrl Pts',(105.806518177894,144.817062755354,-77.054384181967));
#19971=CARTESIAN_POINT('Ctrl Pts',(104.971564130646,145.569447788168,-77.1771740451513));
#19972=CARTESIAN_POINT('Ctrl Pts',(104.129891430385,146.314830427712,-77.2966438182492));
#19973=CARTESIAN_POINT('Ctrl Pts',(102.881043322562,147.420806300174,-77.473909399073));
#19974=CARTESIAN_POINT('Ctrl Pts',(101.619608187914,148.509435764892,-77.643559231171));
#19975=CARTESIAN_POINT('Ctrl Pts',(100.345654535066,149.580844722008,-77.8053456962242));
#19976=CARTESIAN_POINT('Ctrl Pts',(99.9024225601615,149.953607661172,-77.8616341916949));
#19977=CARTESIAN_POINT('Ctrl Pts',(99.4576751258032,150.324285878761,-77.9169704642455));
#19978=CARTESIAN_POINT('Ctrl Pts',(99.011414756953,150.692883965256,-77.971342843451));
#19979=CARTESIAN_POINT('Ctrl Pts',(97.7693082210675,151.718827840867,-78.1226811479409));
#19980=CARTESIAN_POINT('Ctrl Pts',(96.5154925721465,152.728661615878,-78.2665514875638));
#19981=CARTESIAN_POINT('Ctrl Pts',(95.2499812988189,153.722453132978,-78.4026874034882));
#19982=CARTESIAN_POINT('Ctrl Pts',(93.9839970223882,154.716616094001,-78.538874202176));
#19983=CARTESIAN_POINT('Ctrl Pts',(92.7063079976469,155.694724630978,-78.6673208962488));
#19984=CARTESIAN_POINT('Ctrl Pts',(91.416924495997,156.656823856401,-78.7877139697859));
#19985=CARTESIAN_POINT('Ctrl Pts',(90.4071022541114,157.410322870069,-78.8820036851973));
#19986=CARTESIAN_POINT('Ctrl Pts',(89.3901067970427,158.154001691191,-78.9713526037555));
#19987=CARTESIAN_POINT('Ctrl Pts',(88.3659439434344,158.887873384098,-79.0555895260508));
#19988=CARTESIAN_POINT('Ctrl Pts',(87.1437413180917,159.763651983738,-79.1561151282217));
#19989=CARTESIAN_POINT('Ctrl Pts',(85.9113392665142,160.62546502764,-79.2493608525903));
#19990=CARTESIAN_POINT('Ctrl Pts',(84.6686824263498,161.473300644551,-79.3350129070214));
#19991=CARTESIAN_POINT('Ctrl Pts',(83.4331570535623,162.316270628531,-79.4201734139776));
#19992=CARTESIAN_POINT('Ctrl Pts',(82.1874939418069,163.145422894328,-79.497827189361));
#19993=CARTESIAN_POINT('Ctrl Pts',(80.9316483599466,163.960729856028,-79.5676180305605));
#19994=CARTESIAN_POINT('Ctrl Pts',(79.689772071307,164.766967818978,-79.6366325591792));
#19995=CARTESIAN_POINT('Ctrl Pts',(78.4379383029592,165.55966648192,-79.6979580775793));
#19996=CARTESIAN_POINT('Ctrl Pts',(77.1761176725809,166.338787716879,-79.751203332978));
#19997=CARTESIAN_POINT('Ctrl Pts',(76.0053484983634,167.061688502386,-79.8006064749092));
#19998=CARTESIAN_POINT('Ctrl Pts',(74.8259920696566,167.772903562918,-79.8430528496191));
#19999=CARTESIAN_POINT('Ctrl Pts',(73.6379472668019,168.472368248304,-79.8781987072658));
#20000=CARTESIAN_POINT('Ctrl Pts',(72.4567121022887,169.167823740157,-79.9131431157927));
#20001=CARTESIAN_POINT('Ctrl Pts',(71.2668876275958,169.851662875256,-79.9408704679589));
#20002=CARTESIAN_POINT('Ctrl Pts',(70.0683926518377,170.523813905937,-79.9609955712169));
#20003=CARTESIAN_POINT('Ctrl Pts',(68.8812223363898,171.189613735943,-79.9809305110094));
#20004=CARTESIAN_POINT('Ctrl Pts',(67.6855443847963,171.843944978397,-79.9934061572428));
#20005=CARTESIAN_POINT('Ctrl Pts',(66.481301251357,172.486734441791,-79.9980017915023));
#20006=CARTESIAN_POINT('Ctrl Pts',(66.1331776656422,172.672552543338,-79.9993303011966));
#20007=CARTESIAN_POINT('Ctrl Pts',(65.7843384560529,172.857406119814,-80.));
#20008=CARTESIAN_POINT('Ctrl Pts',(65.4347826086956,173.041293409847,-80.));
#20009=CARTESIAN_POINT('Origin',(3.92135447228745,250.,28.0096748020596));
#20010=CARTESIAN_POINT('Origin',(-126.751426934183,250.,46.3038641989655));
#20011=CARTESIAN_POINT('Origin',(-108.033967922038,250.,180.));
#20012=CARTESIAN_POINT('Origin',(-115.000000000001,250.,45.1798442476468));
#20013=CARTESIAN_POINT('Ctrl Pts',(-113.193991683492,250.,80.1332179612198));
#20014=CARTESIAN_POINT('Ctrl Pts',(-113.193991683492,285.,80.1332179612198));
#20015=CARTESIAN_POINT('Ctrl Pts',(-115.000000000001,285.,45.1798442476468));
#20016=CARTESIAN_POINT('Ctrl Pts',(-111.474797972362,250.000000000097,80.0443888208503));
#20017=CARTESIAN_POINT('Ctrl Pts',(-111.151224324474,284.983237668963,80.0276700713582));
#20018=CARTESIAN_POINT('Ctrl Pts',(-112.354160313515,285.,45.0599248825255));
#20019=CARTESIAN_POINT('Ctrl Pts',(-109.754786521371,249.967686391406,80.0000000000001));
#20020=CARTESIAN_POINT('Ctrl Pts',(-109.104754181423,284.946373149817,79.9832218311837));
#20021=CARTESIAN_POINT('Ctrl Pts',(-109.707063740001,284.963162499787,44.9999999999839));
#20022=CARTESIAN_POINT('Ctrl Pts',(-108.033967922038,249.902929948988,80.0000000000001));
#20023=CARTESIAN_POINT('Ctrl Pts',(-107.058723431124,284.889340141846,80.0000000000001));
#20024=CARTESIAN_POINT('Ctrl Pts',(-107.058723431124,284.889340141846,45.0000000000001));
#20025=CARTESIAN_POINT('Origin',(-108.033967922038,249.902929948988,45.0000000000001));
#20026=CARTESIAN_POINT('Origin',(-115.,0.,45.0000000000001));
#20027=CARTESIAN_POINT('Ctrl Pts',(65.4347826086958,173.041293409847,80.));
#20028=CARTESIAN_POINT('Ctrl Pts',(66.6461323784681,172.404050954516,80.));
#20029=CARTESIAN_POINT('Ctrl Pts',(67.8488741821648,171.755204325261,79.9919611843668));
#20030=CARTESIAN_POINT('Ctrl Pts',(69.0430590209991,171.094827191335,79.9763199823015));
#20031=CARTESIAN_POINT('Ctrl Pts',(70.2450844944289,170.430114232975,79.9605760851207));
#20032=CARTESIAN_POINT('Ctrl Pts',(71.4384404980377,169.753719199296,79.9371296605925));
#20033=CARTESIAN_POINT('Ctrl Pts',(72.6232020546047,169.065715093842,79.9063781002701));
#20034=CARTESIAN_POINT('Ctrl Pts',(73.8175810187664,168.372126053704,79.8753769114143));
#20035=CARTESIAN_POINT('Ctrl Pts',(75.0032256809894,167.666739016059,79.8369515176592));
#20036=CARTESIAN_POINT('Ctrl Pts',(76.1802326477079,166.949621683208,79.7914605218376));
#20037=CARTESIAN_POINT('Ctrl Pts',(76.5129016171382,166.746935810629,79.7786029575867));
#20038=CARTESIAN_POINT('Ctrl Pts',(76.8448806696896,166.543312801713,79.7651806603313));
#20039=CARTESIAN_POINT('Ctrl Pts',(77.1761722268184,166.338754031917,79.7512010309385));
#20040=CARTESIAN_POINT('Ctrl Pts',(78.4502335131952,165.552074130852,79.6974390070534));
#20041=CARTESIAN_POINT('Ctrl Pts',(79.7141132075376,164.751552111255,79.6354392698203));
#20042=CARTESIAN_POINT('Ctrl Pts',(80.967841633028,163.937227172555,79.5656043347192));
#20043=CARTESIAN_POINT('Ctrl Pts',(82.2296315257554,163.117666128747,79.4953203613495));
#20044=CARTESIAN_POINT('Ctrl Pts',(83.4811394894385,162.284124393098,79.4171000956569));
#20045=CARTESIAN_POINT('Ctrl Pts',(84.7224110600106,161.436629785652,79.3313044021991));
#20046=CARTESIAN_POINT('Ctrl Pts',(85.9469000979227,160.600593674691,79.2466687039122));
#20047=CARTESIAN_POINT('Ctrl Pts',(87.1614280078243,159.750979641084,79.1546608597167));
#20048=CARTESIAN_POINT('Ctrl Pts',(88.3660478508558,158.887798928392,79.0555809796938));
#20049=CARTESIAN_POINT('Ctrl Pts',(89.6734044670519,157.951001296975,78.9480510087828));
#20050=CARTESIAN_POINT('Ctrl Pts',(90.9690817922079,156.998223705516,78.8321926827009));
#20051=CARTESIAN_POINT('Ctrl Pts',(92.2530681368108,156.0294369149,78.7083568595487));
#20052=CARTESIAN_POINT('Ctrl Pts',(93.5372691533739,155.060488151098,78.584500332065));
#20053=CARTESIAN_POINT('Ctrl Pts',(94.8097756557245,154.075525043431,78.4526635519813));
#20054=CARTESIAN_POINT('Ctrl Pts',(96.0705771572415,153.074497779078,78.3131497015861));
#20055=CARTESIAN_POINT('Ctrl Pts',(97.058088528114,152.290452229549,78.2038767403042));
#20056=CARTESIAN_POINT('Ctrl Pts',(98.0384193587957,151.496551473984,78.0898931912743));
#20057=CARTESIAN_POINT('Ctrl Pts',(99.0115628561522,150.692761639502,77.9713247989972));
#20058=CARTESIAN_POINT('Ctrl Pts',(100.294220382482,149.633321707378,77.8150450302352));
#20059=CARTESIAN_POINT('Ctrl Pts',(101.564380068726,148.556699124926,77.6508055324762));
#20060=CARTESIAN_POINT('Ctrl Pts',(102.821978092576,147.462776792109,77.4788690746293));
#20061=CARTESIAN_POINT('Ctrl Pts',(103.259527029588,147.082174608566,77.4190481994867));
#20062=CARTESIAN_POINT('Ctrl Pts',(103.695555249051,146.69947804494,77.3582952087644));
#20063=CARTESIAN_POINT('Ctrl Pts',(104.130059658361,146.314681445384,77.2966199393637));
#20064=CARTESIAN_POINT('Ctrl Pts',(104.971735602031,145.569294208538,77.1771491366246));
#20065=CARTESIAN_POINT('Ctrl Pts',(105.806692611071,144.816904703943,77.0543582486579));
#20066=CARTESIAN_POINT('Ctrl Pts',(106.634220566184,144.058207403801,76.9284556400773));
#20067=CARTESIAN_POINT('Ctrl Pts',(107.461748521298,143.299510103659,76.8025530314967));
#20068=CARTESIAN_POINT('Ctrl Pts',(108.281847257875,142.534505115263,76.6735387741947));
#20069=CARTESIAN_POINT('Ctrl Pts',(109.093843490683,141.763932442456,76.5416368750921));
#20070=CARTESIAN_POINT('Ctrl Pts',(110.282654488823,140.635768011038,76.3485246142302));
#20071=CARTESIAN_POINT('Ctrl Pts',(111.455138482761,139.494739173689,76.1490506803267));
#20072=CARTESIAN_POINT('Ctrl Pts',(112.611420646104,138.340968291007,75.9435279501095));
#20073=CARTESIAN_POINT('Ctrl Pts',(113.769896451987,137.185008530064,75.7376153121186));
#20074=CARTESIAN_POINT('Ctrl Pts',(114.912109249862,136.016258399039,75.5256307997759));
#20075=CARTESIAN_POINT('Ctrl Pts',(116.038181686695,134.834807735391,75.307848804401));
#20076=CARTESIAN_POINT('Ctrl Pts',(117.166182792069,133.651333554735,75.0896938052392));
#20077=CARTESIAN_POINT('Ctrl Pts',(118.277988553096,132.455115332012,74.8657213326374));
#20078=CARTESIAN_POINT('Ctrl Pts',(119.373713676575,131.246209304145,74.636168474289));
#20079=CARTESIAN_POINT('Ctrl Pts',(120.46960611424,130.037118679682,74.406580563856));
#20080=CARTESIAN_POINT('Ctrl Pts',(121.549413346339,128.815336367242,74.1714104337045));
#20081=CARTESIAN_POINT('Ctrl Pts',(122.613236345249,127.580884409607,73.9308584323559));
#20082=CARTESIAN_POINT('Ctrl Pts',(123.676359826661,126.347244166651,73.6904646061305));
#20083=CARTESIAN_POINT('Ctrl Pts',(124.723520420591,125.100950892824,73.444695846114));
#20084=CARTESIAN_POINT('Ctrl Pts',(125.75480007494,123.841992797908,73.1937173237016));
#20085=CARTESIAN_POINT('Ctrl Pts',(126.219366288216,123.274863026308,73.0806576494622));
#20086=CARTESIAN_POINT('Ctrl Pts',(126.680709527289,122.705162753967,72.966540311257));
#20087=CARTESIAN_POINT('Ctrl Pts',(127.138835761371,122.13288870443,72.8513782152747));
#20088=CARTESIAN_POINT('Ctrl Pts',(128.210661006918,120.794004946999,72.5819467079277));
#20089=CARTESIAN_POINT('Ctrl Pts',(129.264832288659,119.441061318821,72.3068215265784));
#20090=CARTESIAN_POINT('Ctrl Pts',(130.301341770802,118.074024048082,72.0261836067221));
#20091=CARTESIAN_POINT('Ctrl Pts',(131.333339219409,116.712937632707,71.7467673329075));
#20092=CARTESIAN_POINT('Ctrl Pts',(132.347828610888,115.337879883744,71.461886051324));
#20093=CARTESIAN_POINT('Ctrl Pts',(133.344772650024,113.948787359142,71.171688683276));
#20094=CARTESIAN_POINT('Ctrl Pts',(133.934200329062,113.127507978754,71.0001139966372));
#20095=CARTESIAN_POINT('Ctrl Pts',(134.517494302768,112.30132206452,70.8266804775351));
#20096=CARTESIAN_POINT('Ctrl Pts',(135.094641307937,111.470211814142,70.6514143384368));
#20097=CARTESIAN_POINT('Ctrl Pts',(135.728081448236,110.558037638606,70.4590532818156));
#20098=CARTESIAN_POINT('Ctrl Pts',(136.354463262642,109.639420272454,70.2643779700071));
#20099=CARTESIAN_POINT('Ctrl Pts',(136.97318350466,108.715168561764,70.067597497168));
#20100=CARTESIAN_POINT('Ctrl Pts',(137.591903746677,107.790916851074,69.8708170243288));
#20101=CARTESIAN_POINT('Ctrl Pts',(138.20296226777,106.861030923092,69.6719314547462));
#20102=CARTESIAN_POINT('Ctrl Pts',(138.805802472581,105.926356872724,69.4711632769561));
#20103=CARTESIAN_POINT('Ctrl Pts',(139.686395610747,104.561040577283,69.1778930565674));
#20104=CARTESIAN_POINT('Ctrl Pts',(140.548033055148,103.18773742639,68.8810855487316));
#20105=CARTESIAN_POINT('Ctrl Pts',(141.39095234604,101.806527636459,68.5809000334162));
#20106=CARTESIAN_POINT('Ctrl Pts',(141.702131618801,101.29662845322,68.4700809889848));
#20107=CARTESIAN_POINT('Ctrl Pts',(142.010759658666,100.785651337718,68.358801298185));
#20108=CARTESIAN_POINT('Ctrl Pts',(142.316847597481,100.273599037248,68.2470680358434));
#20109=CARTESIAN_POINT('Ctrl Pts',(143.188689922049,98.8151003140736,67.9288137865961));
#20110=CARTESIAN_POINT('Ctrl Pts',(144.039953118992,97.3478506960236,67.6068657481795));
#20111=CARTESIAN_POINT('Ctrl Pts',(144.870820280825,95.8719469048255,67.2813968647469));
#20112=CARTESIAN_POINT('Ctrl Pts',(145.744966077093,94.3191654807479,66.9389747913547));
#20113=CARTESIAN_POINT('Ctrl Pts',(146.596536296559,92.7568049920601,66.5926556152579));
#20114=CARTESIAN_POINT('Ctrl Pts',(147.425710892994,91.1849357183585,66.242609978645));
#20115=CARTESIAN_POINT('Ctrl Pts',(148.217312758539,89.6842932061474,65.9084261045126));
#20116=CARTESIAN_POINT('Ctrl Pts',(148.988502674307,88.1749836666552,65.5708454866793));
#20117=CARTESIAN_POINT('Ctrl Pts',(149.739404058878,86.6570340611208,65.2299920279374));
#20118=CARTESIAN_POINT('Ctrl Pts',(150.490623793833,85.1384409092449,64.8889940617655));
#20119=CARTESIAN_POINT('Ctrl Pts',(151.221538035357,83.6112001634024,64.5447203357147));
#20120=CARTESIAN_POINT('Ctrl Pts',(151.932234113087,82.0753083209362,64.197273065751));
#20121=CARTESIAN_POINT('Ctrl Pts',(152.642725551019,80.5398587274236,63.8499258407172));
#20122=CARTESIAN_POINT('Ctrl Pts',(153.333010691149,78.9957627989489,63.4994067527238));
#20123=CARTESIAN_POINT('Ctrl Pts',(154.003137062145,77.4429897178712,63.145798278425));
#20124=CARTESIAN_POINT('Ctrl Pts',(154.098169966934,77.2227856746341,63.0956518554142));
#20125=CARTESIAN_POINT('Ctrl Pts',(154.192797389382,77.0024070831775,63.0454432714742));
#20126=CARTESIAN_POINT('Ctrl Pts',(154.287019396353,76.7818538151815,62.995172732479));
#20127=CARTESIAN_POINT('Ctrl Pts',(154.969920185579,75.1833312871433,62.6308227057908));
#20128=CARTESIAN_POINT('Ctrl Pts',(155.631509575676,73.5756648494386,62.2632351988744));
#20129=CARTESIAN_POINT('Ctrl Pts',(156.271767918129,71.9588255780039,61.8925027191992));
#20130=CARTESIAN_POINT('Ctrl Pts',(156.90994347294,70.3472459535393,61.5229762480604));
#20131=CARTESIAN_POINT('Ctrl Pts',(157.52692671005,68.7265528117573,61.1503250777792));
#20132=CARTESIAN_POINT('Ctrl Pts',(158.122652620036,67.0966980818089,60.774625906449));
#20133=CARTESIAN_POINT('Ctrl Pts',(158.436687411552,66.2375259663423,60.5765774264958));
#20134=CARTESIAN_POINT('Ctrl Pts',(158.744814366495,65.3758076965917,60.3776817221769));
#20135=CARTESIAN_POINT('Ctrl Pts',(159.047018599036,64.5115344360402,60.1779485747607));
#20136=CARTESIAN_POINT('Ctrl Pts',(159.616169765598,62.8838201901668,59.8017845717057));
#20137=CARTESIAN_POINT('Ctrl Pts',(160.164315738842,61.2470442552432,59.4226520428314));
#20138=CARTESIAN_POINT('Ctrl Pts',(160.691320701882,59.6011287064151,59.0406108572493));
#20139=CARTESIAN_POINT('Ctrl Pts',(160.835925898711,59.1495049863498,58.9357823552198));
#20140=CARTESIAN_POINT('Ctrl Pts',(160.978939094884,58.6971930807887,58.8307348028855));
#20141=CARTESIAN_POINT('Ctrl Pts',(161.12035681976,58.2441912509891,58.7254693140811));
#20142=CARTESIAN_POINT('Ctrl Pts',(161.390759200204,57.3780143044214,58.5241929975773));
#20143=CARTESIAN_POINT('Ctrl Pts',(161.65536766827,56.5091739433876,58.3220873619862));
#20144=CARTESIAN_POINT('Ctrl Pts',(161.913876783448,55.6386225203367,58.1193844025833));
#20145=CARTESIAN_POINT('Ctrl Pts',(162.172378437343,54.7680962237895,57.9166872937441));
#20146=CARTESIAN_POINT('Ctrl Pts',(162.424781040467,53.8958590880924,57.7133929440505));
#20147=CARTESIAN_POINT('Ctrl Pts',(162.6708283902,53.0228796342858,57.5097391548275));
#20148=CARTESIAN_POINT('Ctrl Pts',(162.776391719317,52.6483394594182,57.4223642166254));
#20149=CARTESIAN_POINT('Ctrl Pts',(162.880785841691,52.2736628366288,57.3349231841326));
#20150=CARTESIAN_POINT('Ctrl Pts',(162.983993330494,51.898927081956,57.2474351316884));
#20151=CARTESIAN_POINT('Ctrl Pts',(163.44181462992,50.236625129495,56.8593441673714));
#20152=CARTESIAN_POINT('Ctrl Pts',(163.876849494941,48.5711473098526,56.4698531943719));
#20153=CARTESIAN_POINT('Ctrl Pts',(164.289304748925,46.9025389459629,56.0790556533708));
#20154=CARTESIAN_POINT('Ctrl Pts',(164.712616410982,45.1900104401014,55.6779717660619));
#20155=CARTESIAN_POINT('Ctrl Pts',(165.112144521505,43.4741842389034,55.2755115308422));
#20156=CARTESIAN_POINT('Ctrl Pts',(165.488065228237,41.7550820886685,54.8717608318544));
#20157=CARTESIAN_POINT('Ctrl Pts',(165.856698167564,40.06930722366,54.4758374249816));
#20158=CARTESIAN_POINT('Ctrl Pts',(166.2026301339,38.3803818300019,54.078672912382));
#20159=CARTESIAN_POINT('Ctrl Pts',(166.525980271794,36.688304964299,53.6803362266353));
#20160=CARTESIAN_POINT('Ctrl Pts',(166.858919218813,34.9460502876389,53.2701870379699));
#20161=CARTESIAN_POINT('Ctrl Pts',(167.167917546405,33.2004542212604,52.8587950132626));
#20162=CARTESIAN_POINT('Ctrl Pts',(167.453051830328,31.4514970984036,52.4462246664667));
#20163=CARTESIAN_POINT('Ctrl Pts',(167.738186114251,29.7025399755469,52.0336543196709));
#20164=CARTESIAN_POINT('Ctrl Pts',(167.999456457707,27.9502214508155,51.6199054808393));
#20165=CARTESIAN_POINT('Ctrl Pts',(168.236883475619,26.1945080380638,51.2050343015782));
#20166=CARTESIAN_POINT('Ctrl Pts',(168.470502966904,24.4669503323876,50.7968162533534));
#20167=CARTESIAN_POINT('Ctrl Pts',(168.681033417607,22.7361302648766,50.3875209152059));
#20168=CARTESIAN_POINT('Ctrl Pts',(168.86844066887,21.0020257404361,49.9772058899181));
#20169=CARTESIAN_POINT('Ctrl Pts',(169.055408494949,19.2719872763818,49.5678529552349));
#20170=CARTESIAN_POINT('Ctrl Pts',(169.21936146439,17.5386794258596,49.1574849600718));
#20171=CARTESIAN_POINT('Ctrl Pts',(169.360214013948,15.8020771827112,48.7461560842687));
#20172=CARTESIAN_POINT('Ctrl Pts',(169.431623414445,14.9216548866687,48.537620644048));
#20173=CARTESIAN_POINT('Ctrl Pts',(169.497094521659,14.0403858180888,48.328838195924));
#20174=CARTESIAN_POINT('Ctrl Pts',(169.556611063575,13.1582668116683,48.1198156901436));
#20175=CARTESIAN_POINT('Ctrl Pts',(169.672434204295,11.4416046783918,47.7130440209424));
#20176=CARTESIAN_POINT('Ctrl Pts',(169.765709655592,9.72172177919562,47.3053630211217));
#20177=CARTESIAN_POINT('Ctrl Pts',(169.836279969576,7.99858073586123,46.8968207381216));
#20178=CARTESIAN_POINT('Ctrl Pts',(169.855452850521,7.5304295231175,46.7858260137005));
#20179=CARTESIAN_POINT('Ctrl Pts',(169.872949511331,7.06203785414009,46.6747677241711));
#20180=CARTESIAN_POINT('Ctrl Pts',(169.888766135311,6.59340507295846,46.5636468581297));
#20181=CARTESIAN_POINT('Ctrl Pts',(169.9257828563,5.49663189754684,46.3035831366046));
#20182=CARTESIAN_POINT('Ctrl Pts',(169.953598091479,4.39853740250482,46.0431764899174));
#20183=CARTESIAN_POINT('Ctrl Pts',(169.972156850062,3.29911036932559,45.782438961203));
#20184=CARTESIAN_POINT('Ctrl Pts',(169.981436229354,2.74939685273598,45.6520701968457));
#20185=CARTESIAN_POINT('Ctrl Pts',(169.988401335714,2.19927120329341,45.5215999770967));
#20186=CARTESIAN_POINT('Ctrl Pts',(169.993042478652,1.64921227805479,45.3911437233179));
#20187=CARTESIAN_POINT('Ctrl Pts',(169.995363050121,1.37418281543549,45.3259155964285));
#20188=CARTESIAN_POINT('Ctrl Pts',(169.997103130708,1.09914979647015,45.2606861617961));
#20189=CARTESIAN_POINT('Ctrl Pts',(169.998262721974,0.824113169007625,45.1954556393542));
#20190=CARTESIAN_POINT('Ctrl Pts',(169.999310371452,0.575627355555245,45.1365221817255));
#20191=CARTESIAN_POINT('Ctrl Pts',(169.999884019389,0.326147221333698,45.0773527091105));
#20192=CARTESIAN_POINT('Ctrl Pts',(169.999983994202,0.0791027940534806,
45.0187609002855));
#20193=CARTESIAN_POINT('Ctrl Pts',(169.999994676552,0.0527059927639873,
45.0125003407911));
#20194=CARTESIAN_POINT('Ctrl Pts',(170.,0.0263369999825807,45.0062463764957));
#20195=CARTESIAN_POINT('Ctrl Pts',(170.,3.49024337756996E-14,45.));
#20196=CARTESIAN_POINT('Ctrl Pts',(65.4171737766276,173.051051117154,79.9999995059578));
#20197=CARTESIAN_POINT('Ctrl Pts',(60.1122246678144,159.017358945106,79.9970990772669));
#20198=CARTESIAN_POINT('Ctrl Pts',(60.1111292806026,159.017773023373,94.9999991814784));
#20199=CARTESIAN_POINT('Ctrl Pts',(69.4980654230037,170.904781366711,80.0002461066156));
#20200=CARTESIAN_POINT('Ctrl Pts',(63.9530125618426,157.565452095818,80.5517562050311));
#20201=CARTESIAN_POINT('Ctrl Pts',(64.2759055369405,157.443423435057,95.0003752334648));
#20202=CARTESIAN_POINT('Ctrl Pts',(73.4707404887855,168.632425582207,79.9097827742579));
#20203=CARTESIAN_POINT('Ctrl Pts',(67.8395215153769,155.937211445011,80.9562032488646));
#20204=CARTESIAN_POINT('Ctrl Pts',(68.3475774635587,155.717622842009,94.8711639053697));
#20205=CARTESIAN_POINT('Ctrl Pts',(81.2094588046944,163.843390610061,79.5786121468522));
#20206=CARTESIAN_POINT('Ctrl Pts',(75.4920654363854,152.377267497421,81.4803629792958));
#20207=CARTESIAN_POINT('Ctrl Pts',(76.3074783717929,151.97526765444,94.3981030531638));
#20208=CARTESIAN_POINT('Ctrl Pts',(84.9757899122008,161.327031171744,79.3379637809786));
#20209=CARTESIAN_POINT('Ctrl Pts',(79.2729405826562,150.450643097299,81.6101590419467));
#20210=CARTESIAN_POINT('Ctrl Pts',(80.1959679691824,149.959099180759,94.0543379213307));
#20211=CARTESIAN_POINT('Ctrl Pts',(92.3178906398677,156.046341834353,78.726584215355));
#20212=CARTESIAN_POINT('Ctrl Pts',(86.703867958156,146.292589569395,81.6312588050202));
#20213=CARTESIAN_POINT('Ctrl Pts',(87.8000684551384,145.63747005799,93.1809712877857));
#20214=CARTESIAN_POINT('Ctrl Pts',(95.8936351170506,153.282013829614,78.3557679502871));
#20215=CARTESIAN_POINT('Ctrl Pts',(90.366568547758,144.064645410308,81.5291707439827));
#20216=CARTESIAN_POINT('Ctrl Pts',(91.5156662167517,143.332003833601,92.6512484049633));
#20217=CARTESIAN_POINT('Ctrl Pts',(101.118204191116,148.945321347681,77.7118506792732));
#20218=CARTESIAN_POINT('Ctrl Pts',(95.7862627827622,140.469122843766,81.2184413297099));
#20219=CARTESIAN_POINT('Ctrl Pts',(96.9597420465698,139.655302598131,91.7313856490923));
#20220=CARTESIAN_POINT('Ctrl Pts',(102.836519125185,147.468018930124,77.482549849181));
#20221=CARTESIAN_POINT('Ctrl Pts',(97.565644447969,139.240074537784,81.090445307719));
#20222=CARTESIAN_POINT('Ctrl Pts',(98.7528522876237,138.393276733981,91.4038190221291));
#20223=CARTESIAN_POINT('Ctrl Pts',(106.226989159944,144.448761853408,76.995800971589));
#20224=CARTESIAN_POINT('Ctrl Pts',(101.08836341206,136.704210075211,80.7859435362935));
#20225=CARTESIAN_POINT('Ctrl Pts',(102.295631429104,135.795539951172,90.7084745843325));
#20226=CARTESIAN_POINT('Ctrl Pts',(107.890968873499,142.914010809927,76.7395043574806));
#20227=CARTESIAN_POINT('Ctrl Pts',(102.824700615765,135.403548235755,80.6106070677653));
#20228=CARTESIAN_POINT('Ctrl Pts',(104.036759724697,134.466015015203,90.3423416598691));
#20229=CARTESIAN_POINT('Ctrl Pts',(112.780952654854,138.245372609845,75.9362630272676));
#20230=CARTESIAN_POINT('Ctrl Pts',(107.914041409476,131.435704892851,80.0241711268571));
#20231=CARTESIAN_POINT('Ctrl Pts',(109.159801879539,130.396180641736,89.194868194963));
#20232=CARTESIAN_POINT('Ctrl Pts',(115.910241252279,135.042722467798,75.3543730521059));
#20233=CARTESIAN_POINT('Ctrl Pts',(111.217729890296,128.654798675575,79.5479025767146));
#20234=CARTESIAN_POINT('Ctrl Pts',(112.446820922398,127.570888947572,88.3636043218873));
#20235=CARTESIAN_POINT('Ctrl Pts',(121.921081660961,128.457279192248,74.1087295936706));
#20236=CARTESIAN_POINT('Ctrl Pts',(117.585782041987,122.859192470861,78.4483848144859));
#20237=CARTESIAN_POINT('Ctrl Pts',(118.773955284971,121.701958851907,86.5841254177092));
#20238=CARTESIAN_POINT('Ctrl Pts',(124.802595831012,125.07448269568,73.4449368880087));
#20239=CARTESIAN_POINT('Ctrl Pts',(120.661020346731,119.8431662431,77.8267940081951));
#20240=CARTESIAN_POINT('Ctrl Pts',(121.814041889375,118.658306100492,85.6358543716459));
#20241=CARTESIAN_POINT('Ctrl Pts',(130.325562286974,118.125822190644,72.0427084253293));
#20242=CARTESIAN_POINT('Ctrl Pts',(126.571701806773,113.57987068343,76.4540968289114));
#20243=CARTESIAN_POINT('Ctrl Pts',(127.651676978702,112.354366949351,83.6326763250335));
#20244=CARTESIAN_POINT('Ctrl Pts',(132.966997982629,114.559964739603,71.3042501994499));
#20245=CARTESIAN_POINT('Ctrl Pts',(129.416365550538,110.330915246744,75.7039088018499));
#20246=CARTESIAN_POINT('Ctrl Pts',(130.449215516202,109.094078884113,82.5777372261749));
#20247=CARTESIAN_POINT('Ctrl Pts',(136.120374389438,109.984367133449,70.3373592580949));
#20248=CARTESIAN_POINT('Ctrl Pts',(132.838493553414,106.101344893951,74.6872762465277));
#20249=CARTESIAN_POINT('Ctrl Pts',(133.794311682361,104.88202612324,81.1964639412465));
#20250=CARTESIAN_POINT('Ctrl Pts',(136.743616942198,109.063325258521,70.1417843056297));
#20251=CARTESIAN_POINT('Ctrl Pts',(133.511839276197,105.252753785792,74.4814177447014));
#20252=CARTESIAN_POINT('Ctrl Pts',(134.455728161604,104.03277160558,80.9170710194299));
#20253=CARTESIAN_POINT('Ctrl Pts',(137.975229697851,107.209266309907,69.7462901240218));
#20254=CARTESIAN_POINT('Ctrl Pts',(134.843563811306,103.540882689278,74.0625229474022));
#20255=CARTESIAN_POINT('Ctrl Pts',(135.763304172514,102.320504511889,80.3520788936533));
#20256=CARTESIAN_POINT('Ctrl Pts',(138.584011129024,106.275579631437,69.5462255028335));
#20257=CARTESIAN_POINT('Ctrl Pts',(135.502515209047,102.676936655468,73.8493312382261));
#20258=CARTESIAN_POINT('Ctrl Pts',(136.409901038821,101.456869632069,80.0662719859412));
#20259=CARTESIAN_POINT('Ctrl Pts',(140.381410996897,103.46681038063,68.9418375941936));
#20260=CARTESIAN_POINT('Ctrl Pts',(137.44622664547,100.0771502473,73.2027293733177));
#20261=CARTESIAN_POINT('Ctrl Pts',(138.319688906568,98.8549121117867,79.202859577207));
#20262=CARTESIAN_POINT('Ctrl Pts',(141.543035442275,101.581203701731,68.5327283633642));
#20263=CARTESIAN_POINT('Ctrl Pts',(138.70739707142,98.3214899215068,72.7594318660626));
#20264=CARTESIAN_POINT('Ctrl Pts',(139.554945257313,97.1029464009744,78.6184167041338));
#20265=CARTESIAN_POINT('Ctrl Pts',(147.172811063143,92.087379772777,66.4580230839566));
#20266=CARTESIAN_POINT('Ctrl Pts',(144.769209540695,89.533625084567,70.5112314665258));
#20267=CARTESIAN_POINT('Ctrl Pts',(145.545768022766,88.2579658671962,75.6545459907609));
#20268=CARTESIAN_POINT('Ctrl Pts',(151.109449633708,84.2828338416036,64.7059125945462));
#20269=CARTESIAN_POINT('Ctrl Pts',(149.105656521244,82.1186746640789,68.5241447463077));
#20270=CARTESIAN_POINT('Ctrl Pts',(149.748394838999,80.9109007293675,73.1515201292455));
#20271=CARTESIAN_POINT('Ctrl Pts',(156.211187639656,72.2434629872912,61.9599182770527));
#20272=CARTESIAN_POINT('Ctrl Pts',(154.735913992316,70.5418248837457,65.3361267841599));
#20273=CARTESIAN_POINT('Ctrl Pts',(155.204094851699,69.494444703793,69.2286486643273));
#20274=CARTESIAN_POINT('Ctrl Pts',(157.777199757704,68.1747130608376,61.0247584570915));
#20275=CARTESIAN_POINT('Ctrl Pts',(156.462811523132,66.6261512273264,64.2443587388644));
#20276=CARTESIAN_POINT('Ctrl Pts',(156.880610977599,65.6227064854861,67.8926978274835));
#20277=CARTESIAN_POINT('Ctrl Pts',(159.924440854169,61.9838631433058,59.5934387075325));
#20278=CARTESIAN_POINT('Ctrl Pts',(158.835393854645,60.637084725701,62.5584808456691));
#20279=CARTESIAN_POINT('Ctrl Pts',(159.181124815158,59.7146207337651,65.8479415995783));
#20280=CARTESIAN_POINT('Ctrl Pts',(160.606519612154,59.9056105043635,59.1115603052182));
#20281=CARTESIAN_POINT('Ctrl Pts',(159.588605202354,58.6261359817312,61.9898219519289));
#20282=CARTESIAN_POINT('Ctrl Pts',(159.91221396583,57.7284955929032,65.1595391420191));
#20283=CARTESIAN_POINT('Ctrl Pts',(161.578790554131,56.7655952183065,58.381658570037));
#20284=CARTESIAN_POINT('Ctrl Pts',(160.663581107371,55.5804420707533,61.1251183623648));
#20285=CARTESIAN_POINT('Ctrl Pts',(160.954720457782,54.7238687144436,64.1168149427384));
#20286=CARTESIAN_POINT('Ctrl Pts',(161.894669322878,55.7142130958785,58.1369583834399));
#20287=CARTESIAN_POINT('Ctrl Pts',(161.012707510978,54.5605741948746,60.8350012341958));
#20288=CARTESIAN_POINT('Ctrl Pts',(161.293483687908,53.7171877677032,63.7672407289973));
#20289=CARTESIAN_POINT('Ctrl Pts',(162.507622034656,53.609926721994,57.6466368798811));
#20290=CARTESIAN_POINT('Ctrl Pts',(161.690355249542,52.5177903875452,60.2528453586207));
#20291=CARTESIAN_POINT('Ctrl Pts',(161.950956676584,51.7011776789588,63.0667763221949));
#20292=CARTESIAN_POINT('Ctrl Pts',(162.804784056278,52.5568039701366,57.4009654066192));
#20293=CARTESIAN_POINT('Ctrl Pts',(162.019036836798,51.4945755320385,59.9607244749972));
#20294=CARTESIAN_POINT('Ctrl Pts',(162.269760743604,50.6916407802224,62.7158144755576));
#20295=CARTESIAN_POINT('Ctrl Pts',(165.396228192944,43.0696062215838,55.1854558190958));
#20296=CARTESIAN_POINT('Ctrl Pts',(164.871359483185,42.3174710775594,57.3363962613807));
#20297=CARTESIAN_POINT('Ctrl Pts',(165.050384666089,41.5921040022264,59.5507777172448));
#20298=CARTESIAN_POINT('Ctrl Pts',(167.112953991422,34.5721559152113,53.1846925294639));
#20299=CARTESIAN_POINT('Ctrl Pts',(166.788260728433,33.9828141288519,54.9228163985495));
#20300=CARTESIAN_POINT('Ctrl Pts',(166.895487919238,33.4066584126088,56.6925206006809));
#20301=CARTESIAN_POINT('Ctrl Pts',(168.839541545282,21.7037023432943,50.1437575021141));
#20302=CARTESIAN_POINT('Ctrl Pts',(168.70884062626,21.342590484654,51.2420487378816));
#20303=CARTESIAN_POINT('Ctrl Pts',(168.751767516685,20.9849502863122,52.3482901787236));
#20304=CARTESIAN_POINT('Ctrl Pts',(169.272994226546,17.3937906477954,49.123418475587));
#20305=CARTESIAN_POINT('Ctrl Pts',(169.191375205164,17.10625282417,50.0050582261906));
#20306=CARTESIAN_POINT('Ctrl Pts',(169.217967102382,16.8203670207432,50.8906501976363));
#20307=CARTESIAN_POINT('Ctrl Pts',(169.708244737431,10.8943962228678,47.5833483445016));
#20308=CARTESIAN_POINT('Ctrl Pts',(169.675477965546,10.7154189680991,48.1364420790708));
#20309=CARTESIAN_POINT('Ctrl Pts',(169.686138855143,10.5368669288742,48.690530528023));
#20310=CARTESIAN_POINT('Ctrl Pts',(169.817467420501,8.72217091897812,47.0683956196518));
#20311=CARTESIAN_POINT('Ctrl Pts',(169.796983990652,8.5791113628161,47.5113888393872));
#20312=CARTESIAN_POINT('Ctrl Pts',(169.803634766948,8.43625666941946,47.9548772375799));
#20313=CARTESIAN_POINT('Ctrl Pts',(169.963400726732,4.36546597417207,46.0353525704263));
#20314=CARTESIAN_POINT('Ctrl Pts',(169.959277929682,4.29443906431818,46.2573336219265));
#20315=CARTESIAN_POINT('Ctrl Pts',(169.960625243948,4.22263819734908,46.4790883103916));
#20316=CARTESIAN_POINT('Ctrl Pts',(170.,2.17934967149295,45.5168739027144));
#20317=CARTESIAN_POINT('Ctrl Pts',(170.,2.14369814666887,45.6276358938455));
#20318=CARTESIAN_POINT('Ctrl Pts',(170.,2.10804680089195,45.7383979484285));
#20319=CARTESIAN_POINT('Ctrl Pts',(170.,0.,45.));
#20320=CARTESIAN_POINT('Ctrl Pts',(170.,0.,45.));
#20321=CARTESIAN_POINT('Ctrl Pts',(170.,0.,45.));
#20322=CARTESIAN_POINT('Origin',(65.4347826086958,173.041293409847,95.));
#20323=CARTESIAN_POINT('Origin',(0.,0.,95.));
#20324=CARTESIAN_POINT('Origin',(-14.5652173913043,184.425742352699,95.));
#20325=CARTESIAN_POINT('Ctrl Pts',(-13.3842538190363,169.472303783561,95.));
#20326=CARTESIAN_POINT('Ctrl Pts',(-13.3842538190363,169.472303783561,80.));
#20327=CARTESIAN_POINT('Ctrl Pts',(-14.5652173913043,184.425742352699,80.));
#20328=CARTESIAN_POINT('Ctrl Pts',(-17.5395512351767,169.144134790342,95.));
#20329=CARTESIAN_POINT('Ctrl Pts',(-17.2144232870799,169.169812112664,79.3644410713064));
#20330=CARTESIAN_POINT('Ctrl Pts',(-18.7318660089282,184.721037013812,80.));
#20331=CARTESIAN_POINT('Ctrl Pts',(-21.6441982168127,168.666370511884,94.8172074050833));
#20332=CARTESIAN_POINT('Ctrl Pts',(-20.8543660593525,168.752921516777,78.5305161733615));
#20333=CARTESIAN_POINT('Ctrl Pts',(-22.876822841872,184.876406726332,79.8720451835484));
#20334=CARTESIAN_POINT('Ctrl Pts',(-29.7513824612582,167.426614072389,94.060173223671));
#20335=CARTESIAN_POINT('Ctrl Pts',(-27.8670083443154,167.750643110992,76.4491424798736));
#20336=CARTESIAN_POINT('Ctrl Pts',(-31.1273096488505,184.919419561866,79.3421212565797));
#20337=CARTESIAN_POINT('Ctrl Pts',(-33.7540169272061,166.664538735009,93.4863288792126));
#20338=CARTESIAN_POINT('Ctrl Pts',(-31.2373560808963,167.15512258256,75.1777949173772));
#20339=CARTESIAN_POINT('Ctrl Pts',(-35.2329409933915,184.807006229873,78.9404302153998));
#20340=CARTESIAN_POINT('Ctrl Pts',(-39.6776586745835,165.317222135875,92.2879046923386));
#20341=CARTESIAN_POINT('Ctrl Pts',(-35.9693696574127,166.20324713768,72.9549331576006));
#20342=CARTESIAN_POINT('Ctrl Pts',(-41.3622144006103,184.443659034893,78.1015332846615));
#20343=CARTESIAN_POINT('Ctrl Pts',(-41.6387819418482,164.834067193048,91.8318643970813));
#20344=CARTESIAN_POINT('Ctrl Pts',(-37.5231338419952,165.868473328022,72.1406418324815));
#20345=CARTESIAN_POINT('Ctrl Pts',(-43.4004096859107,184.290063044221,77.7823050779236));
#20346=CARTESIAN_POINT('Ctrl Pts',(-44.5594044158236,164.059361041538,91.0538818796549));
#20347=CARTESIAN_POINT('Ctrl Pts',(-39.7599794861513,165.361699241537,70.8335077858203));
#20348=CARTESIAN_POINT('Ctrl Pts',(-46.4499795033957,184.011560356448,77.2377173157751));
#20349=CARTESIAN_POINT('Ctrl Pts',(-45.5294312692045,163.79279700543,90.7788716538768));
#20350=CARTESIAN_POINT('Ctrl Pts',(-40.4978371304263,165.190041788369,70.3778813312569));
#20351=CARTESIAN_POINT('Ctrl Pts',(-47.4652121610676,183.910707315012,77.0452101577021));
#20352=CARTESIAN_POINT('Ctrl Pts',(-47.4622527854103,163.243205136057,90.1955588967012));
#20353=CARTESIAN_POINT('Ctrl Pts',(-41.9450409744791,164.845993388777,69.4331574372367));
#20354=CARTESIAN_POINT('Ctrl Pts',(-49.4929835017655,183.693061788492,76.6368912277025));
#20355=CARTESIAN_POINT('Ctrl Pts',(-48.4266504515543,162.959685425406,89.8867032935461));
#20356=CARTESIAN_POINT('Ctrl Pts',(-42.6553053430736,164.673254829836,68.942551397809));
#20357=CARTESIAN_POINT('Ctrl Pts',(-50.5072136184811,183.576056117467,76.4206923054768));
#20358=CARTESIAN_POINT('Ctrl Pts',(-51.2966354956011,162.088412227551,88.9109268015102));
#20359=CARTESIAN_POINT('Ctrl Pts',(-44.7469464262981,164.155637506621,67.4128983527913));
#20360=CARTESIAN_POINT('Ctrl Pts',(-53.5329794899747,183.202867702932,75.7376487610681));
#20361=CARTESIAN_POINT('Ctrl Pts',(-53.1733448982289,161.481802427548,88.1971446848615));
#20362=CARTESIAN_POINT('Ctrl Pts',(-46.0494224580936,163.820664239566,66.3397922862081));
#20363=CARTESIAN_POINT('Ctrl Pts',(-55.5215816926986,182.925374134496,75.2380012793601));
#20364=CARTESIAN_POINT('Ctrl Pts',(-56.8511651327196,160.22397494123,86.6315720785634));
#20365=CARTESIAN_POINT('Ctrl Pts',(-48.478602658805,163.188342727077,64.082468778351));
#20366=CARTESIAN_POINT('Ctrl Pts',(-59.4384997234822,182.318483802645,74.1421004550374));
#20367=CARTESIAN_POINT('Ctrl Pts',(-58.6522951136164,159.572737982238,85.7798428475361));
#20368=CARTESIAN_POINT('Ctrl Pts',(-49.6000886182912,162.892055598081,62.8933190799086));
#20369=CARTESIAN_POINT('Ctrl Pts',(-61.3668401614234,181.989071709277,73.545889993238));
#20370=CARTESIAN_POINT('Ctrl Pts',(-62.1748189026221,158.23350569228,83.9219691980032));
#20371=CARTESIAN_POINT('Ctrl Pts',(-51.637017574247,162.366710734437,60.4121506921274));
#20372=CARTESIAN_POINT('Ctrl Pts',(-65.15798176608,181.284440720707,72.2453784386395));
#20373=CARTESIAN_POINT('Ctrl Pts',(-63.8962495517862,157.545478964947,82.9159377469876));
#20374=CARTESIAN_POINT('Ctrl Pts',(-52.545511584158,162.139981860392,59.1148834184348));
#20375=CARTESIAN_POINT('Ctrl Pts',(-67.0208288573461,180.909197594207,71.5411564228308));
#20376=CARTESIAN_POINT('Ctrl Pts',(-66.4135506755794,156.493026838041,81.2731565607321));
#20377=CARTESIAN_POINT('Ctrl Pts',(-53.7105373582531,161.881828084746,57.1273358583113));
#20378=CARTESIAN_POINT('Ctrl Pts',(-69.7596407351623,180.317443237727,70.3912095925427));
#20379=CARTESIAN_POINT('Ctrl Pts',(-67.2418202127918,156.138823420855,80.7032055873364));
#20380=CARTESIAN_POINT('Ctrl Pts',(-54.0699645553869,161.808931015126,56.4472226877468));
#20381=CARTESIAN_POINT('Ctrl Pts',(-70.6633063132461,180.115388269163,69.9922439111036));
#20382=CARTESIAN_POINT('Ctrl Pts',(-68.8754848173699,155.425101434584,79.514506063713));
#20383=CARTESIAN_POINT('Ctrl Pts',(-54.7189452269188,161.696107176842,55.0708260730923));
#20384=CARTESIAN_POINT('Ctrl Pts',(-72.4505873293311,179.702774329136,69.160154244631));
#20385=CARTESIAN_POINT('Ctrl Pts',(-69.6795919234263,155.066105739768,78.8965035406746));
#20386=CARTESIAN_POINT('Ctrl Pts',(-55.0063194658611,161.657075331116,54.3752022489627));
#20387=CARTESIAN_POINT('Ctrl Pts',(-73.3328070782591,179.492503237854,68.7275524784488));
#20388=CARTESIAN_POINT('Ctrl Pts',(-72.0324106623047,153.994488647569,76.9821802471142));
#20389=CARTESIAN_POINT('Ctrl Pts',(-55.7548099034461,161.598620210439,52.2723911996401));
#20390=CARTESIAN_POINT('Ctrl Pts',(-75.921231436318,178.857382701198,67.3875261730269));
#20391=CARTESIAN_POINT('Ctrl Pts',(-73.5292807993369,153.283865054872,75.62063975569));
#20392=CARTESIAN_POINT('Ctrl Pts',(-56.0781101307272,161.644219581938,50.8878411365529));
#20393=CARTESIAN_POINT('Ctrl Pts',(-77.5776030421959,178.426261084882,66.4344478289248));
#20394=CARTESIAN_POINT('Ctrl Pts',(-76.366751875532,151.890149874864,72.7006648710333));
#20395=CARTESIAN_POINT('Ctrl Pts',(-56.3756134497039,161.93051189576,48.2172467564738));
#20396=CARTESIAN_POINT('Ctrl Pts',(-80.7336339099764,177.564857597969,64.3904654097815));
#20397=CARTESIAN_POINT('Ctrl Pts',(-77.7075527077816,151.206919364782,71.1425408034194));
#20398=CARTESIAN_POINT('Ctrl Pts',(-56.3324815494095,162.180759006444,46.9371883104744));
#20399=CARTESIAN_POINT('Ctrl Pts',(-82.2335307362999,177.134474712401,63.2997785623094));
#20400=CARTESIAN_POINT('Ctrl Pts',(-79.5843975938565,150.222577239668,68.6265804660936));
#20401=CARTESIAN_POINT('Ctrl Pts',(-55.9936784211686,162.717602630982,45.2323932608695));
#20402=CARTESIAN_POINT('Ctrl Pts',(-84.3431679099447,176.505297510891,61.5386063263076));
#20403=CARTESIAN_POINT('Ctrl Pts',(-80.1887658265789,149.900578404234,67.755569241579));
#20404=CARTESIAN_POINT('Ctrl Pts',(-55.8294042116326,162.9288556975,44.6926349322782));
#20405=CARTESIAN_POINT('Ctrl Pts',(-85.0243102277581,176.297889106232,60.9288984690785));
#20406=CARTESIAN_POINT('Ctrl Pts',(-81.3314469036299,149.283680672992,65.9735353866643));
#20407=CARTESIAN_POINT('Ctrl Pts',(-55.4166431025694,163.399678588271,43.7235153888331));
#20408=CARTESIAN_POINT('Ctrl Pts',(-86.3151146859738,175.897970347453,59.6814747706918));
#20409=CARTESIAN_POINT('Ctrl Pts',(-81.871857983652,148.987704499459,65.0600083704848));
#20410=CARTESIAN_POINT('Ctrl Pts',(-55.1663164325277,163.660533878635,43.2952935416342));
#20411=CARTESIAN_POINT('Ctrl Pts',(-86.9271268382518,175.704778800986,59.0420058593072));
#20412=CARTESIAN_POINT('Ctrl Pts',(-82.8877983348762,148.424897200268,63.1847493041814));
#20413=CARTESIAN_POINT('Ctrl Pts',(-54.5968742872658,164.221510744674,42.5719496657066));
#20414=CARTESIAN_POINT('Ctrl Pts',(-88.0800512417677,175.335427624406,57.7293245129592));
#20415=CARTESIAN_POINT('Ctrl Pts',(-83.3633401165125,148.158058769467,62.2230271057914));
#20416=CARTESIAN_POINT('Ctrl Pts',(-54.276749072151,164.521983493455,42.2805814044158));
#20417=CARTESIAN_POINT('Ctrl Pts',(-88.6209776878574,175.159263160964,57.0561189740244));
#20418=CARTESIAN_POINT('Ctrl Pts',(-84.2452339637734,147.658380758111,60.2472126840058));
#20419=CARTESIAN_POINT('Ctrl Pts',(-53.5924579506749,165.144968110372,41.8573492354118));
#20420=CARTESIAN_POINT('Ctrl Pts',(-89.6259478489954,174.827893059694,55.6730488788336));
#20421=CARTESIAN_POINT('Ctrl Pts',(-84.6516057522163,147.425530224166,59.2331358058206));
#20422=CARTESIAN_POINT('Ctrl Pts',(-53.2282068700753,165.467180261645,41.7294386859836));
#20423=CARTESIAN_POINT('Ctrl Pts',(-90.0900138002506,174.672680323464,54.9631950640533));
#20424=CARTESIAN_POINT('Ctrl Pts',(-85.2047113619757,147.106092638268,57.668598294985));
#20425=CARTESIAN_POINT('Ctrl Pts',(-52.6783494190424,165.945140624608,41.6733190176321));
#20426=CARTESIAN_POINT('Ctrl Pts',(-90.7226032635016,174.458984880958,53.8680188065001));
#20427=CARTESIAN_POINT('Ctrl Pts',(-85.3800570143097,147.004359733543,57.1383954883763));
#20428=CARTESIAN_POINT('Ctrl Pts',(-52.4930107984057,166.104798004517,41.6778593074336));
#20429=CARTESIAN_POINT('Ctrl Pts',(-90.9233240871832,174.390787586828,53.4968768418598));
#20430=CARTESIAN_POINT('Ctrl Pts',(-85.7076058638931,146.813630884585,56.0739089930283));
#20431=CARTESIAN_POINT('Ctrl Pts',(-52.130067443758,166.415353901805,41.7330271353183));
#20432=CARTESIAN_POINT('Ctrl Pts',(-91.2985385599009,174.262722433064,52.7517362951234));
#20433=CARTESIAN_POINT('Ctrl Pts',(-85.8601535980719,146.72443849077,55.5388388898697));
#20434=CARTESIAN_POINT('Ctrl Pts',(-51.9524059049901,166.56629536905,41.7838517318022));
#20435=CARTESIAN_POINT('Ctrl Pts',(-91.473425281088,174.202723928459,52.3771872229046));
#20436=CARTESIAN_POINT('Ctrl Pts',(-86.2840014488134,146.475862855443,53.9250716815212));
#20437=CARTESIAN_POINT('Ctrl Pts',(-51.4370137885404,167.001978667705,42.0026128108074));
#20438=CARTESIAN_POINT('Ctrl Pts',(-91.9596328391763,174.03528173318,51.2475501770734));
#20439=CARTESIAN_POINT('Ctrl Pts',(-86.5215572476422,146.335470001124,52.8378286338531));
#20440=CARTESIAN_POINT('Ctrl Pts',(-51.1225180710597,167.264794255433,42.2370323177161));
#20441=CARTESIAN_POINT('Ctrl Pts',(-92.2325526199218,173.940389301699,50.4864800436924));
#20442=CARTESIAN_POINT('Ctrl Pts',(-86.9048658142535,146.108158385538,50.639890051958));
#20443=CARTESIAN_POINT('Ctrl Pts',(-50.5901985332046,167.707523804762,42.8482236974603));
#20444=CARTESIAN_POINT('Ctrl Pts',(-92.6732256277408,173.786512852862,48.9479230363755));
#20445=CARTESIAN_POINT('Ctrl Pts',(-87.050627720092,146.02123567785,49.5291966979117));
#20446=CARTESIAN_POINT('Ctrl Pts',(-50.3747927527441,167.885405901664,43.2250058043474));
#20447=CARTESIAN_POINT('Ctrl Pts',(-92.8409885630906,173.727526790654,48.1704376885321));
#20448=CARTESIAN_POINT('Ctrl Pts',(-87.2468358858299,145.904087274001,47.2833282524998));
#20449=CARTESIAN_POINT('Ctrl Pts',(-50.0788716488328,168.129413435683,44.066695404472));
#20450=CARTESIAN_POINT('Ctrl Pts',(-93.0668677799616,173.647986546177,46.598329776756));
#20451=CARTESIAN_POINT('Ctrl Pts',(-87.297297297057,145.873856069651,46.1481485313624));
#20452=CARTESIAN_POINT('Ctrl Pts',(-50.0000000004664,168.194190488835,44.5295600305827));
#20453=CARTESIAN_POINT('Ctrl Pts',(-93.1249999997334,173.62742978858,45.803703971949));
#20454=CARTESIAN_POINT('Ctrl Pts',(-87.2972972972973,145.873856069507,45.0000000000001));
#20455=CARTESIAN_POINT('Ctrl Pts',(-50.0000000000001,168.194190489106,45.));
#20456=CARTESIAN_POINT('Ctrl Pts',(-93.125,173.627429788614,45.0000000000001));
#20457=CARTESIAN_POINT('Ctrl Pts',(-87.2972972972973,145.873856069507,-45.));
#20458=CARTESIAN_POINT('Ctrl Pts',(-50.,168.194190489106,-45.));
#20459=CARTESIAN_POINT('Ctrl Pts',(-93.125,173.627429788614,-45.));
#20460=CARTESIAN_POINT('Ctrl Pts',(-87.2972972971987,145.873856069566,-46.1481557420891));
#20461=CARTESIAN_POINT('Ctrl Pts',(-50.0000000004424,168.194190488739,-44.5295601183673));
#20462=CARTESIAN_POINT('Ctrl Pts',(-93.1249999998352,173.627429788593,-45.8037090194605));
#20463=CARTESIAN_POINT('Ctrl Pts',(-87.2468342072022,145.90408834183,-47.2836204764629));
#20464=CARTESIAN_POINT('Ctrl Pts',(-50.07887561782,168.129410327578,-44.0665685622004));
#20465=CARTESIAN_POINT('Ctrl Pts',(-93.06686582199,173.647987290785,-46.5985343335265));
#20466=CARTESIAN_POINT('Ctrl Pts',(-87.0504855774481,146.021320480162,-49.5305505033));
#20467=CARTESIAN_POINT('Ctrl Pts',(-50.3750045511616,167.885231095311,-43.22451839411));
#20468=CARTESIAN_POINT('Ctrl Pts',(-92.8408249508251,173.727584349276,-48.1713853523075));
#20469=CARTESIAN_POINT('Ctrl Pts',(-86.9045853411086,146.108325679447,-50.6420203314529));
#20470=CARTESIAN_POINT('Ctrl Pts',(-50.5906119841123,167.70718247082,-42.8475063288785));
#20471=CARTESIAN_POINT('Ctrl Pts',(-92.6729028059307,173.7866263903,-48.9494142320252));
#20472=CARTESIAN_POINT('Ctrl Pts',(-86.5207468489932,146.335949618861,-52.8419520617065));
#20473=CARTESIAN_POINT('Ctrl Pts',(-51.1236121852308,167.263881768268,-42.236016926739));
#20474=CARTESIAN_POINT('Ctrl Pts',(-92.231621315453,173.940713684159,-50.4893664431864));
#20475=CARTESIAN_POINT('Ctrl Pts',(-86.2827997893804,146.476572189292,-53.930411905424));
#20476=CARTESIAN_POINT('Ctrl Pts',(-51.4385779165005,167.000669358337,-42.0015322603363));
#20477=CARTESIAN_POINT('Ctrl Pts',(-91.9582526161004,174.03576092614,-51.2512883338007));
#20478=CARTESIAN_POINT('Ctrl Pts',(-85.8580915626072,146.725645502692,-55.5463038168551));
#20479=CARTESIAN_POINT('Ctrl Pts',(-51.9548424687745,166.564229188848,-41.7830254980675));
#20480=CARTESIAN_POINT('Ctrl Pts',(-91.471060754875,174.203536282685,-52.3824126717966));
#20481=CARTESIAN_POINT('Ctrl Pts',(-85.7052114634742,146.815029246798,-56.0821321396214));
#20482=CARTESIAN_POINT('Ctrl Pts',(-52.1328160383236,166.413014140323,-41.7323431781605));
#20483=CARTESIAN_POINT('Ctrl Pts',(-91.295794141676,174.263662608782,-52.7574924977414));
#20484=CARTESIAN_POINT('Ctrl Pts',(-85.3768924607479,147.006198231513,-57.1482305947251));
#20485=CARTESIAN_POINT('Ctrl Pts',(-52.4964140404309,166.10187378431,-41.6776104852154));
#20486=CARTESIAN_POINT('Ctrl Pts',(-90.9197006272883,174.392020784196,-53.5037614163011));
#20487=CARTESIAN_POINT('Ctrl Pts',(-85.201572980522,147.107910335063,-57.6778553276653));
#20488=CARTESIAN_POINT('Ctrl Pts',(-52.6815987230577,165.942332214323,-41.6733918796236));
#20489=CARTESIAN_POINT('Ctrl Pts',(-90.7190119102538,174.460202437778,-53.8744987293807));
#20490=CARTESIAN_POINT('Ctrl Pts',(-84.6485098428038,147.427307739811,-59.2411239335854));
#20491=CARTESIAN_POINT('Ctrl Pts',(-53.2310695420675,165.46465987102,-41.730247968301));
#20492=CARTESIAN_POINT('Ctrl Pts',(-90.0864769882907,174.673866265291,-54.9687867534798));
#20493=CARTESIAN_POINT('Ctrl Pts',(-84.2419452441406,147.660259181751,-60.2551804226534));
#20494=CARTESIAN_POINT('Ctrl Pts',(-53.5952858098106,165.142447362445,-41.8585442148455));
#20495=CARTESIAN_POINT('Ctrl Pts',(-89.6221944884166,174.829143356289,-55.6786262958786));
#20496=CARTESIAN_POINT('Ctrl Pts',(-83.3589636976755,148.160523255651,-62.2322272830292));
#20497=CARTESIAN_POINT('Ctrl Pts',(-54.2798557221847,164.519102036724,-42.2830504688397));
#20498=CARTESIAN_POINT('Ctrl Pts',(-88.6159962195585,175.16089290001,-57.0625590980993));
#20499=CARTESIAN_POINT('Ctrl Pts',(-82.8825282275814,148.427846133224,-63.1952037501853));
#20500=CARTESIAN_POINT('Ctrl Pts',(-54.6002746634411,164.218288168885,-42.5752870988414));
#20501=CARTESIAN_POINT('Ctrl Pts',(-88.0740596024118,175.33737196623,-57.7366426251549));
#20502=CARTESIAN_POINT('Ctrl Pts',(-81.8638978961899,148.992084401777,-65.0739651883141));
#20503=CARTESIAN_POINT('Ctrl Pts',(-55.1703038853821,163.656479580582,-43.3013319230022));
#20504=CARTESIAN_POINT('Ctrl Pts',(-86.9181045359956,175.70764400461,-59.0517756317946));
#20505=CARTESIAN_POINT('Ctrl Pts',(-81.3216912305501,149.289006692322,-65.9897411795777));
#20506=CARTESIAN_POINT('Ctrl Pts',(-55.4209153337387,163.395146817933,-43.7313440943059));
#20507=CARTESIAN_POINT('Ctrl Pts',(-86.3040727099585,175.90144153157,-59.6928188257368));
#20508=CARTESIAN_POINT('Ctrl Pts',(-80.4611806720501,149.75347959498,-67.3302212152897));
#20509=CARTESIAN_POINT('Ctrl Pts',(-55.7323628889726,163.039374353445,-44.4659089553466));
#20510=CARTESIAN_POINT('Ctrl Pts',(-85.3320488395596,176.202519245937,-60.6311548506866));
#20511=CARTESIAN_POINT('Ctrl Pts',(-80.1660792196943,149.911692897809,-67.7720166440731));
#20512=CARTESIAN_POINT('Ctrl Pts',(-55.8249508600411,162.927551611724,-44.7233355746148));
#20513=CARTESIAN_POINT('Ctrl Pts',(-84.9990979101181,176.304741064775,-60.9404116508692));
#20514=CARTESIAN_POINT('Ctrl Pts',(-79.5649495321451,150.231603635495,-68.638474298271));
#20515=CARTESIAN_POINT('Ctrl Pts',(-55.9858061786668,162.71878843487,-45.2587322589989));
#20516=CARTESIAN_POINT('Ctrl Pts',(-84.3217302379204,176.510695829274,-61.5469320087717));
#20517=CARTESIAN_POINT('Ctrl Pts',(-79.2584561448351,150.393554949854,-69.0639054241725));
#20518=CARTESIAN_POINT('Ctrl Pts',(-56.0545272978165,162.621495302187,-45.5367648107279));
#20519=CARTESIAN_POINT('Ctrl Pts',(-83.9767870352385,176.614594219734,-61.8447337969382));
#20520=CARTESIAN_POINT('Ctrl Pts',(-77.6976281010343,151.211991727362,-71.1542377786429));
#20521=CARTESIAN_POINT('Ctrl Pts',(-56.3329566915923,162.17877220309,-46.946790015033));
#20522=CARTESIAN_POINT('Ctrl Pts',(-82.2224229503939,177.137674896828,-63.3079664449803));
#20523=CARTESIAN_POINT('Ctrl Pts',(-76.358755256544,151.894158252871,-72.7094834320272));
#20524=CARTESIAN_POINT('Ctrl Pts',(-56.3753525382564,161.929333704007,-48.2248892798433));
#20525=CARTESIAN_POINT('Ctrl Pts',(-80.7247115749601,177.567361482489,-64.3966384024778));
#20526=CARTESIAN_POINT('Ctrl Pts',(-73.5232682991988,153.286737307182,-75.6262347306282));
#20527=CARTESIAN_POINT('Ctrl Pts',(-56.0769147808614,161.64396004567,-50.8934787988654));
#20528=CARTESIAN_POINT('Ctrl Pts',(-77.5709436079268,178.428009730871,-66.438364311381));
#20529=CARTESIAN_POINT('Ctrl Pts',(-72.026462046429,153.997283676109,-76.9874494541838));
#20530=CARTESIAN_POINT('Ctrl Pts',(-55.7533758428049,161.598527556718,-52.277798604289));
#20531=CARTESIAN_POINT('Ctrl Pts',(-75.9146586641507,178.859068766111,-67.3912146179833));
#20532=CARTESIAN_POINT('Ctrl Pts',(-69.6720528505947,155.069496372499,-78.9024214954926));
#20533=CARTESIAN_POINT('Ctrl Pts',(-55.0037430741423,161.657376274586,-54.3817685485241));
#20534=CARTESIAN_POINT('Ctrl Pts',(-73.3245273944502,179.494497920776,-68.7316950468175));
#20535=CARTESIAN_POINT('Ctrl Pts',(-68.8668727613371,155.42891241544,-79.5209801538095));
#20536=CARTESIAN_POINT('Ctrl Pts',(-54.7157160376554,161.696600504129,-55.0782117530934));
#20537=CARTESIAN_POINT('Ctrl Pts',(-72.4411497039392,179.704994726958,-69.1646861076988));
#20538=CARTESIAN_POINT('Ctrl Pts',(-67.2348038674229,156.14183977231,-80.708101155254));
#20539=CARTESIAN_POINT('Ctrl Pts',(-54.066973497348,161.809518307269,-56.4530352471832));
#20540=CARTESIAN_POINT('Ctrl Pts',(-70.6556461223016,180.117114694266,-69.9956708086456));
#20541=CARTESIAN_POINT('Ctrl Pts',(-66.4074631994888,156.495603406397,-81.2772464428291));
#20542=CARTESIAN_POINT('Ctrl Pts',(-53.7077907544062,161.88241013336,-57.1322849215662));
#20543=CARTESIAN_POINT('Ctrl Pts',(-69.7530076022098,180.31890347519,-70.3940725100073));
#20544=CARTESIAN_POINT('Ctrl Pts',(-63.8933382808409,157.546632905389,-82.9176021366126));
#20545=CARTESIAN_POINT('Ctrl Pts',(-52.5438986519127,162.140391064739,-59.1171215542775));
#20546=CARTESIAN_POINT('Ctrl Pts',(-67.0176814730437,180.909823248112,-71.5423214955749));
#20547=CARTESIAN_POINT('Ctrl Pts',(-62.174543902428,158.233573752389,-83.9220069329356));
#20548=CARTESIAN_POINT('Ctrl Pts',(-51.6366986179836,162.366801122918,-60.4123360466614));
#20549=CARTESIAN_POINT('Ctrl Pts',(-65.157696820993,181.284462131077,-72.2454048531114));
#20550=CARTESIAN_POINT('Ctrl Pts',(-58.6583288600459,159.570480438189,-85.7767676195814));
#20551=CARTESIAN_POINT('Ctrl Pts',(-49.6036015941499,162.891141744692,-62.889235475676));
#20552=CARTESIAN_POINT('Ctrl Pts',(-61.3733230166759,181.987898288311,-73.5437373336506));
#20553=CARTESIAN_POINT('Ctrl Pts',(-56.8608714195449,160.220477504758,-86.6270094856871));
#20554=CARTESIAN_POINT('Ctrl Pts',(-48.4845845503338,163.186764146197,-64.0761818103832));
#20555=CARTESIAN_POINT('Ctrl Pts',(-59.4488880520778,182.316719637853,-74.1389066400079));
#20556=CARTESIAN_POINT('Ctrl Pts',(-53.1914516507995,161.475786363539,-88.1898645846761));
#20557=CARTESIAN_POINT('Ctrl Pts',(-46.061615193226,163.817511046626,-66.3291607861143));
#20558=CARTESIAN_POINT('Ctrl Pts',(-55.5408149349383,182.922547542729,-75.2329052092463));
#20559=CARTESIAN_POINT('Ctrl Pts',(-51.319470175582,162.081117268138,-88.902415984378));
#20560=CARTESIAN_POINT('Ctrl Pts',(-44.7628166978043,164.151587900672,-67.4001257057399));
#20561=CARTESIAN_POINT('Ctrl Pts',(-53.5571522154415,183.199569273526,-75.7316911890953));
#20562=CARTESIAN_POINT('Ctrl Pts',(-48.4573974379579,162.950528633808,-89.8766149078073));
#20563=CARTESIAN_POINT('Ctrl Pts',(-42.6777574357427,164.667756974113,-68.9266888034224));
#20564=CARTESIAN_POINT('Ctrl Pts',(-50.5395813143088,183.572219031567,-76.4136304354497));
#20565=CARTESIAN_POINT('Ctrl Pts',(-47.4925380968551,163.234409214934,-90.1860654079167));
#20566=CARTESIAN_POINT('Ctrl Pts',(-41.9675064328372,164.840576291436,-69.4179616869902));
#20567=CARTESIAN_POINT('Ctrl Pts',(-49.5248053055096,183.689484703437,-76.6302457855649));
#20568=CARTESIAN_POINT('Ctrl Pts',(-45.5559253860908,163.785442542513,-90.7712192710136));
#20569=CARTESIAN_POINT('Ctrl Pts',(-40.517921424902,165.185340070797,-70.3652778060076));
#20570=CARTESIAN_POINT('Ctrl Pts',(-47.4929604819986,183.907885928098,-77.0398534896864));
#20571=CARTESIAN_POINT('Ctrl Pts',(-44.5840993906858,164.052662821325,-91.0470382563051));
#20572=CARTESIAN_POINT('Ctrl Pts',(-39.7788834259429,165.357345411408,-70.8220737068328));
#20573=CARTESIAN_POINT('Ctrl Pts',(-46.4758027387637,184.009072193089,-77.2329267794284));
#20574=CARTESIAN_POINT('Ctrl Pts',(-41.6583648757858,164.829163150394,-91.8271696738661));
#20575=CARTESIAN_POINT('Ctrl Pts',(-37.5386431096872,165.865096098891,-72.1323233720483));
#20576=CARTESIAN_POINT('Ctrl Pts',(-43.4207826222858,184.288457643329,-77.7790187716767));
#20577=CARTESIAN_POINT('Ctrl Pts',(-39.6942137926577,165.31328171977,-92.2842750101778));
#20578=CARTESIAN_POINT('Ctrl Pts',(-35.9826718196518,166.200468258917,-72.9482919924133));
#20579=CARTESIAN_POINT('Ctrl Pts',(-41.3793866364986,184.44248647661,-78.0989925071645));
#20580=CARTESIAN_POINT('Ctrl Pts',(-33.7626089079634,166.662932669615,-93.4851484356314));
#20581=CARTESIAN_POINT('Ctrl Pts',(-31.2448533153792,167.153811440344,-75.175023213843));
#20582=CARTESIAN_POINT('Ctrl Pts',(-35.2417468235887,184.806791744904,-78.9396039048619));
#20583=CARTESIAN_POINT('Ctrl Pts',(-29.7561551119682,167.425823856563,-94.0596464150218));
#20584=CARTESIAN_POINT('Ctrl Pts',(-27.8711969032041,167.75000000849,-76.447793000883));
#20585=CARTESIAN_POINT('Ctrl Pts',(-31.1321796448434,184.919391068587,-79.341752490545));
#20586=CARTESIAN_POINT('Ctrl Pts',(-21.6443130141392,168.666413299276,-94.8172777838099));
#20587=CARTESIAN_POINT('Ctrl Pts',(-20.8545946334258,168.752931245308,-78.5305497139422));
#20588=CARTESIAN_POINT('Ctrl Pts',(-22.8769266922517,184.876461117654,-79.8720944486372));
#20589=CARTESIAN_POINT('Ctrl Pts',(-17.5388295044679,169.144191789785,-95.));
#20590=CARTESIAN_POINT('Ctrl Pts',(-17.2137406264089,169.169866026837,-79.3645543485074));
#20591=CARTESIAN_POINT('Ctrl Pts',(-18.7311428158619,184.720985760753,-80.));
#20592=CARTESIAN_POINT('Ctrl Pts',(-13.3842538190364,169.472303783561,-95.));
#20593=CARTESIAN_POINT('Ctrl Pts',(-13.3842538190364,169.472303783561,-80.));
#20594=CARTESIAN_POINT('Ctrl Pts',(-14.5652173913043,184.425742352699,-80.));
#20595=CARTESIAN_POINT('Origin',(-14.5652173913044,184.425742352699,-95.));
#20596=CARTESIAN_POINT('Origin',(0.,0.,-95.));
#20597=CARTESIAN_POINT('Origin',(65.4347826086956,173.041293409847,-95.));
#20598=CARTESIAN_POINT('Ctrl Pts',(60.1111342549551,159.017771142991,-94.9999991819279));
#20599=CARTESIAN_POINT('Ctrl Pts',(60.112229341533,159.017357178332,-79.9970998734751));
#20600=CARTESIAN_POINT('Ctrl Pts',(65.417178607917,173.051048440272,-79.9999995062288));
#20601=CARTESIAN_POINT('Ctrl Pts',(64.2759087790417,157.443422060874,-95.0003751304781));
#20602=CARTESIAN_POINT('Ctrl Pts',(63.9530157134296,157.565450775654,-80.5517566472176));
#20603=CARTESIAN_POINT('Ctrl Pts',(69.4980685405773,170.904779447422,-80.0002460391242));
#20604=CARTESIAN_POINT('Ctrl Pts',(68.3475790492405,155.717622096499,-94.871163811165));
#20605=CARTESIAN_POINT('Ctrl Pts',(67.839523093928,155.937210710705,-80.9562034651419));
#20606=CARTESIAN_POINT('Ctrl Pts',(73.4707419831936,168.632424521765,-79.9097827170611));
#20607=CARTESIAN_POINT('Ctrl Pts',(76.3074783717944,151.975267654439,-94.3981030531305));
#20608=CARTESIAN_POINT('Ctrl Pts',(75.4920654425922,152.377267494459,-81.4803630768627));
#20609=CARTESIAN_POINT('Ctrl Pts',(81.2094587552533,163.843390510905,-79.5786121633006));
#20610=CARTESIAN_POINT('Ctrl Pts',(80.1959679692073,149.959099180745,-94.0543379212976));
#20611=CARTESIAN_POINT('Ctrl Pts',(79.2729405895899,150.450643093642,-81.610159134502));
#20612=CARTESIAN_POINT('Ctrl Pts',(84.9757898620679,161.327031076194,-79.3379638009463));
#20613=CARTESIAN_POINT('Ctrl Pts',(87.8000684551132,145.637470058004,-93.1809712878189));
#20614=CARTESIAN_POINT('Ctrl Pts',(86.7038679660169,146.292589564658,-81.6312588884628));
#20615=CARTESIAN_POINT('Ctrl Pts',(92.3178905891635,156.046341746203,-78.7265842415997));
#20616=CARTESIAN_POINT('Ctrl Pts',(91.5156662167745,143.332003833586,-92.6512484049633));
#20617=CARTESIAN_POINT('Ctrl Pts',(90.3665685559524,144.064645405084,-81.5291708234098));
#20618=CARTESIAN_POINT('Ctrl Pts',(95.8936350663941,153.282013745197,-78.3557679793618));
#20619=CARTESIAN_POINT('Ctrl Pts',(96.9597420465583,139.655302598139,-91.7313856490923));
#20620=CARTESIAN_POINT('Ctrl Pts',(95.7862627909755,140.469122838069,-81.2184414032456));
#20621=CARTESIAN_POINT('Ctrl Pts',(101.118204141379,148.945321268586,-77.7118507119895));
#20622=CARTESIAN_POINT('Ctrl Pts',(98.7528522876294,138.393276733977,-91.4038190221124));
#20623=CARTESIAN_POINT('Ctrl Pts',(97.5656444562283,139.240074531893,-81.090445379421));
#20624=CARTESIAN_POINT('Ctrl Pts',(102.83651907572,147.468018852879,-77.482549883046));
#20625=CARTESIAN_POINT('Ctrl Pts',(102.295631429099,135.795539951176,-90.7084745843493));
#20626=CARTESIAN_POINT('Ctrl Pts',(101.08836342036,136.704210068963,-80.7859436045695));
#20627=CARTESIAN_POINT('Ctrl Pts',(106.226989111109,144.448761779836,-76.9958010076012));
#20628=CARTESIAN_POINT('Ctrl Pts',(104.036759724654,134.466015015237,-90.3423416599025));
#20629=CARTESIAN_POINT('Ctrl Pts',(102.824700624036,135.403548229412,-80.6106071343671));
#20630=CARTESIAN_POINT('Ctrl Pts',(107.890968825064,142.914010738197,-76.7395043944721));
#20631=CARTESIAN_POINT('Ctrl Pts',(109.159801879624,130.396180641668,-89.1948681948962));
#20632=CARTESIAN_POINT('Ctrl Pts',(107.914041417891,131.435704885724,-80.0241711884031));
#20633=CARTESIAN_POINT('Ctrl Pts',(112.780952607655,138.245372543666,-75.9362630669522));
#20634=CARTESIAN_POINT('Ctrl Pts',(112.446820922312,127.570888947651,-88.3636043219537));
#20635=CARTESIAN_POINT('Ctrl Pts',(111.217729898413,128.654798668491,-79.5479026354358));
#20636=CARTESIAN_POINT('Ctrl Pts',(115.910241206126,135.042722405181,-75.3543730932938));
#20637=CARTESIAN_POINT('Ctrl Pts',(118.773955285056,121.701958851828,-86.5841254176429));
#20638=CARTESIAN_POINT('Ctrl Pts',(117.585782049815,122.85919246317,-78.4483848675869));
#20639=CARTESIAN_POINT('Ctrl Pts',(121.921081617715,128.457279136201,-74.1087296370299));
#20640=CARTESIAN_POINT('Ctrl Pts',(121.814041889342,118.658306100528,-85.6358543716128));
#20641=CARTESIAN_POINT('Ctrl Pts',(120.66102035423,119.843166235463,-77.8267940587746));
#20642=CARTESIAN_POINT('Ctrl Pts',(124.802595789209,125.074482642951,-73.4449369322121));
#20643=CARTESIAN_POINT('Ctrl Pts',(127.651676978735,112.354366949315,-83.6326763250667));
#20644=CARTESIAN_POINT('Ctrl Pts',(126.571701813616,113.579870675594,-76.4540968745708));
#20645=CARTESIAN_POINT('Ctrl Pts',(130.325562248462,118.125822143933,-72.0427084706124));
#20646=CARTESIAN_POINT('Ctrl Pts',(130.449215516193,109.094078884125,-82.5777372262417));
#20647=CARTESIAN_POINT('Ctrl Pts',(129.416365557056,110.330915238904,-75.7039088453632));
#20648=CARTESIAN_POINT('Ctrl Pts',(132.966997945925,114.559964695876,-71.3042502449321));
#20649=CARTESIAN_POINT('Ctrl Pts',(133.794311682363,104.882026123237,-81.1964639412298));
#20650=CARTESIAN_POINT('Ctrl Pts',(132.838493559395,106.10134488633,-74.6872762872343));
#20651=CARTESIAN_POINT('Ctrl Pts',(136.120374355175,109.984367092914,-70.3373593035059));
#20652=CARTESIAN_POINT('Ctrl Pts',(134.455728161623,104.032771605557,-80.9170710194717));
#20653=CARTESIAN_POINT('Ctrl Pts',(133.511839282076,105.252753778121,-74.4814177849335));
#20654=CARTESIAN_POINT('Ctrl Pts',(136.743616908387,109.063325218641,-70.1417843510365));
#20655=CARTESIAN_POINT('Ctrl Pts',(135.763304172496,102.320504511913,-80.3520788936114));
#20656=CARTESIAN_POINT('Ctrl Pts',(134.843563817047,103.540882681733,-74.0625229865155));
#20657=CARTESIAN_POINT('Ctrl Pts',(137.975229665001,107.209266271442,-69.7462901692913));
#20658=CARTESIAN_POINT('Ctrl Pts',(136.409901038833,101.456869632053,-80.0662719859412));
#20659=CARTESIAN_POINT('Ctrl Pts',(135.502515214701,102.676936647862,-73.8493312768616));
#20660=CARTESIAN_POINT('Ctrl Pts',(138.58401109663,106.275579593581,-69.54622554808));
#20661=CARTESIAN_POINT('Ctrl Pts',(138.319688906544,98.8549121118194,-79.2028595772069));
#20662=CARTESIAN_POINT('Ctrl Pts',(137.446226650836,100.077150239795,-73.2027294103901));
#20663=CARTESIAN_POINT('Ctrl Pts',(140.38141096588,103.466810344861,-68.9418376391995));
#20664=CARTESIAN_POINT('Ctrl Pts',(139.554945257284,97.1029464010168,-78.6184167040672));
#20665=CARTESIAN_POINT('Ctrl Pts',(138.707397076576,98.3214899139818,-72.7594319021101));
#20666=CARTESIAN_POINT('Ctrl Pts',(141.543035412226,101.581203667191,-68.5327284081521));
#20667=CARTESIAN_POINT('Ctrl Pts',(145.545768022881,88.257965867027,-75.6545459910273));
#20668=CARTESIAN_POINT('Ctrl Pts',(144.769209545676,89.5336250768842,-70.5112314979136));
#20669=CARTESIAN_POINT('Ctrl Pts',(147.172811037201,92.0873797452005,-66.4580231276975));
#20670=CARTESIAN_POINT('Ctrl Pts',(149.748394839051,80.9109007292597,-73.1515201298415));
#20671=CARTESIAN_POINT('Ctrl Pts',(149.10565652523,82.1186746566399,-68.5241447747446));
#20672=CARTESIAN_POINT('Ctrl Pts',(151.109449611751,84.2828338177688,-64.7059126364692));
#20673=CARTESIAN_POINT('Ctrl Pts',(155.204094851673,69.494444703847,-69.2286486640292));
#20674=CARTESIAN_POINT('Ctrl Pts',(154.735913995021,70.5418248776468,-65.3361268068727));
#20675=CARTESIAN_POINT('Ctrl Pts',(156.211187623449,72.2434629686532,-61.9599183141271));
#20676=CARTESIAN_POINT('Ctrl Pts',(156.880610977566,65.6227064855729,-67.8926978273502));
#20677=CARTESIAN_POINT('Ctrl Pts',(156.462811525529,66.6261512215435,-64.244358760138));
#20678=CARTESIAN_POINT('Ctrl Pts',(157.777199743145,68.1747130437632,-61.0247584927152));
#20679=CARTESIAN_POINT('Ctrl Pts',(159.181124815175,59.7146207337219,-65.8479415996448));
#20680=CARTESIAN_POINT('Ctrl Pts',(158.835393856705,60.6370847202265,-62.5584808650695));
#20681=CARTESIAN_POINT('Ctrl Pts',(159.924440842033,61.9838631282589,-59.5934387405923));
#20682=CARTESIAN_POINT('Ctrl Pts',(159.912213965834,57.7284955928914,-65.1595391421529));
#20683=CARTESIAN_POINT('Ctrl Pts',(159.588605204181,58.6261359764456,-61.9898219706128));
#20684=CARTESIAN_POINT('Ctrl Pts',(160.606519600763,59.9056104900601,-59.1115603374229));
#20685=CARTESIAN_POINT('Ctrl Pts',(160.954720457779,54.7238687144498,-64.1168149426715));
#20686=CARTESIAN_POINT('Ctrl Pts',(160.663581109104,55.5804420657701,-61.1251183797621));
#20687=CARTESIAN_POINT('Ctrl Pts',(161.578790543905,56.765595205057,-58.381658600695));
#20688=CARTESIAN_POINT('Ctrl Pts',(161.29348368791,53.7171877676969,-63.7672407290392));
#20689=CARTESIAN_POINT('Ctrl Pts',(161.012707512599,54.5605741899303,-60.8350012513618));
#20690=CARTESIAN_POINT('Ctrl Pts',(161.894669312994,55.7142130829498,-58.1369584136762));
#20691=CARTESIAN_POINT('Ctrl Pts',(161.950956676582,51.7011776789652,-63.0667763221531));
#20692=CARTESIAN_POINT('Ctrl Pts',(161.690355251076,52.5177903828148,-60.2528453749454));
#20693=CARTESIAN_POINT('Ctrl Pts',(162.507622025497,53.6099267097544,-57.6466369090903));
#20694=CARTESIAN_POINT('Ctrl Pts',(162.269760743618,50.6916407801757,-62.7158144756995));
#20695=CARTESIAN_POINT('Ctrl Pts',(162.019036838256,51.4945755273328,-59.9607244911299));
#20696=CARTESIAN_POINT('Ctrl Pts',(162.804784047433,52.5568039581638,-57.4009654354441));
#20697=CARTESIAN_POINT('Ctrl Pts',(165.050384665975,41.5921040025995,-59.5507777161095));
#20698=CARTESIAN_POINT('Ctrl Pts',(164.871359484215,42.3174710736492,-57.3363962733902));
#20699=CARTESIAN_POINT('Ctrl Pts',(165.396228187219,43.0696062134821,-55.1854558426586));
#20700=CARTESIAN_POINT('Ctrl Pts',(166.895487919146,33.4066584132222,-56.6925205986574));
#20701=CARTESIAN_POINT('Ctrl Pts',(166.788260729585,33.9828141264701,-54.9228164063036));
#20702=CARTESIAN_POINT('Ctrl Pts',(167.112953987927,34.5721559092001,-53.184692547786));
#20703=CARTESIAN_POINT('Ctrl Pts',(168.751767516731,20.9849502860056,-52.3482901797354));
#20704=CARTESIAN_POINT('Ctrl Pts',(168.708840626242,21.3425904821289,-51.2420487454299));
#20705=CARTESIAN_POINT('Ctrl Pts',(168.839541543698,21.7037023388406,-50.1437575153319));
#20706=CARTESIAN_POINT('Ctrl Pts',(169.217967102393,16.8203670205984,-50.8906501981523));
#20707=CARTESIAN_POINT('Ctrl Pts',(169.191375205316,17.1062528224251,-50.0050582315602));
#20708=CARTESIAN_POINT('Ctrl Pts',(169.272994225589,17.3937906443598,-49.1234184860096));
#20709=CARTESIAN_POINT('Ctrl Pts',(169.686138855138,10.5368669289468,-48.6905305277644));
#20710=CARTESIAN_POINT('Ctrl Pts',(169.675477965606,10.7154189671323,-48.1364420820892));
#20711=CARTESIAN_POINT('Ctrl Pts',(169.70824473707,10.8943962209014,-47.5833483506363));
#20712=CARTESIAN_POINT('Ctrl Pts',(169.803634766947,8.43625666946546,-47.9548772374033));
#20713=CARTESIAN_POINT('Ctrl Pts',(169.796983992598,8.57911136209104,-47.5113888418552));
#20714=CARTESIAN_POINT('Ctrl Pts',(169.817467420272,8.72217091739304,-47.0683956245868));
#20715=CARTESIAN_POINT('Ctrl Pts',(169.96062524395,4.22263819730324,-46.4790883105662));
#20716=CARTESIAN_POINT('Ctrl Pts',(169.959277927784,4.29443906381557,-46.2573336232601));
#20717=CARTESIAN_POINT('Ctrl Pts',(169.96340072668,4.36546597331119,-46.0353525730877));
#20718=CARTESIAN_POINT('Ctrl Pts',(170.,2.10804680144307,-45.7383979468224));
#20719=CARTESIAN_POINT('Ctrl Pts',(170.,2.1436981469272,-45.6276358930879));
#20720=CARTESIAN_POINT('Ctrl Pts',(170.,2.17934967138514,-45.516873902782));
#20721=CARTESIAN_POINT('Ctrl Pts',(170.,0.,-45.));
#20722=CARTESIAN_POINT('Ctrl Pts',(170.,0.,-45.));
#20723=CARTESIAN_POINT('Ctrl Pts',(170.,0.,-45.));
#20724=CARTESIAN_POINT('Origin',(0.,0.,-95.));
#20725=CARTESIAN_POINT('Origin',(0.,0.,-95.));
#20726=CARTESIAN_POINT('Origin',(-115.,0.,-105.));
#20727=CARTESIAN_POINT('',(-95.6492560750855,183.985186114405,-44.9999999999999));
#20728=CARTESIAN_POINT('Origin',(-115.,0.,-44.9999999999999));
#20729=CARTESIAN_POINT('',(-95.6492560750855,183.985186114405,45.0000000000001));
#20730=CARTESIAN_POINT('',(-95.6492560750855,183.985186114405,-105.));
#20731=CARTESIAN_POINT('Origin',(-115.,0.,45.0000000000001));
#20732=CARTESIAN_POINT('Origin',(-115.000000000001,175.,70.0000000000001));
#20733=CARTESIAN_POINT('',(-93.0342906798268,208.848049102839,70.0000000000001));
#20734=CARTESIAN_POINT('',(-14.5652173913043,184.425742352699,70.));
#20735=CARTESIAN_POINT('Origin',(-115.,0.,70.0000000000001));
#20736=CARTESIAN_POINT('',(-108.033967922038,209.585728186396,70.));
#20737=CARTESIAN_POINT('Origin',(-107.155103814224,74.5885889652995,70.0000000000001));
#20738=CARTESIAN_POINT('',(-108.033967922038,249.902929948988,70.0000000000001));
#20739=CARTESIAN_POINT('',(-108.033967922038,175.,70.0000000000001));
#20740=CARTESIAN_POINT('',(65.4347826086958,173.041293409847,70.));
#20741=CARTESIAN_POINT('Origin',(-115.,0.,70.0000000000001));
#20742=CARTESIAN_POINT('Origin',(-6.30808536718839E-15,0.,70.));
#20743=CARTESIAN_POINT('Origin',(-115.,0.,-105.));
#20744=CARTESIAN_POINT('',(-107.337364714242,274.893222943887,45.0000000000001));
#20745=CARTESIAN_POINT('Origin',(-115.,0.,45.0000000000001));
#20746=CARTESIAN_POINT('',(-115.000000000001,275.,45.1798442476467));
#20747=CARTESIAN_POINT('Origin',(-109.334804813311,203.273336013208,165.779888116268));
#20748=CARTESIAN_POINT('',(-115.000000000001,275.,-45.1798442476466));
#20749=CARTESIAN_POINT('',(-115.000000000001,275.,2.35800814060629E-28));
#20750=CARTESIAN_POINT('',(-107.337364714242,274.893222943887,-44.9999999999999));
#20751=CARTESIAN_POINT('Origin',(-109.334804813308,203.273336012913,-165.779888116317));
#20752=CARTESIAN_POINT('Origin',(-115.,0.,-44.9999999999999));
#20753=CARTESIAN_POINT('Origin',(-115.000000000001,175.,-70.));
#20754=CARTESIAN_POINT('',(-108.033967922038,249.902929948988,-69.9999999999999));
#20755=CARTESIAN_POINT('',(65.4347826086956,173.041293409847,-70.));
#20756=CARTESIAN_POINT('Origin',(-115.,0.,-70.));
#20757=CARTESIAN_POINT('',(-108.033967922038,209.585728186396,-70.));
#20758=CARTESIAN_POINT('',(-108.033967922038,175.,-70.));
#20759=CARTESIAN_POINT('',(-93.0342906798268,208.848049102839,-70.));
#20760=CARTESIAN_POINT('Origin',(-107.155103814224,74.5885889652995,-70.));
#20761=CARTESIAN_POINT('',(-14.5652173913044,184.425742352699,-70.));
#20762=CARTESIAN_POINT('Origin',(-115.,0.,-70.));
#20763=CARTESIAN_POINT('Origin',(6.30808536718839E-15,0.,-70.));
#20764=CARTESIAN_POINT('Origin',(-9.76996261670139E-13,275.,2.35800814060629E-28));
#20765=CARTESIAN_POINT('',(-126.751426934183,275.,46.3038641989654));
#20766=CARTESIAN_POINT('Origin',(-108.033967922038,275.,180.));
#20767=CARTESIAN_POINT('',(3.92135447228736,275.,28.0096748020595));
#20768=CARTESIAN_POINT('',(-126.751426934183,275.,-46.3038641989653));
#20769=CARTESIAN_POINT('',(3.92135447228734,275.,-28.0096748020595));
#20770=CARTESIAN_POINT('Origin',(-108.033967922039,275.,-180.));
#20771=CARTESIAN_POINT('Origin',(7.3875505856485,2.56307148617813E-14,52.7682184689178));
#20772=CARTESIAN_POINT('',(-130.164585944519,206.966980183574,72.0255175831412));
#20773=CARTESIAN_POINT('',(-36.8701707223189,225.625863228014,58.9642994520331));
#20774=CARTESIAN_POINT('',(-123.285230820823,250.,71.0624078658237));
#20775=CARTESIAN_POINT('',(7.38755058564849,250.,52.7682184689177));
#20776=CARTESIAN_POINT('',(-123.285230820823,208.15873578029,71.0624078658237));
#20777=CARTESIAN_POINT('',(-123.285230820823,2.56307148617813E-14,71.0624078658238));
#20778=CARTESIAN_POINT('Origin',(-103.70046162358,72.0502949994303,68.3205401782068));
#20779=CARTESIAN_POINT('Origin',(7.38755058564847,2.56307148617812E-14,
-52.7682184689177));
#20780=CARTESIAN_POINT('',(-123.285230820823,250.,-71.0624078658236));
#20781=CARTESIAN_POINT('',(-123.285230820823,208.15873578029,-71.0624078658236));
#20782=CARTESIAN_POINT('',(-123.285230820823,2.56307148617812E-14,-71.0624078658237));
#20783=CARTESIAN_POINT('',(7.38755058564846,249.999999999999,-52.7682184689176));
#20784=CARTESIAN_POINT('',(-130.164585944519,206.966980183574,-72.0255175831411));
#20785=CARTESIAN_POINT('',(-36.870170722319,225.625863228014,-58.964299452033));
#20786=CARTESIAN_POINT('Origin',(-103.700461599128,72.0502948555587,-68.3205401747857));
#20787=CARTESIAN_POINT('Origin',(-40.0380844283057,200.190422141525,9.66330504221541E-15));
#20788=CARTESIAN_POINT('',(-128.727878679424,182.452463291301,47.2669739162829));
#20789=CARTESIAN_POINT('',(-35.4334634572244,201.111346335741,34.2057557851749));
#20790=CARTESIAN_POINT('',(-128.727878679425,182.452463291301,-47.2669739162828));
#20791=CARTESIAN_POINT('',(-128.727878679425,182.452463291301,9.66330504221541E-15));
#20792=CARTESIAN_POINT('',(-35.4334634572244,201.111346335741,-34.2057557851748));
#20793=CARTESIAN_POINT('Origin',(-108.033967922037,-3.74818120714568E-13,
180.));
#20794=CARTESIAN_POINT('',(-113.709994059638,250.,70.1465397573418));
#20795=CARTESIAN_POINT('Origin',(-108.033967922038,250.,180.));
#20796=CARTESIAN_POINT('Origin',(-109.765188581363,199.310273833714,146.488884695692));
#20797=CARTESIAN_POINT('Ctrl Pts',(-123.285230820823,208.15873578029,71.0624078658237));
#20798=CARTESIAN_POINT('Ctrl Pts',(-120.772211061873,208.611218684362,70.7105850995707));
#20799=CARTESIAN_POINT('Ctrl Pts',(-118.243257051618,208.957585927806,70.4450832185436));
#20800=CARTESIAN_POINT('Ctrl Pts',(-115.698109518352,209.19624749802,70.267320575903));
#20801=CARTESIAN_POINT('Ctrl Pts',(-113.490059874391,209.40329899042,70.1131021132552));
#20802=CARTESIAN_POINT('Ctrl Pts',(-111.269812456632,209.529293532016,70.0249139423489));
#20803=CARTESIAN_POINT('Ctrl Pts',(-109.037063883093,209.572105119168,70.0045693065261));
#20804=CARTESIAN_POINT('Ctrl Pts',(-108.702978801238,209.578510996107,70.0015251485744));
#20805=CARTESIAN_POINT('Ctrl Pts',(-108.368613822657,209.583054418182,70.));
#20806=CARTESIAN_POINT('Ctrl Pts',(-108.033967922038,209.585728186396,70.));
#20807=CARTESIAN_POINT('Origin',(-107.155103814224,74.5885889652995,-105.));
#20808=CARTESIAN_POINT('',(-123.122478208265,183.423523407144,-46.3038641989653));
#20809=CARTESIAN_POINT('',(-107.87121530948,184.586257960267,-44.9999999999999));
#20810=CARTESIAN_POINT('Ctrl Pts',(-123.122478208265,183.423523407144,-46.3038641989653));
#20811=CARTESIAN_POINT('Ctrl Pts',(-120.609173163533,183.792255035655,-45.8720326960086));
#20812=CARTESIAN_POINT('Ctrl Pts',(-118.08021495677,184.07446046044,-45.5462136818661));
#20813=CARTESIAN_POINT('Ctrl Pts',(-115.535356905798,184.268903325358,-45.3280752522695));
#20814=CARTESIAN_POINT('Ctrl Pts',(-113.288417354346,184.440583377813,-45.1354736001008));
#20815=CARTESIAN_POINT('Ctrl Pts',(-111.029072640325,184.543852620633,-45.0268083769033));
#20816=CARTESIAN_POINT('Ctrl Pts',(-108.75701249268,184.576927773769,-45.004372785009));
#20817=CARTESIAN_POINT('Ctrl Pts',(-108.461961429881,184.581222932546,-45.0014592858925));
#20818=CARTESIAN_POINT('Ctrl Pts',(-108.166695930546,184.584334309781,-45.));
#20819=CARTESIAN_POINT('Ctrl Pts',(-107.87121530948,184.586257960267,-45.));
#20820=CARTESIAN_POINT('Origin',(-107.170701202847,71.4826465588299,-43.5630588770692));
#20821=CARTESIAN_POINT('',(-123.122478208265,183.423523407144,46.3038641989655));
#20822=CARTESIAN_POINT('Origin',(-107.170701202831,71.4826465587667,43.5630588771165));
#20823=CARTESIAN_POINT('',(-107.87121530948,184.586257960267,45.0000000000001));
#20824=CARTESIAN_POINT('Ctrl Pts',(-107.87121530948,184.586257960267,45.0000000000001));
#20825=CARTESIAN_POINT('Ctrl Pts',(-110.146583407099,184.571444762264,45.0000000000001));
#20826=CARTESIAN_POINT('Ctrl Pts',(-112.409195439908,184.486203531093,45.0865304305993));
#20827=CARTESIAN_POINT('Ctrl Pts',(-114.65936227692,184.332321719849,45.2572927923187));
#20828=CARTESIAN_POINT('Ctrl Pts',(-114.951570140632,184.312338545895,45.2794680835459));
#20829=CARTESIAN_POINT('Ctrl Pts',(-115.24356812522,184.291197789453,45.3030638979795));
#20830=CARTESIAN_POINT('Ctrl Pts',(-115.535356905797,184.268903325358,45.3280752522795));
#20831=CARTESIAN_POINT('Ctrl Pts',(-118.080214956822,184.074460460436,45.5462136818366));
#20832=CARTESIAN_POINT('Ctrl Pts',(-120.60917316356,183.792255035651,45.8720326958299));
#20833=CARTESIAN_POINT('Ctrl Pts',(-123.122478208265,183.423523407144,46.3038641989655));
#20834=CARTESIAN_POINT('Origin',(-107.155103814224,74.5885889652995,45.0000000000001));
#20835=CARTESIAN_POINT('Origin',(-107.155103814224,74.5885889652995,-44.9999999999999));
#20836=CARTESIAN_POINT('Origin',(-108.033967922038,-3.74818120714567E-13,
-180.));
#20837=CARTESIAN_POINT('',(-113.709994059637,250.,-70.1465397573417));
#20838=CARTESIAN_POINT('Origin',(-109.765188581367,199.3102738337,-146.488884695695));
#20839=CARTESIAN_POINT('Origin',(-108.033967922038,250.,-180.));
#20840=CARTESIAN_POINT('Ctrl Pts',(-108.033967922038,209.585728186396,-69.9999999999999));
#20841=CARTESIAN_POINT('Ctrl Pts',(-110.270464428139,209.567858930397,-69.9999999999999));
#20842=CARTESIAN_POINT('Ctrl Pts',(-112.494413985885,209.46648519935,-70.068117723223));
#20843=CARTESIAN_POINT('Ctrl Pts',(-114.706120670835,209.28373893618,-70.2025349187483));
#20844=CARTESIAN_POINT('Ctrl Pts',(-115.037057397657,209.256394690859,-70.2226477063157));
#20845=CARTESIAN_POINT('Ctrl Pts',(-115.367720010236,209.227228522798,-70.2442449343946));
#20846=CARTESIAN_POINT('Ctrl Pts',(-115.698109518352,209.19624749802,-70.2673205759029));
#20847=CARTESIAN_POINT('Ctrl Pts',(-118.243257051566,208.957585927807,-70.4450832185398));
#20848=CARTESIAN_POINT('Ctrl Pts',(-120.772211061871,208.611218684354,-70.7105850995704));
#20849=CARTESIAN_POINT('Ctrl Pts',(-123.285230820823,208.15873578029,-71.0624078658236));
#20850=CARTESIAN_POINT('Origin',(-40.3363668356791,225.625863228014,-34.2057557851748));
#20851=CARTESIAN_POINT('Origin',(-133.630782057879,206.966980183574,-47.2669739162828));
#20852=CARTESIAN_POINT('Ctrl Pts',(-123.122478208265,183.423523407144,-46.3038641989654));
#20853=CARTESIAN_POINT('Ctrl Pts',(-119.79626063639,183.911518935037,-70.573952040003));
#20854=CARTESIAN_POINT('Ctrl Pts',(-123.285230820823,208.15873578029,-71.0624078658236));
#20855=CARTESIAN_POINT('Ctrl Pts',(-124.998899886253,183.148230114533,-46.6262675599709));
#20856=CARTESIAN_POINT('Ctrl Pts',(-121.695019586639,183.691462295903,-70.8397782931125));
#20857=CARTESIAN_POINT('Ctrl Pts',(-125.588111971152,207.820875830254,-71.3848112268697));
#20858=CARTESIAN_POINT('Ctrl Pts',(-126.86819905826,182.824399215534,-46.9474471449936));
#20859=CARTESIAN_POINT('Ctrl Pts',(-123.591604529994,183.421472951449,-71.1053001850761));
#20860=CARTESIAN_POINT('Ctrl Pts',(-127.882251854971,207.423447001444,-71.7059908106043));
#20861=CARTESIAN_POINT('Ctrl Pts',(-128.727878679424,182.452463291301,-47.2669739162828));
#20862=CARTESIAN_POINT('Ctrl Pts',(-125.483223478439,183.101394331498,-71.3701268378898));
#20863=CARTESIAN_POINT('Ctrl Pts',(-130.164585944519,206.966980183574,-72.0255175831411));
#20864=CARTESIAN_POINT('Origin',(-126.751426934183,208.15873578029,-46.3038641989653));
#20865=CARTESIAN_POINT('Ctrl Pts',(-107.87121530948,184.586257960267,-44.9999999999999));
#20866=CARTESIAN_POINT('Ctrl Pts',(-107.87121530948,184.586257960267,-69.9999999999999));
#20867=CARTESIAN_POINT('Ctrl Pts',(-108.033967922038,209.585728186396,-69.9999999999999));
#20868=CARTESIAN_POINT('Ctrl Pts',(-110.438920857601,184.569541574581,-44.9999999999671));
#20869=CARTESIAN_POINT('Ctrl Pts',(-109.855167975854,184.573341947487,-69.9962013003749));
#20870=CARTESIAN_POINT('Ctrl Pts',(-110.601673611506,209.565212621119,-69.9999999999999));
#20871=CARTESIAN_POINT('Ctrl Pts',(-112.993544026661,184.463113520349,-45.1101978466298));
#20872=CARTESIAN_POINT('Ctrl Pts',(-111.8270421663,184.512020248025,-70.0409090864542));
#20873=CARTESIAN_POINT('Ctrl Pts',(-113.156296639219,209.434596373781,-70.0897908380047));
#20874=CARTESIAN_POINT('Ctrl Pts',(-118.077169784938,184.074693130366,-45.5459526578601));
#20875=CARTESIAN_POINT('Ctrl Pts',(-115.791831475917,184.289393680222,-70.2300552343412));
#20876=CARTESIAN_POINT('Ctrl Pts',(-118.239922397497,208.957898622415,-70.4448503138019));
#20877=CARTESIAN_POINT('Ctrl Pts',(-120.606185416306,183.792693373573,-45.8715193467126));
#20878=CARTESIAN_POINT('Ctrl Pts',(-117.778521014566,184.128732905586,-70.3739036491836));
#20879=CARTESIAN_POINT('Ctrl Pts',(-120.768938161273,208.611807987944,-70.7101268934865));
#20880=CARTESIAN_POINT('Ctrl Pts',(-123.122478208265,183.423523407144,-46.3038641989653));
#20881=CARTESIAN_POINT('Ctrl Pts',(-119.79626063639,183.911518935037,-70.573952040003));
#20882=CARTESIAN_POINT('Ctrl Pts',(-123.285230820823,208.15873578029,-71.0624078658236));
#20883=CARTESIAN_POINT('Origin',(-108.033967922038,209.585728186396,-44.9999999999999));
#20884=CARTESIAN_POINT('Origin',(-107.155103814224,74.5885889652995,-44.9999999999999));
#20885=CARTESIAN_POINT('Origin',(-93.0342906798268,208.848049102839,-45.));
#20886=CARTESIAN_POINT('Origin',(-115.,0.,-44.9999999999999));
#20887=CARTESIAN_POINT('Ctrl Pts',(-14.5652173913044,184.425742352699,-70.));
#20888=CARTESIAN_POINT('Ctrl Pts',(-16.3332090306658,184.754274466599,-70.));
#20889=CARTESIAN_POINT('Ctrl Pts',(-18.1023329015486,185.057744804456,-69.9814986316322));
#20890=CARTESIAN_POINT('Ctrl Pts',(-19.872512033359,185.336453963332,-69.9438574986233));
#20891=CARTESIAN_POINT('Ctrl Pts',(-21.6426911651695,185.615163122208,-69.9062163656144));
#20892=CARTESIAN_POINT('Ctrl Pts',(-23.413925616323,185.869111277598,-69.8494352575069));
#20893=CARTESIAN_POINT('Ctrl Pts',(-25.1861398363754,186.098646846334,-69.7729130408332));
#20894=CARTESIAN_POINT('Ctrl Pts',(-25.5781521525593,186.149419923837,-69.7559863899473));
#20895=CARTESIAN_POINT('Ctrl Pts',(-25.9702115289155,186.198996530262,-69.7380937641867));
#20896=CARTESIAN_POINT('Ctrl Pts',(-26.3623178779184,186.247381007943,-69.7192288310756));
#20897=CARTESIAN_POINT('Ctrl Pts',(-28.0897549408391,186.460540372048,-69.6361187648179));
#20898=CARTESIAN_POINT('Ctrl Pts',(-29.8181218381042,186.650553146811,-69.5341740687916));
#20899=CARTESIAN_POINT('Ctrl Pts',(-31.547298538853,186.817623039099,-69.4121562675502));
#20900=CARTESIAN_POINT('Ctrl Pts',(-32.9744695816452,186.955513696713,-69.3114492243883));
#20901=CARTESIAN_POINT('Ctrl Pts',(-34.4021922929087,187.077776406133,-69.1970689821003));
#20902=CARTESIAN_POINT('Ctrl Pts',(-35.8304007809344,187.184542684468,-69.068339898143));
#20903=CARTESIAN_POINT('Ctrl Pts',(-36.6176289651215,187.243392232087,-68.9973844572074));
#20904=CARTESIAN_POINT('Ctrl Pts',(-37.4050006589494,187.297524969372,-68.922068073687));
#20905=CARTESIAN_POINT('Ctrl Pts',(-38.1925161207239,187.346963461637,-68.8422776054607));
#20906=CARTESIAN_POINT('Ctrl Pts',(-40.0459152858722,187.463315793415,-68.6544926102758));
#20907=CARTESIAN_POINT('Ctrl Pts',(-41.9000878550032,187.553637649455,-68.4417940850099));
#20908=CARTESIAN_POINT('Ctrl Pts',(-43.7548464440809,187.618108571057,-68.2017594754763));
#20909=CARTESIAN_POINT('Ctrl Pts',(-43.8781086657332,187.62239313352,-68.1858074268276));
#20910=CARTESIAN_POINT('Ctrl Pts',(-44.0013734754008,187.62656353256,-68.1697346633771));
#20911=CARTESIAN_POINT('Ctrl Pts',(-44.1246408180115,187.630619824725,-68.1535404814305));
#20912=CARTESIAN_POINT('Ctrl Pts',(-44.9138902588186,187.656591231711,-68.0498532535323));
#20913=CARTESIAN_POINT('Ctrl Pts',(-45.7032416288397,187.677883839451,-67.9411788907505));
#20914=CARTESIAN_POINT('Ctrl Pts',(-46.492669161194,187.694509338513,-67.8272800457684));
#20915=CARTESIAN_POINT('Ctrl Pts',(-46.6935155796415,187.69873920358,-67.7983018632978));
#20916=CARTESIAN_POINT('Ctrl Pts',(-46.8943739810412,187.702667120824,-67.7689845079355));
#20917=CARTESIAN_POINT('Ctrl Pts',(-47.0952639568852,187.706293513407,-67.7393209875906));
#20918=CARTESIAN_POINT('Ctrl Pts',(-47.747314955179,187.718064100236,-67.6430387914656));
#20919=CARTESIAN_POINT('Ctrl Pts',(-48.3997417071708,187.726644621486,-67.5430866920454));
#20920=CARTESIAN_POINT('Ctrl Pts',(-49.051045556932,187.732055009666,-67.4395736529904));
#20921=CARTESIAN_POINT('Ctrl Pts',(-49.3882561779941,187.734856221971,-67.3859800864844));
#20922=CARTESIAN_POINT('Ctrl Pts',(-49.7251654725643,187.736807214015,-67.331431509529));
#20923=CARTESIAN_POINT('Ctrl Pts',(-50.0615611195167,187.737908013141,-67.2759403248462));
#20924=CARTESIAN_POINT('Ctrl Pts',(-50.6474554155661,187.739825255337,-67.1792923186035));
#20925=CARTESIAN_POINT('Ctrl Pts',(-51.2324498655741,187.739178946069,-67.0796996497906));
#20926=CARTESIAN_POINT('Ctrl Pts',(-51.8169655883217,187.735991706155,-66.9769680882559));
#20927=CARTESIAN_POINT('Ctrl Pts',(-52.8892222062581,187.730144918877,-66.7885136251172));
#20928=CARTESIAN_POINT('Ctrl Pts',(-53.958658043911,187.715757546733,-66.589710153915));
#20929=CARTESIAN_POINT('Ctrl Pts',(-55.025126049737,187.692983980761,-66.3798156662999));
#20930=CARTESIAN_POINT('Ctrl Pts',(-55.3182459502838,187.686724641188,-66.3221259362761));
#20931=CARTESIAN_POINT('Ctrl Pts',(-55.6111414887107,187.679831757017,-66.2635981034966));
#20932=CARTESIAN_POINT('Ctrl Pts',(-55.9038092350969,187.67230848245,-66.2042161775242));
#20933=CARTESIAN_POINT('Ctrl Pts',(-56.3020859570986,187.662070438901,-66.123406320222));
#20934=CARTESIAN_POINT('Ctrl Pts',(-56.6999420224511,187.650664478993,-66.0410161314753));
#20935=CARTESIAN_POINT('Ctrl Pts',(-57.0973581429572,187.638100024657,-65.9569932475349));
#20936=CARTESIAN_POINT('Ctrl Pts',(-57.9831815087046,187.610094398679,-65.7697098686999));
#20937=CARTESIAN_POINT('Ctrl Pts',(-58.8667491346833,187.576343097077,-65.5743373152664));
#20938=CARTESIAN_POINT('Ctrl Pts',(-59.748022636317,187.536944885931,-65.3702357907628));
#20939=CARTESIAN_POINT('Ctrl Pts',(-60.3701587719641,187.509131669276,-65.226150063121));
#20940=CARTESIAN_POINT('Ctrl Pts',(-60.9911510499064,187.478503994181,-65.0777132914352));
#20941=CARTESIAN_POINT('Ctrl Pts',(-61.6109773508216,187.445093862065,-64.9246875207813));
#20942=CARTESIAN_POINT('Ctrl Pts',(-62.4246579959206,187.401234513386,-64.7238020346402));
#20943=CARTESIAN_POINT('Ctrl Pts',(-63.2363399885754,187.352576836396,-64.5150207754862));
#20944=CARTESIAN_POINT('Ctrl Pts',(-64.0458122363587,187.299219962311,-64.2976170779646));
#20945=CARTESIAN_POINT('Ctrl Pts',(-64.8354194022501,187.247172507637,-64.0855486371695));
#20946=CARTESIAN_POINT('Ctrl Pts',(-65.6229240187697,187.190653571721,-63.8652758490625));
#20947=CARTESIAN_POINT('Ctrl Pts',(-66.4081014307383,187.129752250111,-63.6360837689149));
#20948=CARTESIAN_POINT('Ctrl Pts',(-66.6607827592823,187.110153333204,-63.5623264773516));
#20949=CARTESIAN_POINT('Ctrl Pts',(-66.9132228410625,187.090100539921,-63.4876451395221));
#20950=CARTESIAN_POINT('Ctrl Pts',(-67.1654135146365,187.06959679849,-63.4120149817037));
#20951=CARTESIAN_POINT('Ctrl Pts',(-67.2763479110417,187.060577550682,-63.3787465590903));
#20952=CARTESIAN_POINT('Ctrl Pts',(-67.3872335922792,187.051471155586,-63.3452940284817));
#20953=CARTESIAN_POINT('Ctrl Pts',(-67.4980694122349,187.042277973773,-63.3116547642332));
#20954=CARTESIAN_POINT('Ctrl Pts',(-68.1891623934665,186.984955860499,-63.1019043475792));
#20955=CARTESIAN_POINT('Ctrl Pts',(-68.8784061259738,186.92425066319,-62.8848692013738));
#20956=CARTESIAN_POINT('Ctrl Pts',(-69.5656014077318,186.860244783527,-62.6598608171745));
#20957=CARTESIAN_POINT('Ctrl Pts',(-69.6694849243805,186.85056899552,-62.6258462323156));
#20958=CARTESIAN_POINT('Ctrl Pts',(-69.7733215727291,186.840817773274,-62.591649360303));
#20959=CARTESIAN_POINT('Ctrl Pts',(-69.8771106036008,186.83099139587,-62.5572677367493));
#20960=CARTESIAN_POINT('Ctrl Pts',(-69.9376320137037,186.825261443372,-62.5372191408464));
#20961=CARTESIAN_POINT('Ctrl Pts',(-69.9981396362794,186.819505511523,-62.5171063931954));
#20962=CARTESIAN_POINT('Ctrl Pts',(-70.0586302384664,186.813724031626,-62.4969301244232));
#20963=CARTESIAN_POINT('Ctrl Pts',(-70.4373401605021,186.777528263659,-62.3706137563026));
#20964=CARTESIAN_POINT('Ctrl Pts',(-70.8154187338308,186.740326306256,-62.2417960880244));
#20965=CARTESIAN_POINT('Ctrl Pts',(-71.1924802640547,186.70217904041,-62.1104779549871));
#20966=CARTESIAN_POINT('Ctrl Pts',(-71.5383672842266,186.66718569568,-61.9900168787701));
#20967=CARTESIAN_POINT('Ctrl Pts',(-71.883398906256,186.631396708284,-61.8674513360236));
#20968=CARTESIAN_POINT('Ctrl Pts',(-72.22723352361,186.594856854709,-61.7427730099849));
#20969=CARTESIAN_POINT('Ctrl Pts',(-72.3285124818555,186.584093778166,-61.7060481127824));
#20970=CARTESIAN_POINT('Ctrl Pts',(-72.4296872512436,186.573265547093,-61.6691398576058));
#20971=CARTESIAN_POINT('Ctrl Pts',(-72.53074821145,186.562373297712,-61.6320479328138));
#20972=CARTESIAN_POINT('Ctrl Pts',(-72.5524850931717,186.560030518304,-61.624069948235));
#20973=CARTESIAN_POINT('Ctrl Pts',(-72.5742182031628,186.557684636607,-61.6160830365718));
#20974=CARTESIAN_POINT('Ctrl Pts',(-72.5959475943732,186.555335651049,-61.6080871405041));
#20975=CARTESIAN_POINT('Ctrl Pts',(-73.0750811308316,186.503540469726,-61.4317774628443));
#20976=CARTESIAN_POINT('Ctrl Pts',(-73.5520260771487,186.450278236732,-61.2512439961753));
#20977=CARTESIAN_POINT('Ctrl Pts',(-74.0266639966632,186.39561293057,-61.0661252075006));
#20978=CARTESIAN_POINT('Ctrl Pts',(-74.4933003459508,186.341869186442,-60.8841271997981));
#20979=CARTESIAN_POINT('Ctrl Pts',(-74.9577069279405,186.286769176235,-60.6976972459528));
#20980=CARTESIAN_POINT('Ctrl Pts',(-75.4197294652055,186.230378252862,-60.5064652710687));
#20981=CARTESIAN_POINT('Ctrl Pts',(-75.870278313599,186.175387719854,-60.3199822770354));
#20982=CARTESIAN_POINT('Ctrl Pts',(-76.3185601193047,186.119169509541,-60.1289328394813));
#20983=CARTESIAN_POINT('Ctrl Pts',(-76.7643904712269,186.061789933078,-59.9329475682572));
#20984=CARTESIAN_POINT('Ctrl Pts',(-77.0251398082259,186.028230785622,-59.8183231840874));
#20985=CARTESIAN_POINT('Ctrl Pts',(-77.285049808661,185.994274490326,-59.7020099337784));
#20986=CARTESIAN_POINT('Ctrl Pts',(-77.5440766099974,185.959935431812,-59.5839295084219));
#20987=CARTESIAN_POINT('Ctrl Pts',(-77.5450711085164,185.959803591622,-59.5834761545314));
#20988=CARTESIAN_POINT('Ctrl Pts',(-77.5460655939007,185.959671745816,-59.5830227745252));
#20989=CARTESIAN_POINT('Ctrl Pts',(-77.5470600661468,185.959539894396,-59.582569368398));
#20990=CARTESIAN_POINT('Ctrl Pts',(-77.9410693805506,185.907300440083,-59.4029301295733));
#20991=CARTESIAN_POINT('Ctrl Pts',(-78.332979228556,185.85418497661,-59.2192124213913));
#20992=CARTESIAN_POINT('Ctrl Pts',(-78.7227006320066,185.800243549814,-59.0310068937098));
#20993=CARTESIAN_POINT('Ctrl Pts',(-79.0870092104663,185.749819517821,-58.8550738101255));
#20994=CARTESIAN_POINT('Ctrl Pts',(-79.4494052396861,185.698673675177,-58.6752189694766));
#20995=CARTESIAN_POINT('Ctrl Pts',(-79.8097729729191,185.646852044688,-58.4910808942653));
#20996=CARTESIAN_POINT('Ctrl Pts',(-79.8349108990578,185.64323715856,-58.4782361001644));
#20997=CARTESIAN_POINT('Ctrl Pts',(-79.860038937817,185.639618986481,-58.4653704529016));
#20998=CARTESIAN_POINT('Ctrl Pts',(-79.8851570418036,185.635997545186,-58.4524838246918));
#20999=CARTESIAN_POINT('Ctrl Pts',(-80.2271667926614,185.586687763051,-58.2770186500199));
#21000=CARTESIAN_POINT('Ctrl Pts',(-80.5673404844472,185.536770724644,-58.097667248913));
#21001=CARTESIAN_POINT('Ctrl Pts',(-80.905487185369,185.486304601332,-57.9140644289558));
#21002=CARTESIAN_POINT('Ctrl Pts',(-81.2350552092114,185.43711878794,-57.7351195556797));
#21003=CARTESIAN_POINT('Ctrl Pts',(-81.5626978743657,185.387411331872,-57.552136292134));
#21004=CARTESIAN_POINT('Ctrl Pts',(-81.8881965724081,185.337243380279,-57.3647505333222));
#21005=CARTESIAN_POINT('Ctrl Pts',(-81.9594892979342,185.326255287163,-57.3237081526589));
#21006=CARTESIAN_POINT('Ctrl Pts',(-82.030679006116,185.315245133469,-57.2824544704765));
#21007=CARTESIAN_POINT('Ctrl Pts',(-82.1017631156658,185.304213614831,-57.2409854846495));
#21008=CARTESIAN_POINT('Ctrl Pts',(-82.1641085977492,185.294538240799,-57.2046144316918));
#21009=CARTESIAN_POINT('Ctrl Pts',(-82.2263725660917,185.284846503345,-57.1680775913122));
#21010=CARTESIAN_POINT('Ctrl Pts',(-82.2885528589849,185.275138973569,-57.1313720132604));
#21011=CARTESIAN_POINT('Ctrl Pts',(-82.5537094566501,185.233742970956,-56.9748477233497));
#21012=CARTESIAN_POINT('Ctrl Pts',(-82.8173085533163,185.192065700995,-56.815280772334));
#21013=CARTESIAN_POINT('Ctrl Pts',(-83.0793493574573,185.15012491829,-56.6523178031346));
#21014=CARTESIAN_POINT('Ctrl Pts',(-83.1059294390114,185.145870659384,-56.6357876714026));
#21015=CARTESIAN_POINT('Ctrl Pts',(-83.1324934497333,185.141613693795,-56.6192225744983));
#21016=CARTESIAN_POINT('Ctrl Pts',(-83.1590413630191,185.137354043298,-56.6026221275495));
#21017=CARTESIAN_POINT('Ctrl Pts',(-83.3477570764781,185.107074338296,-56.4846179305355));
#21018=CARTESIAN_POINT('Ctrl Pts',(-83.5358233772913,185.076631188317,-56.3647122352436));
#21019=CARTESIAN_POINT('Ctrl Pts',(-83.7227350501772,185.04611606651,-56.2430899760604));
#21020=CARTESIAN_POINT('Ctrl Pts',(-83.8754267602103,185.021187681574,-56.1437344331665));
#21021=CARTESIAN_POINT('Ctrl Pts',(-84.0273472610658,184.996211366635,-56.0432334924026));
#21022=CARTESIAN_POINT('Ctrl Pts',(-84.1781966533824,184.971240983028,-55.941695692402));
#21023=CARTESIAN_POINT('Ctrl Pts',(-84.3028452567794,184.950607665286,-55.8577938299702));
#21024=CARTESIAN_POINT('Ctrl Pts',(-84.4268258047856,184.929968681078,-55.7731493348459));
#21025=CARTESIAN_POINT('Ctrl Pts',(-84.550121873792,184.90933042457,-55.6877257199939));
#21026=CARTESIAN_POINT('Ctrl Pts',(-84.7876740654026,184.869567088205,-55.5231416656365));
#21027=CARTESIAN_POINT('Ctrl Pts',(-85.0226597642961,184.829811900678,-55.35568886156));
#21028=CARTESIAN_POINT('Ctrl Pts',(-85.2549076799668,184.790120644856,-55.1851091265834));
#21029=CARTESIAN_POINT('Ctrl Pts',(-85.4820939782465,184.751294421344,-55.0182470109903));
#21030=CARTESIAN_POINT('Ctrl Pts',(-85.7066606083177,184.712529308532,-54.8483927990932));
#21031=CARTESIAN_POINT('Ctrl Pts',(-85.9284004963375,184.673887791977,-54.6752898962077));
#21032=CARTESIAN_POINT('Ctrl Pts',(-85.9743358203938,184.665882869629,-54.6394301417443));
#21033=CARTESIAN_POINT('Ctrl Pts',(-86.0201496699684,184.657883289184,-54.60343091788));
#21034=CARTESIAN_POINT('Ctrl Pts',(-86.0658399404311,184.64988966699,-54.5672898593966));
#21035=CARTESIAN_POINT('Ctrl Pts',(-86.2709553449911,184.614004235942,-54.405043329512));
#21036=CARTESIAN_POINT('Ctrl Pts',(-86.4735852521456,184.578237776751,-54.2399399631925));
#21037=CARTESIAN_POINT('Ctrl Pts',(-86.6734831582947,184.542656686666,-54.0717480448259));
#21038=CARTESIAN_POINT('Ctrl Pts',(-86.8570706538062,184.509978789523,-53.9172795281064));
#21039=CARTESIAN_POINT('Ctrl Pts',(-87.0383425977796,184.477460157983,-53.7602184288664));
#21040=CARTESIAN_POINT('Ctrl Pts',(-87.2171464938128,184.445147523806,-53.6003097299749));
#21041=CARTESIAN_POINT('Ctrl Pts',(-87.3923292574055,184.413489284362,-53.4436394984206));
#21042=CARTESIAN_POINT('Ctrl Pts',(-87.5651430323094,184.382028724284,-53.2842358707506));
#21043=CARTESIAN_POINT('Ctrl Pts',(-87.7353991285702,184.350819525833,-53.1218444821961));
#21044=CARTESIAN_POINT('Ctrl Pts',(-87.8984589116787,184.320929464671,-52.9663169846326));
#21045=CARTESIAN_POINT('Ctrl Pts',(-88.0591750208179,184.291269544404,-52.8080497256244));
#21046=CARTESIAN_POINT('Ctrl Pts',(-88.2173066844818,184.261901670574,-52.6467953084342));
#21047=CARTESIAN_POINT('Ctrl Pts',(-88.3489258435748,184.237457642298,-52.51257695963));
#21048=CARTESIAN_POINT('Ctrl Pts',(-88.478753822866,184.213216087887,-52.3762889160388));
#21049=CARTESIAN_POINT('Ctrl Pts',(-88.6066260845763,184.189218592662,-52.2377803000698));
#21050=CARTESIAN_POINT('Ctrl Pts',(-88.7423987435818,184.163738447926,-52.0907141354948));
#21051=CARTESIAN_POINT('Ctrl Pts',(-88.8759595521882,184.138535045677,-51.9411553279166));
#21052=CARTESIAN_POINT('Ctrl Pts',(-89.007139024002,184.113653620594,-51.7888395413096));
#21053=CARTESIAN_POINT('Ctrl Pts',(-89.0610951115254,184.103419516653,-51.7261897699718));
#21054=CARTESIAN_POINT('Ctrl Pts',(-89.1146477662933,184.093240005199,-51.6630733955921));
#21055=CARTESIAN_POINT('Ctrl Pts',(-89.1677827797996,184.083118761996,-51.5994712579033));
#21056=CARTESIAN_POINT('Ctrl Pts',(-89.2735870907887,184.062964985931,-51.4728244404557));
#21057=CARTESIAN_POINT('Ctrl Pts',(-89.3778592759144,184.043017998514,-51.3440714967514));
#21058=CARTESIAN_POINT('Ctrl Pts',(-89.4802240523979,184.02335791968,-51.2133748814786));
#21059=CARTESIAN_POINT('Ctrl Pts',(-89.5846662384106,184.003298855603,-51.0800258851492));
#21060=CARTESIAN_POINT('Ctrl Pts',(-89.6871213991053,183.983539255981,-50.9446550233047));
#21061=CARTESIAN_POINT('Ctrl Pts',(-89.787050816559,183.964192805037,-50.8075906059771));
#21062=CARTESIAN_POINT('Ctrl Pts',(-89.9538329812593,183.931903584806,-50.5788301387615));
#21063=CARTESIAN_POINT('Ctrl Pts',(-90.1134653217683,183.900788683591,-50.3455986429249));
#21064=CARTESIAN_POINT('Ctrl Pts',(-90.2649122865753,183.871104542861,-50.107908393505));
#21065=CARTESIAN_POINT('Ctrl Pts',(-90.2869520658823,183.866784668168,-50.0733177983925));
#21066=CARTESIAN_POINT('Ctrl Pts',(-90.3088215648408,183.86249445937,-50.0386276981052));
#21067=CARTESIAN_POINT('Ctrl Pts',(-90.3305184659637,183.858234565329,-50.0038364107849));
#21068=CARTESIAN_POINT('Ctrl Pts',(-90.4388801877854,183.836959202068,-49.830076859729));
#21069=CARTESIAN_POINT('Ctrl Pts',(-90.5429465739695,183.816439370396,-49.653794440825));
#21070=CARTESIAN_POINT('Ctrl Pts',(-90.6423754682554,183.796762200223,-49.4747737442102));
#21071=CARTESIAN_POINT('Ctrl Pts',(-90.7359515882384,183.778243305386,-49.306290907242));
#21072=CARTESIAN_POINT('Ctrl Pts',(-90.8254198130981,183.760470832419,-49.1353826443591));
#21073=CARTESIAN_POINT('Ctrl Pts',(-90.9104447973024,183.74352951109,-48.9618638325262));
#21074=CARTESIAN_POINT('Ctrl Pts',(-90.9157627357116,183.742469906032,-48.9510109948243));
#21075=CARTESIAN_POINT('Ctrl Pts',(-90.9210632759633,183.741413556434,-48.9401479429578));
#21076=CARTESIAN_POINT('Ctrl Pts',(-90.9263463293841,183.740360484662,-48.9292746308957));
#21077=CARTESIAN_POINT('Ctrl Pts',(-90.9852403645883,183.72862112845,-48.8080619206772));
#21078=CARTESIAN_POINT('Ctrl Pts',(-91.0421061938172,183.717259001773,-48.6852599408307));
#21079=CARTESIAN_POINT('Ctrl Pts',(-91.0966291024536,183.706343449781,-48.5611616805563));
#21080=CARTESIAN_POINT('Ctrl Pts',(-91.1243382887326,183.700796037307,-48.4980934786416));
#21081=CARTESIAN_POINT('Ctrl Pts',(-91.1514431441962,183.695363828463,-48.4346905584647));
#21082=CARTESIAN_POINT('Ctrl Pts',(-91.1779074466647,183.690055029156,-48.3709919142252));
#21083=CARTESIAN_POINT('Ctrl Pts',(-91.2289358904181,183.679818607202,-48.2481682468109));
#21084=CARTESIAN_POINT('Ctrl Pts',(-91.2775802069475,183.670041568329,-48.1242448232095));
#21085=CARTESIAN_POINT('Ctrl Pts',(-91.3236087361308,183.660775010778,-47.9995040966891));
#21086=CARTESIAN_POINT('Ctrl Pts',(-91.3642312992659,183.652596793359,-47.8894139389433));
#21087=CARTESIAN_POINT('Ctrl Pts',(-91.4028170594171,183.644816079972,-47.778687252021));
#21088=CARTESIAN_POINT('Ctrl Pts',(-91.4392397760242,183.637461709821,-47.6675216693592));
#21089=CARTESIAN_POINT('Ctrl Pts',(-91.5301427046272,183.619106852,-47.3900773169012));
#21090=CARTESIAN_POINT('Ctrl Pts',(-91.6075721796016,183.603408457479,-47.1099727365793));
#21091=CARTESIAN_POINT('Ctrl Pts',(-91.6708671314707,183.590553705567,-46.8270612872151));
#21092=CARTESIAN_POINT('Ctrl Pts',(-91.6800654005284,183.588685602926,-46.7859474929247));
#21093=CARTESIAN_POINT('Ctrl Pts',(-91.6889650755193,183.586877577863,-46.744774411718));
#21094=CARTESIAN_POINT('Ctrl Pts',(-91.6975640385099,183.585130228127,-46.7035415847502));
#21095=CARTESIAN_POINT('Ctrl Pts',(-91.7555966293713,183.573337732632,-46.4252699163973));
#21096=CARTESIAN_POINT('Ctrl Pts',(-91.7999412124509,183.56430768583,-46.1442769510425));
#21097=CARTESIAN_POINT('Ctrl Pts',(-91.8297919983774,183.558222566852,-45.8604063906217));
#21098=CARTESIAN_POINT('Ctrl Pts',(-91.8596427843038,183.552137447875,-45.576535830201));
#21099=CARTESIAN_POINT('Ctrl Pts',(-91.8749999999089,183.548997205095,-45.2897876967856));
#21100=CARTESIAN_POINT('Ctrl Pts',(-91.875,183.548997205106,-45.));
#21101=CARTESIAN_POINT('Origin',(-40.3363668356791,225.625863228014,34.2057557851749));
#21102=CARTESIAN_POINT('Origin',(-133.630782057879,206.966980183574,47.2669739162829));
#21103=CARTESIAN_POINT('Ctrl Pts',(-128.727878679424,182.452463291301,47.2669739162829));
#21104=CARTESIAN_POINT('Ctrl Pts',(-125.483223478439,183.101394331498,71.37012683789));
#21105=CARTESIAN_POINT('Ctrl Pts',(-130.164585944519,206.966980183574,72.0255175831412));
#21106=CARTESIAN_POINT('Ctrl Pts',(-126.868199058258,182.824399215534,46.9474471450068));
#21107=CARTESIAN_POINT('Ctrl Pts',(-123.591604530024,183.421472951552,71.1053001850989));
#21108=CARTESIAN_POINT('Ctrl Pts',(-127.882251854987,207.423447001473,71.7059908106067));
#21109=CARTESIAN_POINT('Ctrl Pts',(-124.998899886252,183.148230114533,46.626267559976));
#21110=CARTESIAN_POINT('Ctrl Pts',(-121.695019586642,183.691462296002,70.8397782930618));
#21111=CARTESIAN_POINT('Ctrl Pts',(-125.588111971157,207.820875830351,71.3848112268705));
#21112=CARTESIAN_POINT('Ctrl Pts',(-123.122478208265,183.423523407144,46.3038641989655));
#21113=CARTESIAN_POINT('Ctrl Pts',(-119.79626063639,183.911518935037,70.5739520400031));
#21114=CARTESIAN_POINT('Ctrl Pts',(-123.285230820823,208.15873578029,71.0624078658238));
#21115=CARTESIAN_POINT('Origin',(-126.751426934183,208.15873578029,46.3038641989655));
#21116=CARTESIAN_POINT('Ctrl Pts',(-108.033967922038,209.585728186396,70.));
#21117=CARTESIAN_POINT('Ctrl Pts',(-107.87121530948,184.586257960267,70.));
#21118=CARTESIAN_POINT('Ctrl Pts',(-107.87121530948,184.586257960267,45.));
#21119=CARTESIAN_POINT('Ctrl Pts',(-110.601673611534,209.565212621119,70.));
#21120=CARTESIAN_POINT('Ctrl Pts',(-109.85516797587,184.573341947487,69.9962013003751));
#21121=CARTESIAN_POINT('Ctrl Pts',(-110.438920857634,184.569541574581,44.9999999999672));
#21122=CARTESIAN_POINT('Ctrl Pts',(-113.15629663918,209.434596373781,70.0897908380021));
#21123=CARTESIAN_POINT('Ctrl Pts',(-111.827042166278,184.512020248025,70.0409090865197));
#21124=CARTESIAN_POINT('Ctrl Pts',(-112.993544026618,184.463113520352,45.1101978466734));
#21125=CARTESIAN_POINT('Ctrl Pts',(-118.239922397535,208.957898622415,70.4448503138047));
#21126=CARTESIAN_POINT('Ctrl Pts',(-115.791831475939,184.289393680222,70.2300552342761));
#21127=CARTESIAN_POINT('Ctrl Pts',(-118.077169784981,184.074693130363,45.5459526578167));
#21128=CARTESIAN_POINT('Ctrl Pts',(-120.768938161246,208.611807987957,70.7101268934829));
#21129=CARTESIAN_POINT('Ctrl Pts',(-117.778521014579,184.128732905726,70.3739036490886));
#21130=CARTESIAN_POINT('Ctrl Pts',(-120.606185416313,183.792693373572,45.8715193465168));
#21131=CARTESIAN_POINT('Ctrl Pts',(-123.285230820823,208.15873578029,71.0624078658237));
#21132=CARTESIAN_POINT('Ctrl Pts',(-119.79626063639,183.911518935037,70.5739520400031));
#21133=CARTESIAN_POINT('Ctrl Pts',(-123.122478208265,183.423523407144,46.3038641989654));
#21134=CARTESIAN_POINT('Origin',(-108.033967922038,209.585728186396,45.0000000000001));
#21135=CARTESIAN_POINT('Origin',(-107.155103814224,74.5885889652995,45.0000000000001));
#21136=CARTESIAN_POINT('Origin',(-93.0342906798268,208.848049102839,45.0000000000001));
#21137=CARTESIAN_POINT('Origin',(-115.,0.,45.0000000000001));
#21138=CARTESIAN_POINT('Ctrl Pts',(-91.875,183.548997205106,45.0000000000001));
#21139=CARTESIAN_POINT('Ctrl Pts',(-91.8749999998576,183.548997205088,45.2896000759332));
#21140=CARTESIAN_POINT('Ctrl Pts',(-91.8596625980027,183.552133377192,45.5762242871697));
#21141=CARTESIAN_POINT('Ctrl Pts',(-91.8298318968589,183.558214394318,45.8600283115351));
#21142=CARTESIAN_POINT('Ctrl Pts',(-91.8000011957152,183.564295411445,46.1438323359004));
#21143=CARTESIAN_POINT('Ctrl Pts',(-91.7556769885713,183.573321320276,46.4248161529088));
#21144=CARTESIAN_POINT('Ctrl Pts',(-91.6976496523008,183.585112765732,46.7031300609794));
#21145=CARTESIAN_POINT('Ctrl Pts',(-91.637369668756,183.5973619604,46.9922482400498));
#21146=CARTESIAN_POINT('Ctrl Pts',(-91.5622974063693,183.61259559088,47.2784857624134));
#21147=CARTESIAN_POINT('Ctrl Pts',(-91.473124343595,183.630616797189,47.561991552747));
#21148=CARTESIAN_POINT('Ctrl Pts',(-91.4617400188155,183.632917483733,47.598185464828));
#21149=CARTESIAN_POINT('Ctrl Pts',(-91.4501258054148,183.635263621029,47.6343348470904));
#21150=CARTESIAN_POINT('Ctrl Pts',(-91.4382830838388,183.63765481468,47.6704400035409));
#21151=CARTESIAN_POINT('Ctrl Pts',(-91.4056950676103,183.644234742865,47.7697917798027));
#21152=CARTESIAN_POINT('Ctrl Pts',(-91.3713189504872,183.651167837988,47.8689747154106));
#21153=CARTESIAN_POINT('Ctrl Pts',(-91.3353086631554,183.658420153658,47.9676327090243));
#21154=CARTESIAN_POINT('Ctrl Pts',(-91.2989262398865,183.665747415892,48.0673102497624));
#21155=CARTESIAN_POINT('Ctrl Pts',(-91.2608757374785,183.673400509824,48.1664519468418));
#21156=CARTESIAN_POINT('Ctrl Pts',(-91.2213678244624,183.681334352256,48.2646960569366));
#21157=CARTESIAN_POINT('Ctrl Pts',(-91.2150232933313,183.682608439051,48.2804729676201));
#21158=CARTESIAN_POINT('Ctrl Pts',(-91.2086412839471,183.683889745562,48.2962267419502));
#21159=CARTESIAN_POINT('Ctrl Pts',(-91.2022227901124,183.685178061878,48.3119558946997));
#21160=CARTESIAN_POINT('Ctrl Pts',(-91.1943916959767,183.686749914498,48.3311467639331));
#21161=CARTESIAN_POINT('Ctrl Pts',(-91.1865048506322,183.688332493241,48.3503045398201));
#21162=CARTESIAN_POINT('Ctrl Pts',(-91.1785628076855,183.689925674695,48.3694295168963));
#21163=CARTESIAN_POINT('Ctrl Pts',(-91.1087363643921,183.703932926374,48.5375763194571));
#21164=CARTESIAN_POINT('Ctrl Pts',(-91.034646476792,183.718758774971,48.7031880996127));
#21165=CARTESIAN_POINT('Ctrl Pts',(-90.9566165291512,183.734324372969,48.8664595502886));
#21166=CARTESIAN_POINT('Ctrl Pts',(-90.9461168373726,183.73641887625,48.8884293190783));
#21167=CARTESIAN_POINT('Ctrl Pts',(-90.9355457310213,183.738526792029,48.9103567058832));
#21168=CARTESIAN_POINT('Ctrl Pts',(-90.9249039291036,183.7406479451,48.932242178386));
#21169=CARTESIAN_POINT('Ctrl Pts',(-90.8406028436605,183.757451068078,49.1056121679495));
#21170=CARTESIAN_POINT('Ctrl Pts',(-90.7518683910998,183.775084743858,49.2763588350715));
#21171=CARTESIAN_POINT('Ctrl Pts',(-90.6590379490552,183.793463886533,49.4446683780763));
#21172=CARTESIAN_POINT('Ctrl Pts',(-90.5646175021781,183.812157828158,49.6158607360375));
#21173=CARTESIAN_POINT('Ctrl Pts',(-90.4659594745685,183.831623035935,49.7845317587114));
#21174=CARTESIAN_POINT('Ctrl Pts',(-90.3633670717736,183.85178248117,49.9508715143199));
#21175=CARTESIAN_POINT('Ctrl Pts',(-90.3531584694818,183.85378847531,49.9674233872078));
#21176=CARTESIAN_POINT('Ctrl Pts',(-90.3429108698052,183.85580135319,49.9839521723536));
#21177=CARTESIAN_POINT('Ctrl Pts',(-90.33262454449,183.857821045285,50.0004580539773));
#21178=CARTESIAN_POINT('Ctrl Pts',(-90.3098775310987,183.862287359708,50.0369588935699));
#21179=CARTESIAN_POINT('Ctrl Pts',(-90.2869409228782,183.866786973872,50.073347705516));
#21180=CARTESIAN_POINT('Ctrl Pts',(-90.2638174075046,183.871319137022,50.1096264538567));
#21181=CARTESIAN_POINT('Ctrl Pts',(-90.1478268110307,183.894053063871,50.2916054302969));
#21182=CARTESIAN_POINT('Ctrl Pts',(-90.0271359963355,183.917606706893,50.4708248827606));
#21183=CARTESIAN_POINT('Ctrl Pts',(-89.902092931984,183.941887340518,50.6474690155926));
#21184=CARTESIAN_POINT('Ctrl Pts',(-89.8652183685416,183.949047575831,50.6995604715772));
#21185=CARTESIAN_POINT('Ctrl Pts',(-89.8279649867759,183.956271120596,50.7514279342131));
#21186=CARTESIAN_POINT('Ctrl Pts',(-89.790340884684,183.963555813154,50.8030760387775));
#21187=CARTESIAN_POINT('Ctrl Pts',(-89.6982015750568,183.981395615459,50.9295593415947));
#21188=CARTESIAN_POINT('Ctrl Pts',(-89.6037507212967,183.999618439847,51.0548132891789));
#21189=CARTESIAN_POINT('Ctrl Pts',(-89.5074065290439,184.018135337854,51.1785589171201));
#21190=CARTESIAN_POINT('Ctrl Pts',(-89.4981849683562,184.019907678197,51.1904031994915));
#21191=CARTESIAN_POINT('Ctrl Pts',(-89.4889460311051,184.021682719221,51.2022336866468));
#21192=CARTESIAN_POINT('Ctrl Pts',(-89.4796900645198,184.023460387051,51.2140501483047));
#21193=CARTESIAN_POINT('Ctrl Pts',(-89.3862338429122,184.041409254643,51.3333593365078));
#21194=CARTESIAN_POINT('Ctrl Pts',(-89.2911914529099,184.059596578161,51.4510479915178));
#21195=CARTESIAN_POINT('Ctrl Pts',(-89.1948816910292,184.077954977797,51.5669472071899));
#21196=CARTESIAN_POINT('Ctrl Pts',(-89.1870865088545,184.079440881892,51.5763279333222));
#21197=CARTESIAN_POINT('Ctrl Pts',(-89.1792830000548,184.08092791161,51.5856969503268));
#21198=CARTESIAN_POINT('Ctrl Pts',(-89.1714713212156,184.082416033757,51.5950541756226));
#21199=CARTESIAN_POINT('Ctrl Pts',(-89.0488267301808,184.105779786404,51.7419640900277));
#21200=CARTESIAN_POINT('Ctrl Pts',(-88.9240271148734,184.129440547651,51.8861994560237));
#21201=CARTESIAN_POINT('Ctrl Pts',(-88.7972002069489,184.153362762024,52.0280454940487));
#21202=CARTESIAN_POINT('Ctrl Pts',(-88.7335807470613,184.165362726249,52.0991989146755));
#21203=CARTESIAN_POINT('Ctrl Pts',(-88.6694503783405,184.177428643762,52.169750856651));
#21204=CARTESIAN_POINT('Ctrl Pts',(-88.6048206625496,184.189556961584,52.2397358175433));
#21205=CARTESIAN_POINT('Ctrl Pts',(-88.4520875106276,184.218218641212,52.405124501888));
#21206=CARTESIAN_POINT('Ctrl Pts',(-88.2966148012104,184.24721896858,52.5672961007393));
#21207=CARTESIAN_POINT('Ctrl Pts',(-88.138680219344,184.276488112159,52.7265149727087));
#21208=CARTESIAN_POINT('Ctrl Pts',(-88.0074095306954,184.300815783708,52.8588531264069));
#21209=CARTESIAN_POINT('Ctrl Pts',(-87.8744370528921,184.325329410138,52.9891510658943));
#21210=CARTESIAN_POINT('Ctrl Pts',(-87.7398968895164,184.349994645736,53.1175521934523));
#21211=CARTESIAN_POINT('Ctrl Pts',(-87.5669079643352,184.381708689248,53.2826476749131));
#21212=CARTESIAN_POINT('Ctrl Pts',(-87.3913260249385,184.41367354028,53.4446068601911));
#21213=CARTESIAN_POINT('Ctrl Pts',(-87.2133483459065,184.445833478442,53.6037055710983));
#21214=CARTESIAN_POINT('Ctrl Pts',(-87.0353706668745,184.477993416603,53.7628042820054));
#21215=CARTESIAN_POINT('Ctrl Pts',(-86.8549969608648,184.510348541428,53.9190424247838));
#21216=CARTESIAN_POINT('Ctrl Pts',(-86.6723757709748,184.542853504445,54.0726796240347));
#21217=CARTESIAN_POINT('Ctrl Pts',(-86.475292839042,184.577932530146,54.2384833278686));
#21218=CARTESIAN_POINT('Ctrl Pts',(-86.2756058929237,184.613182555372,54.4012426705288));
#21219=CARTESIAN_POINT('Ctrl Pts',(-86.0735521960395,184.648540151242,54.5611869623873));
#21220=CARTESIAN_POINT('Ctrl Pts',(-85.8543878629899,184.686891955918,54.7346759140415));
#21221=CARTESIAN_POINT('Ctrl Pts',(-85.6324370091774,184.725370702841,54.9048521957901));
#21222=CARTESIAN_POINT('Ctrl Pts',(-85.4079128581921,184.763913428892,55.0719790830492));
#21223=CARTESIAN_POINT('Ctrl Pts',(-85.1783322433329,184.803324168032,55.2428698017895));
#21224=CARTESIAN_POINT('Ctrl Pts',(-84.9460610318809,184.842801868036,55.4105722034497));
#21225=CARTESIAN_POINT('Ctrl Pts',(-84.711276707351,184.882290320516,55.5753510661694));
#21226=CARTESIAN_POINT('Ctrl Pts',(-84.6589544714057,184.891090414526,55.6120724211887));
#21227=CARTESIAN_POINT('Ctrl Pts',(-84.6065072349179,184.899891083013,55.6486485206267));
#21228=CARTESIAN_POINT('Ctrl Pts',(-84.5539366380794,184.908691771476,55.6850821875323));
#21229=CARTESIAN_POINT('Ctrl Pts',(-84.4339755441047,184.928774104173,55.7682203446458));
#21230=CARTESIAN_POINT('Ctrl Pts',(-84.3133857020704,184.948853940928,55.8506069627194));
#21231=CARTESIAN_POINT('Ctrl Pts',(-84.1921856924569,184.968924862174,55.9322745501777));
#21232=CARTESIAN_POINT('Ctrl Pts',(-83.9861474492598,185.003045134655,56.0711082540669));
#21233=CARTESIAN_POINT('Ctrl Pts',(-83.7781170348905,185.037173395447,56.2079845765804));
#21234=CARTESIAN_POINT('Ctrl Pts',(-83.568516464438,185.071229092963,56.3428494397901));
#21235=CARTESIAN_POINT('Ctrl Pts',(-83.3489960646454,185.106896554735,56.4840970930091));
#21236=CARTESIAN_POINT('Ctrl Pts',(-83.1277532697727,185.142484462688,56.6231385182653));
#21237=CARTESIAN_POINT('Ctrl Pts',(-82.9052153450518,185.177909732773,56.7599207635829));
#21238=CARTESIAN_POINT('Ctrl Pts',(-82.7026785012987,185.210151079506,56.884409406509));
#21239=CARTESIAN_POINT('Ctrl Pts',(-82.4990678825317,185.242257885112,57.0070269383323));
#21240=CARTESIAN_POINT('Ctrl Pts',(-82.2946689193971,185.274173280065,57.1277380489338));
#21241=CARTESIAN_POINT('Ctrl Pts',(-82.2352099679613,185.283457358074,57.1628524935129));
#21242=CARTESIAN_POINT('Ctrl Pts',(-82.1756788543776,185.292726231422,57.1978089829018));
#21243=CARTESIAN_POINT('Ctrl Pts',(-82.1160839107254,185.301978283238,57.2326055443681));
#21244=CARTESIAN_POINT('Ctrl Pts',(-81.7887439000654,185.352797472826,57.4237342895821));
#21245=CARTESIAN_POINT('Ctrl Pts',(-81.4591756081384,185.403164059862,57.6102890632906));
#21246=CARTESIAN_POINT('Ctrl Pts',(-81.1276197694625,185.453012021079,57.7926461799151));
#21247=CARTESIAN_POINT('Ctrl Pts',(-80.7875849553267,185.504134758942,57.9796667689819));
#21248=CARTESIAN_POINT('Ctrl Pts',(-80.4454595429424,185.554712071923,58.1622722017703));
#21249=CARTESIAN_POINT('Ctrl Pts',(-80.1014577657148,185.604680843576,58.3408392875945));
#21250=CARTESIAN_POINT('Ctrl Pts',(-80.032898979013,185.614639508282,58.3764273093997));
#21251=CARTESIAN_POINT('Ctrl Pts',(-79.9642655255146,185.624574025262,58.4118548409497));
#21252=CARTESIAN_POINT('Ctrl Pts',(-79.8955588980838,185.634483928414,58.4471247348226));
#21253=CARTESIAN_POINT('Ctrl Pts',(-79.5316246154641,185.68697600421,58.6339469382209));
#21254=CARTESIAN_POINT('Ctrl Pts',(-79.1656381332745,185.738777667491,58.81634686547));
#21255=CARTESIAN_POINT('Ctrl Pts',(-78.797734523417,185.78983874123,58.9946950423225));
#21256=CARTESIAN_POINT('Ctrl Pts',(-78.4204446175163,185.842202532152,59.1775934022715));
#21257=CARTESIAN_POINT('Ctrl Pts',(-78.0411384098941,185.893787548864,59.3562305679962));
#21258=CARTESIAN_POINT('Ctrl Pts',(-77.6599161892546,185.944545250797,59.5309767423899));
#21259=CARTESIAN_POINT('Ctrl Pts',(-77.6239543810173,185.949333373432,59.5474610606523));
#21260=CARTESIAN_POINT('Ctrl Pts',(-77.5879754909047,185.95411413746,59.563910733478));
#21261=CARTESIAN_POINT('Ctrl Pts',(-77.5519795834612,185.958887504175,59.5803260588794));
#21262=CARTESIAN_POINT('Ctrl Pts',(-77.5509731104167,185.959020971152,59.5807850439059));
#21263=CARTESIAN_POINT('Ctrl Pts',(-77.5499666241808,185.959154432318,59.5812440021455));
#21264=CARTESIAN_POINT('Ctrl Pts',(-77.5489601247535,185.959287887672,59.581702933604));
#21265=CARTESIAN_POINT('Ctrl Pts',(-77.104093236163,186.018274377647,59.7845479670832));
#21266=CARTESIAN_POINT('Ctrl Pts',(-76.656675622457,186.076124505428,59.9821566691924));
#21267=CARTESIAN_POINT('Ctrl Pts',(-76.2069171712731,186.132768524725,60.1749241646176));
#21268=CARTESIAN_POINT('Ctrl Pts',(-75.7497127441504,186.190350314071,60.3708830222705));
#21269=CARTESIAN_POINT('Ctrl Pts',(-75.2900891958921,186.246685825175,60.5618389662368));
#21270=CARTESIAN_POINT('Ctrl Pts',(-74.8282214571534,186.301708554694,60.7481774544196));
#21271=CARTESIAN_POINT('Ctrl Pts',(-74.3542859546025,186.358168928042,60.9393846283233));
#21272=CARTESIAN_POINT('Ctrl Pts',(-73.8779873816825,186.413247119223,61.1257298593644));
#21273=CARTESIAN_POINT('Ctrl Pts',(-73.3994686781298,186.466876867152,61.3075995918588));
#21274=CARTESIAN_POINT('Ctrl Pts',(-73.1328670620181,186.49675611192,61.4089263827342));
#21275=CARTESIAN_POINT('Ctrl Pts',(-72.8655754995583,186.526185844042,61.5088634323636));
#21276=CARTESIAN_POINT('Ctrl Pts',(-72.597612901913,186.555155155028,61.607473776701));
#21277=CARTESIAN_POINT('Ctrl Pts',(-72.5779166749682,186.557284504902,61.6147219961848));
#21278=CARTESIAN_POINT('Ctrl Pts',(-72.5582170481678,186.559411341513,61.6219629615358));
#21279=CARTESIAN_POINT('Ctrl Pts',(-72.5385140095715,186.561535662791,61.6291967046453));
#21280=CARTESIAN_POINT('Ctrl Pts',(-72.1599131996972,186.602355242599,61.7681956202845));
#21281=CARTESIAN_POINT('Ctrl Pts',(-71.7796564183865,186.642285282424,61.9046445763352));
#21282=CARTESIAN_POINT('Ctrl Pts',(-71.3982081963154,186.681262919249,62.0385496296937));
#21283=CARTESIAN_POINT('Ctrl Pts',(-70.9933353519151,186.722634161206,62.1806777527151));
#21284=CARTESIAN_POINT('Ctrl Pts',(-70.5871199280422,186.762932566114,62.3199401712124));
#21285=CARTESIAN_POINT('Ctrl Pts',(-70.1800592229702,186.802083325186,62.4563372032453));
#21286=CARTESIAN_POINT('Ctrl Pts',(-70.0819837581538,186.811516141584,62.4892001206174));
#21287=CARTESIAN_POINT('Ctrl Pts',(-69.9838589874606,186.8208823333,62.5218966629664));
#21288=CARTESIAN_POINT('Ctrl Pts',(-69.8856914387029,186.830180842981,62.5544267552581));
#21289=CARTESIAN_POINT('Ctrl Pts',(-69.3917334939288,186.876968939349,62.7181111676227));
#21290=CARTESIAN_POINT('Ctrl Pts',(-68.8971169074742,186.922014017036,62.8774716062755));
#21291=CARTESIAN_POINT('Ctrl Pts',(-68.4014114556514,186.965338130696,63.032944115052));
#21292=CARTESIAN_POINT('Ctrl Pts',(-68.1010971848464,186.991585269101,63.1271343502648));
#21293=CARTESIAN_POINT('Ctrl Pts',(-67.8003826648161,187.017200505675,63.2198967397514));
#21294=CARTESIAN_POINT('Ctrl Pts',(-67.4991671307146,187.042186255654,63.3113209645549));
#21295=CARTESIAN_POINT('Ctrl Pts',(-67.3897881220146,187.051259215893,63.3445194219652));
#21296=CARTESIAN_POINT('Ctrl Pts',(-67.2803598516228,187.060247713469,63.3775362262536));
#21297=CARTESIAN_POINT('Ctrl Pts',(-67.1708834291509,187.0691513977,63.4103738904999));
#21298=CARTESIAN_POINT('Ctrl Pts',(-66.3906302403782,187.132609152859,63.6444123406198));
#21299=CARTESIAN_POINT('Ctrl Pts',(-65.6079560695515,187.191753398071,63.8693796059803));
#21300=CARTESIAN_POINT('Ctrl Pts',(-64.8230945608355,187.246495462802,64.0859928487631));
#21301=CARTESIAN_POINT('Ctrl Pts',(-64.0188735114315,187.302587805534,64.3079491142838));
#21302=CARTESIAN_POINT('Ctrl Pts',(-63.2123558151995,187.354058220625,64.5211340667888));
#21303=CARTESIAN_POINT('Ctrl Pts',(-62.4037608425511,187.400808838323,64.7262749266695));
#21304=CARTESIAN_POINT('Ctrl Pts',(-62.1386954729806,187.416134149729,64.7935221142945));
#21305=CARTESIAN_POINT('Ctrl Pts',(-61.8734066350219,187.430952249136,64.8599045480167));
#21306=CARTESIAN_POINT('Ctrl Pts',(-61.6079013555631,187.445259604425,64.9254468698671));
#21307=CARTESIAN_POINT('Ctrl Pts',(-60.7321298652538,187.492452541188,65.1416387926877));
#21308=CARTESIAN_POINT('Ctrl Pts',(-59.8539948749924,187.534092962162,65.3486811914531));
#21309=CARTESIAN_POINT('Ctrl Pts',(-58.9735550061956,187.570087849531,65.5472366543624));
#21310=CARTESIAN_POINT('Ctrl Pts',(-58.3473067264981,187.595690661366,65.6884672159015));
#21311=CARTESIAN_POINT('Ctrl Pts',(-57.7198916747325,187.618437051291,65.8254029884363));
#21312=CARTESIAN_POINT('Ctrl Pts',(-57.0913221019793,187.638290733231,65.9582694164764));
#21313=CARTESIAN_POINT('Ctrl Pts',(-56.6910661901281,187.65093301487,66.0428751238075));
#21314=CARTESIAN_POINT('Ctrl Pts',(-56.2903567688877,187.662400400639,66.1258265383601));
#21315=CARTESIAN_POINT('Ctrl Pts',(-55.8892136405948,187.67268314244,66.2071768544313));
#21316=CARTESIAN_POINT('Ctrl Pts',(-54.8268757205327,187.699914685915,66.4226149848045));
#21317=CARTESIAN_POINT('Ctrl Pts',(-53.7614897889712,187.718841660279,66.6268177710292));
#21318=CARTESIAN_POINT('Ctrl Pts',(-52.6932101568605,187.729309460939,66.8205301740338));
#21319=CARTESIAN_POINT('Ctrl Pts',(-52.3976784406378,187.73220530113,66.8741192879631));
#21320=CARTESIAN_POINT('Ctrl Pts',(-52.1019250975687,187.734453729065,66.9269053030203));
#21321=CARTESIAN_POINT('Ctrl Pts',(-51.8059530143082,187.73605141499,66.9789034094812));
#21322=CARTESIAN_POINT('Ctrl Pts',(-51.2156484509358,187.739237936104,67.0826115673333));
#21323=CARTESIAN_POINT('Ctrl Pts',(-50.6246907854393,187.739834061284,67.183148451155));
#21324=CARTESIAN_POINT('Ctrl Pts',(-50.0325609317261,187.737811001709,67.2807215961937));
#21325=CARTESIAN_POINT('Ctrl Pts',(-49.3669370627525,187.735536843882,67.3904053317819));
#21326=CARTESIAN_POINT('Ctrl Pts',(-48.7005037624025,187.729943847346,67.4962109139689));
#21327=CARTESIAN_POINT('Ctrl Pts',(-48.0342097043618,187.721039705149,67.5981665837054));
#21328=CARTESIAN_POINT('Ctrl Pts',(-47.7114780816944,187.716726822233,67.6475506632078));
#21329=CARTESIAN_POINT('Ctrl Pts',(-47.3887787089,187.711636603788,67.6960309549637));
#21330=CARTESIAN_POINT('Ctrl Pts',(-47.0662186498782,187.705767111222,67.7436074595605));
#21331=CARTESIAN_POINT('Ctrl Pts',(-46.8709828487003,187.702214485745,67.7724040719506));
#21332=CARTESIAN_POINT('Ctrl Pts',(-46.6757335248632,187.698376276571,67.8008803204517));
#21333=CARTESIAN_POINT('Ctrl Pts',(-46.4804497524561,187.694251645111,67.8290426111402));
#21334=CARTESIAN_POINT('Ctrl Pts',(-45.6873485229294,187.677500379801,67.9434174365343));
#21335=CARTESIAN_POINT('Ctrl Pts',(-44.8942928337594,187.656037737837,68.0525249655041));
#21336=CARTESIAN_POINT('Ctrl Pts',(-44.1013097658917,187.629850768109,68.156604155172));
#21337=CARTESIAN_POINT('Ctrl Pts',(-42.1265420022274,187.564637290365,68.4157928276074));
#21338=CARTESIAN_POINT('Ctrl Pts',(-40.1522371157117,187.470128839998,68.6438522044417));
#21339=CARTESIAN_POINT('Ctrl Pts',(-38.1786286591264,187.346091518818,68.8436843142897));
#21340=CARTESIAN_POINT('Ctrl Pts',(-37.3942034702417,187.296791973728,68.9231090552963));
#21341=CARTESIAN_POINT('Ctrl Pts',(-36.6098926799408,187.242833017126,68.9980981274691));
#21342=CARTESIAN_POINT('Ctrl Pts',(-35.8256957544281,187.18419137613,69.0687626934297));
#21343=CARTESIAN_POINT('Ctrl Pts',(-34.0772988235321,187.053447602716,69.2263120362401));
#21344=CARTESIAN_POINT('Ctrl Pts',(-32.3294901451123,186.899468346254,69.3623707313213));
#21345=CARTESIAN_POINT('Ctrl Pts',(-30.5823941605077,186.722004943281,69.4781726760757));
#21346=CARTESIAN_POINT('Ctrl Pts',(-29.1744261304627,186.578988875422,69.571496361476));
#21347=CARTESIAN_POINT('Ctrl Pts',(-27.7669210639304,186.420721359934,69.6516650119064));
#21348=CARTESIAN_POINT('Ctrl Pts',(-26.3599459146534,186.247088364698,69.7193429471197));
#21349=CARTESIAN_POINT('Ctrl Pts',(-25.9684093601055,186.198769341619,69.7381765317683));
#21350=CARTESIAN_POINT('Ctrl Pts',(-25.5769128675606,186.149260825002,69.7560409460401));
#21351=CARTESIAN_POINT('Ctrl Pts',(-25.185456477602,186.098558361674,69.7729424130737));
#21352=CARTESIAN_POINT('Ctrl Pts',(-23.4136314921367,185.869066919834,69.849442483961));
#21353=CARTESIAN_POINT('Ctrl Pts',(-21.6426480519369,185.615155774587,69.9062160012814));
#21354=CARTESIAN_POINT('Ctrl Pts',(-19.8725824218587,185.336465133903,69.9438553294453));
#21355=CARTESIAN_POINT('Ctrl Pts',(-18.1025167917806,185.057774493219,69.9814946576092));
#21356=CARTESIAN_POINT('Ctrl Pts',(-16.3333689159223,184.754304176831,70.));
#21357=CARTESIAN_POINT('Ctrl Pts',(-14.5652173913043,184.425742352699,70.));
#21358=CARTESIAN_POINT('Origin',(3.92135447228743,250.,-28.0096748020595));
#21359=CARTESIAN_POINT('Origin',(-126.751426934183,250.,-46.3038641989654));
#21360=CARTESIAN_POINT('Origin',(-108.033967922038,250.,-180.));
#21361=CARTESIAN_POINT('Origin',(-115.000000000001,250.,-45.1798442476466));
#21362=CARTESIAN_POINT('Ctrl Pts',(-108.033967922038,249.902929948988,-69.9999999999999));
#21363=CARTESIAN_POINT('Ctrl Pts',(-107.337364714242,274.893222943887,-69.9999999999999));
#21364=CARTESIAN_POINT('Ctrl Pts',(-107.337364714242,274.893222943887,-44.9999999999999));
#21365=CARTESIAN_POINT('Ctrl Pts',(-109.926868419224,249.967686392606,-69.9999999999999));
#21366=CARTESIAN_POINT('Ctrl Pts',(-109.462400534848,274.952458214507,-69.988015594096));
#21367=CARTESIAN_POINT('Ctrl Pts',(-109.892780719038,274.964455041348,-44.9999999999515));
#21368=CARTESIAN_POINT('Ctrl Pts',(-111.81888094899,250.000000000097,-70.0488277014676));
#21369=CARTESIAN_POINT('Ctrl Pts',(-111.587915676122,274.988026907036,-70.0368939405427));
#21370=CARTESIAN_POINT('Ctrl Pts',(-112.446996903964,275.,-45.0599248876671));
#21371=CARTESIAN_POINT('Ctrl Pts',(-113.709994059637,250.,-70.1465397573417));
#21372=CARTESIAN_POINT('Ctrl Pts',(-113.709994059638,275.,-70.1465397573417));
#21373=CARTESIAN_POINT('Ctrl Pts',(-115.000000000001,275.,-45.1798442476466));
#21374=CARTESIAN_POINT('Origin',(-108.033967922038,249.902929948988,-44.9999999999999));
#21375=CARTESIAN_POINT('Origin',(-115.,0.,-44.9999999999999));
#21376=CARTESIAN_POINT('Ctrl Pts',(160.,1.95943487863576E-14,-45.));
#21377=CARTESIAN_POINT('Ctrl Pts',(160.,0.241428813471072,-45.0423872342559));
#21378=CARTESIAN_POINT('Ctrl Pts',(159.999569933784,0.485776692267064,-45.0852869669719));
#21379=CARTESIAN_POINT('Ctrl Pts',(159.998704815839,0.729365769049337,-45.1280532951593));
#21380=CARTESIAN_POINT('Ctrl Pts',(159.998619971277,0.753255238303078,-45.1322475098417));
#21381=CARTESIAN_POINT('Ctrl Pts',(159.998530983713,0.777137409236483,-45.1364404414182));
#21382=CARTESIAN_POINT('Ctrl Pts',(159.99843787551,0.801008812615739,-45.1406314806358));
#21383=CARTESIAN_POINT('Ctrl Pts',(159.997395389115,1.06828508400977,-45.1875564694));
#21384=CARTESIAN_POINT('Ctrl Pts',(159.995831384815,1.33549350879009,-45.2344693061509));
#21385=CARTESIAN_POINT('Ctrl Pts',(159.993746619827,1.60263422617359,-45.2813697753231));
#21386=CARTESIAN_POINT('Ctrl Pts',(159.989577089851,2.13691566094059,-45.3751707136674));
#21387=CARTESIAN_POINT('Ctrl Pts',(159.983324543108,2.67092626652068,-45.4689221824702));
#21388=CARTESIAN_POINT('Ctrl Pts',(159.974994723865,3.20466712940897,-45.5626224552081));
#21389=CARTESIAN_POINT('Ctrl Pts',(159.958335085379,4.27214885518554,-45.750023000684));
#21390=CARTESIAN_POINT('Ctrl Pts',(159.933366764185,5.33855161416616,-45.9372187695708));
#21391=CARTESIAN_POINT('Ctrl Pts',(159.900130777316,6.40388332360616,-46.1241959387466));
#21392=CARTESIAN_POINT('Ctrl Pts',(159.844073645198,8.20071398858914,-46.4395590395064));
#21393=CARTESIAN_POINT('Ctrl Pts',(159.764499768404,9.9944985583727,-46.7543004148088));
#21394=CARTESIAN_POINT('Ctrl Pts',(159.66156459619,11.7852683761882,-47.0683529511729));
#21395=CARTESIAN_POINT('Ctrl Pts',(159.642440294338,12.117975086691,-47.1267006993085));
#21396=CARTESIAN_POINT('Ctrl Pts',(159.622509467296,12.4505777513804,-47.1850246736135));
#21397=CARTESIAN_POINT('Ctrl Pts',(159.601772915272,12.7830765913653,-47.2433244470768));
#21398=CARTESIAN_POINT('Ctrl Pts',(159.488946002297,14.5921920913896,-47.5605316404166));
#21399=CARTESIAN_POINT('Ctrl Pts',(159.352270449035,16.3982349599817,-47.8770224280089));
#21400=CARTESIAN_POINT('Ctrl Pts',(159.191844897926,18.201227162187,-48.1927256439253));
#21401=CARTESIAN_POINT('Ctrl Pts',(159.031054793873,20.0083165054632,-48.5091462676101));
#21402=CARTESIAN_POINT('Ctrl Pts',(158.846406606695,21.8123416173502,-48.8247758695827));
#21403=CARTESIAN_POINT('Ctrl Pts',(158.63794737614,23.6133234274148,-49.1395408988029));
#21404=CARTESIAN_POINT('Ctrl Pts',(158.56644346243,24.2310809025642,-49.2475089241488));
#21405=CARTESIAN_POINT('Ctrl Pts',(158.492137565761,24.8484802804144,-49.3553752009994));
#21406=CARTESIAN_POINT('Ctrl Pts',(158.415030182465,25.4655222709345,-49.4631366661702));
#21407=CARTESIAN_POINT('Ctrl Pts',(158.192546930629,27.2459160892981,-49.7740682549364));
#21408=CARTESIAN_POINT('Ctrl Pts',(157.946747091716,29.0233150502689,-50.0841213897866));
#21409=CARTESIAN_POINT('Ctrl Pts',(157.67760762034,30.7977467655214,-50.393226320715));
#21410=CARTESIAN_POINT('Ctrl Pts',(157.408614074615,32.5712163955664,-50.7021636569825));
#21411=CARTESIAN_POINT('Ctrl Pts',(157.116306108476,34.3417222960772,-51.0101539483635));
#21412=CARTESIAN_POINT('Ctrl Pts',(156.800610504028,36.1092800826396,-51.3171210658553));
#21413=CARTESIAN_POINT('Ctrl Pts',(156.48528503735,37.8747654935152,-51.6237282793055));
#21414=CARTESIAN_POINT('Ctrl Pts',(156.146626628634,39.6373099897026,-51.9293148460777));
#21415=CARTESIAN_POINT('Ctrl Pts',(155.784513744485,41.3969127896342,-52.2337964757992));
#21416=CARTESIAN_POINT('Ctrl Pts',(155.423406849553,43.1516272204391,-52.5374322222349));
#21417=CARTESIAN_POINT('Ctrl Pts',(155.038975473555,44.9034165515896,-52.8399692873509));
#21418=CARTESIAN_POINT('Ctrl Pts',(154.631052697224,46.6522595283741,-53.1413137955519));
#21419=CARTESIAN_POINT('Ctrl Pts',(154.329106510401,47.9467605928748,-53.3643702916616));
#21420=CARTESIAN_POINT('Ctrl Pts',(154.01428836003,49.2396469405541,-53.5867731807701));
#21421=CARTESIAN_POINT('Ctrl Pts',(153.686514832082,50.5309013666428,-53.8084801340299));
#21422=CARTESIAN_POINT('Ctrl Pts',(153.459876360839,51.4237371332936,-53.9617790452175));
#21423=CARTESIAN_POINT('Ctrl Pts',(153.226916829294,52.3162715954779,-54.1148283740067));
#21424=CARTESIAN_POINT('Ctrl Pts',(152.987866013332,53.2074993271734,-54.267442333427));
#21425=CARTESIAN_POINT('Ctrl Pts',(152.748770608958,54.0988932931027,-54.4200847588203));
#21426=CARTESIAN_POINT('Ctrl Pts',(152.503581686487,54.9889799168632,-54.5722916107141));
#21427=CARTESIAN_POINT('Ctrl Pts',(152.252579004115,55.8767679003207,-54.7238815612453));
#21428=CARTESIAN_POINT('Ctrl Pts',(152.172094921845,56.1614373724718,-54.772488922468));
#21429=CARTESIAN_POINT('Ctrl Pts',(152.091013469055,56.4458706268006,-54.8210328936362));
#21430=CARTESIAN_POINT('Ctrl Pts',(152.009344941798,56.7300353333953,-54.8695076066916));
#21431=CARTESIAN_POINT('Ctrl Pts',(151.512006252958,58.4605196134401,-55.1647051698487));
#21432=CARTESIAN_POINT('Ctrl Pts',(150.992598450078,60.1821039252991,-55.4575143567747));
#21433=CARTESIAN_POINT('Ctrl Pts',(150.451275564066,61.8948642781311,-55.7478609014618));
#21434=CARTESIAN_POINT('Ctrl Pts',(150.349315513962,62.2174686532709,-55.8025486839458));
#21435=CARTESIAN_POINT('Ctrl Pts',(150.246577836907,62.5397599556456,-55.8571490762826));
#21436=CARTESIAN_POINT('Ctrl Pts',(150.143063362087,62.8617386556575,-55.9116615490075));
#21437=CARTESIAN_POINT('Ctrl Pts',(149.588997306711,64.5851446676367,-56.2034421022505));
#21438=CARTESIAN_POINT('Ctrl Pts',(149.01268050901,66.2995961835638,-56.4927037319273));
#21439=CARTESIAN_POINT('Ctrl Pts',(148.414211986665,68.0051470032801,-56.7793615666974));
#21440=CARTESIAN_POINT('Ctrl Pts',(147.813151839321,69.7180835884611,-57.0672607526555));
#21441=CARTESIAN_POINT('Ctrl Pts',(147.189747552607,71.4220425040294,-57.3525336847906));
#21442=CARTESIAN_POINT('Ctrl Pts',(146.544050740992,73.1170624313016,-57.635082586302));
#21443=CARTESIAN_POINT('Ctrl Pts',(146.3170290416,73.7130175258135,-57.7344244610465));
#21444=CARTESIAN_POINT('Ctrl Pts',(146.087251184375,74.3078674490983,-57.8334294837149));
#21445=CARTESIAN_POINT('Ctrl Pts',(145.854718046044,74.9016133224768,-57.9320930104149));
#21446=CARTESIAN_POINT('Ctrl Pts',(145.206033961624,76.5579514298781,-58.207328875473));
#21447=CARTESIAN_POINT('Ctrl Pts',(144.535923549658,78.2056781948319,-58.4798984641246));
#21448=CARTESIAN_POINT('Ctrl Pts',(143.844362799228,79.8448249563277,-58.7497069691199));
#21449=CARTESIAN_POINT('Ctrl Pts',(143.1513853196,81.4873296687725,-59.020068202978));
#21450=CARTESIAN_POINT('Ctrl Pts',(142.436869320226,83.1212194287967,-59.2876571684577));
#21451=CARTESIAN_POINT('Ctrl Pts',(141.700748012094,84.7465005374518,-59.5523615928747));
#21452=CARTESIAN_POINT('Ctrl Pts',(140.964375086706,86.372337191461,-59.8171564972169));
#21453=CARTESIAN_POINT('Ctrl Pts',(140.206381845747,87.9895595256459,-60.0790650220006));
#21454=CARTESIAN_POINT('Ctrl Pts',(139.426662132564,89.5981451905916,-60.3379558580429));
#21455=CARTESIAN_POINT('Ctrl Pts',(138.647119944871,91.2063646150111,-60.5967877501831));
#21456=CARTESIAN_POINT('Ctrl Pts',(137.845860923211,92.8059514987935,-60.8526034576932));
#21457=CARTESIAN_POINT('Ctrl Pts',(137.022743375541,94.3968517670101,-61.1052508746052));
#21458=CARTESIAN_POINT('Ctrl Pts',(136.382274663422,95.6347330985131,-61.301836120768));
#21459=CARTESIAN_POINT('Ctrl Pts',(135.728571144476,96.8673545851268,-61.4965027555554));
#21460=CARTESIAN_POINT('Ctrl Pts',(135.061552680395,98.0946763544619,-61.6891696133877));
#21461=CARTESIAN_POINT('Ctrl Pts',(134.239401643232,99.6074438713001,-61.9266461834137));
#21462=CARTESIAN_POINT('Ctrl Pts',(133.397005184789,101.112182410997,-62.1610953092384));
#21463=CARTESIAN_POINT('Ctrl Pts',(132.534149953513,102.608830985837,-62.3923631872123));
#21464=CARTESIAN_POINT('Ctrl Pts',(132.322774384846,102.975468322129,-62.4490173946031));
#21465=CARTESIAN_POINT('Ctrl Pts',(132.110170926118,103.34161999574,-62.5054805761156));
#21466=CARTESIAN_POINT('Ctrl Pts',(131.896336194158,103.707284769956,-62.5617502437278));
#21467=CARTESIAN_POINT('Ctrl Pts',(131.150525617363,104.982646605105,-62.7580070111533));
#21468=CARTESIAN_POINT('Ctrl Pts',(130.391368173285,106.249286509145,-62.9514793059366));
#21469=CARTESIAN_POINT('Ctrl Pts',(129.619361911524,107.506510787503,-63.141982854025));
#21470=CARTESIAN_POINT('Ctrl Pts',(129.266469660511,108.081201340666,-63.2290640465498));
#21471=CARTESIAN_POINT('Ctrl Pts',(128.910893216072,108.653924930634,-63.3155250005697));
#21472=CARTESIAN_POINT('Ctrl Pts',(128.552682965157,109.224617543254,-63.4013485459176));
#21473=CARTESIAN_POINT('Ctrl Pts',(127.593775576704,110.752327488401,-63.6310930368334));
#21474=CARTESIAN_POINT('Ctrl Pts',(126.615676477573,112.266004480819,-63.8563473482364));
#21475=CARTESIAN_POINT('Ctrl Pts',(125.618464049675,113.765729384398,-64.0769716167984));
#21476=CARTESIAN_POINT('Ctrl Pts',(124.614206339913,115.276049808418,-64.2991545905214));
#21477=CARTESIAN_POINT('Ctrl Pts',(123.590563995459,116.77222047651,-64.5166420286909));
#21478=CARTESIAN_POINT('Ctrl Pts',(122.547579997488,118.254296304307,-64.7292655492744));
#21479=CARTESIAN_POINT('Ctrl Pts',(122.15972197473,118.805440906012,-64.8083345843179));
#21480=CARTESIAN_POINT('Ctrl Pts',(121.769188853402,119.354636048327,-64.8867307245452));
#21481=CARTESIAN_POINT('Ctrl Pts',(121.375981673587,119.901883520301,-64.9644443511221));
#21482=CARTESIAN_POINT('Ctrl Pts',(120.35986499798,121.31606746836,-65.1652700632155));
#21483=CARTESIAN_POINT('Ctrl Pts',(119.32592306836,122.717230533083,-65.3615257399208));
#21484=CARTESIAN_POINT('Ctrl Pts',(118.274111846381,124.105401649993,-65.553052721444));
#21485=CARTESIAN_POINT('Ctrl Pts',(117.217260755787,125.500224340776,-65.7454974254661));
#21486=CARTESIAN_POINT('Ctrl Pts',(116.142368392054,126.881930373277,-65.9331681660453));
#21487=CARTESIAN_POINT('Ctrl Pts',(115.049363967163,128.250516040694,-66.1158723525937));
#21488=CARTESIAN_POINT('Ctrl Pts',(113.954288243496,129.621695247307,-66.2989227728345));
#21489=CARTESIAN_POINT('Ctrl Pts',(112.841031394603,130.97970435778,-66.4769879351814));
#21490=CARTESIAN_POINT('Ctrl Pts',(111.709501198964,132.324505533451,-66.6498402760476));
#21491=CARTESIAN_POINT('Ctrl Pts',(110.575125429341,133.672688617315,-66.8231273062629));
#21492=CARTESIAN_POINT('Ctrl Pts',(109.422383925239,135.007597262524,-66.9911753997619));
#21493=CARTESIAN_POINT('Ctrl Pts',(108.251168041227,136.329158679192,-67.1537191905785));
#21494=CARTESIAN_POINT('Ctrl Pts',(107.205533034561,137.509018771246,-67.2988346044949));
#21495=CARTESIAN_POINT('Ctrl Pts',(106.145172602991,138.678239943829,-67.4395623725332));
#21496=CARTESIAN_POINT('Ctrl Pts',(105.070002502002,139.836747253322,-67.575688188434));
#21497=CARTESIAN_POINT('Ctrl Pts',(104.335872795981,140.62777988133,-67.6686353463928));
#21498=CARTESIAN_POINT('Ctrl Pts',(103.594385160809,141.414284085743,-67.759495179416));
#21499=CARTESIAN_POINT('Ctrl Pts',(102.846253577245,142.195425520933,-67.8481017411357));
#21500=CARTESIAN_POINT('Ctrl Pts',(102.098121993682,142.976566956123,-67.9367083028554));
#21501=CARTESIAN_POINT('Ctrl Pts',(101.343346621331,143.752345521681,-68.0230615341653));
#21502=CARTESIAN_POINT('Ctrl Pts',(100.58268168766,144.521972689812,-68.1070104348258));
#21503=CARTESIAN_POINT('Ctrl Pts',(99.325773062813,145.793690344617,-68.2457260408908));
#21504=CARTESIAN_POINT('Ctrl Pts',(98.0538833836472,147.047528667054,-68.3777624601209));
#21505=CARTESIAN_POINT('Ctrl Pts',(96.7671060577393,148.283619243825,-68.5028706402217));
#21506=CARTESIAN_POINT('Ctrl Pts',(96.4964012088721,148.543660904517,-68.5291901830861));
#21507=CARTESIAN_POINT('Ctrl Pts',(96.2250374009896,148.802917009055,-68.5552029557569));
#21508=CARTESIAN_POINT('Ctrl Pts',(95.9530153961869,149.061388643233,-68.5809064063632));
#21509=CARTESIAN_POINT('Ctrl Pts',(94.6909245240803,150.260610340133,-68.7001617968061));
#21510=CARTESIAN_POINT('Ctrl Pts',(93.4146742779891,151.4429502265,-68.8127591153259));
#21511=CARTESIAN_POINT('Ctrl Pts',(92.1243034092432,152.608485238147,-68.9184302559128));
#21512=CARTESIAN_POINT('Ctrl Pts',(90.8270487660792,153.780238059178,-69.0246651230313));
#21513=CARTESIAN_POINT('Ctrl Pts',(89.5155220275952,154.935006065013,-69.1238998529433));
#21514=CARTESIAN_POINT('Ctrl Pts',(88.189753472043,156.072844050722,-69.2158157195382));
#21515=CARTESIAN_POINT('Ctrl Pts',(87.5636550889273,156.610191629314,-69.2592232775292));
#21516=CARTESIAN_POINT('Ctrl Pts',(86.9343803601109,157.143763101884,-69.300997880872));
#21517=CARTESIAN_POINT('Ctrl Pts',(86.3019321777129,157.673562624529,-69.3411022734024));
#21518=CARTESIAN_POINT('Ctrl Pts',(85.0908680290335,158.688066619829,-69.41789748501));
#21519=CARTESIAN_POINT('Ctrl Pts',(83.8682332813244,159.688756437948,-69.4885573011914));
#21520=CARTESIAN_POINT('Ctrl Pts',(82.6339523845695,160.675622844142,-69.5528173901377));
#21521=CARTESIAN_POINT('Ctrl Pts',(81.4013292413063,161.661163797406,-69.6169911718366));
#21522=CARTESIAN_POINT('Ctrl Pts',(80.1570908588353,162.63291819202,-69.6747824784201));
#21523=CARTESIAN_POINT('Ctrl Pts',(78.9011663895971,163.590858124471,-69.7258797875447));
#21524=CARTESIAN_POINT('Ctrl Pts',(77.650965694506,164.54443232319,-69.7767442248173));
#21525=CARTESIAN_POINT('Ctrl Pts',(76.3891848535843,165.484317383387,-69.8209755698939));
#21526=CARTESIAN_POINT('Ctrl Pts',(75.1157634657088,166.410471429902,-69.858217964424));
#21527=CARTESIAN_POINT('Ctrl Pts',(73.8478440584874,167.332623908912,-69.8952994484054));
#21528=CARTESIAN_POINT('Ctrl Pts',(72.5683841627989,168.241163423421,-69.9254522553877));
#21529=CARTESIAN_POINT('Ctrl Pts',(71.2773384017722,169.136039253356,-69.9482765461247));
#21530=CARTESIAN_POINT('Ctrl Pts',(69.9972799515188,170.023299335543,-69.9709065931075));
#21531=CARTESIAN_POINT('Ctrl Pts',(68.7058317241478,170.897126922303,-69.9863322828695));
#21532=CARTESIAN_POINT('Ctrl Pts',(67.4029678704178,171.757468812413,-69.9941163663231));
#21533=CARTESIAN_POINT('Ctrl Pts',(66.7497755452623,172.18880223073,-69.9980189257162));
#21534=CARTESIAN_POINT('Ctrl Pts',(66.0937141832166,172.616745954954,-70.));
#21535=CARTESIAN_POINT('Ctrl Pts',(65.4347826086956,173.041293409847,-70.));
#21536=CARTESIAN_POINT('Origin',(3.92135447228745,250.,28.0096748020596));
#21537=CARTESIAN_POINT('Origin',(-126.751426934183,250.,46.3038641989655));
#21538=CARTESIAN_POINT('Origin',(-108.033967922038,250.,180.));
#21539=CARTESIAN_POINT('Origin',(-115.000000000001,250.,45.1798442476468));
#21540=CARTESIAN_POINT('Ctrl Pts',(-113.709994059637,250.,70.1465397573418));
#21541=CARTESIAN_POINT('Ctrl Pts',(-113.709994059638,275.,70.1465397573418));
#21542=CARTESIAN_POINT('Ctrl Pts',(-115.000000000001,275.,45.1798442476468));
#21543=CARTESIAN_POINT('Ctrl Pts',(-111.818880948996,250.000000000097,70.048827701468));
#21544=CARTESIAN_POINT('Ctrl Pts',(-111.587915676106,274.988026907036,70.0368939406218));
#21545=CARTESIAN_POINT('Ctrl Pts',(-112.446996903957,275.,45.0599248877022));
#21546=CARTESIAN_POINT('Ctrl Pts',(-109.926868419216,249.967686392701,70.0000000000001));
#21547=CARTESIAN_POINT('Ctrl Pts',(-109.462400534861,274.952458214506,69.9880155941608));
#21548=CARTESIAN_POINT('Ctrl Pts',(-109.892780719043,274.964455041348,44.9999999999839));
#21549=CARTESIAN_POINT('Ctrl Pts',(-108.033967922038,249.902929948988,70.0000000000001));
#21550=CARTESIAN_POINT('Ctrl Pts',(-107.337364714242,274.893222943887,70.));
#21551=CARTESIAN_POINT('Ctrl Pts',(-107.337364714242,274.893222943887,45.0000000000001));
#21552=CARTESIAN_POINT('Origin',(-108.033967922038,249.902929948988,45.0000000000001));
#21553=CARTESIAN_POINT('Origin',(-115.,0.,45.0000000000001));
#21554=CARTESIAN_POINT('Ctrl Pts',(65.4347826086958,173.041293409847,70.));
#21555=CARTESIAN_POINT('Ctrl Pts',(66.7484164009789,172.194923460766,70.));
#21556=CARTESIAN_POINT('Ctrl Pts',(68.0506414965792,171.335055332599,69.9921294361605));
#21557=CARTESIAN_POINT('Ctrl Pts',(69.341472894354,170.461741779368,69.9768486490774));
#21558=CARTESIAN_POINT('Ctrl Pts',(70.6413050269686,169.582338768026,69.9614613118182));
#21559=CARTESIAN_POINT('Ctrl Pts',(71.9295842856713,168.689302588284,69.938560099864));
#21560=CARTESIAN_POINT('Ctrl Pts',(73.2063469470379,167.78268628942,69.908566552343));
#21561=CARTESIAN_POINT('Ctrl Pts',(74.4928427896132,166.86915855667,69.8783443541557));
#21562=CARTESIAN_POINT('Ctrl Pts',(75.7676460752356,165.941843244657,69.8409213017712));
#21563=CARTESIAN_POINT('Ctrl Pts',(77.0308108162073,165.000787772658,69.7966789898779));
#21564=CARTESIAN_POINT('Ctrl Pts',(78.2972938165541,164.057260203362,69.752320456037));
#21565=CARTESIAN_POINT('Ctrl Pts',(79.5520773777388,163.099920519143,69.7011067518214));
#21566=CARTESIAN_POINT('Ctrl Pts',(80.7952280690075,162.128804309335,69.6433728837564));
#21567=CARTESIAN_POINT('Ctrl Pts',(82.0410026914299,161.155638354395,69.5855171562128));
#21568=CARTESIAN_POINT('Ctrl Pts',(83.2750956333978,160.168637936665,69.5211136521883));
#21569=CARTESIAN_POINT('Ctrl Pts',(84.4975809196787,159.167822048422,69.4504504842125));
#21570=CARTESIAN_POINT('Ctrl Pts',(85.1018573206763,158.673117179746,69.4155215690699));
#21571=CARTESIAN_POINT('Ctrl Pts',(85.7032976515598,158.175036435941,69.3790624569837));
#21572=CARTESIAN_POINT('Ctrl Pts',(86.301911080951,157.673580297207,69.3411036111759));
#21573=CARTESIAN_POINT('Ctrl Pts',(87.6416535312517,156.551283263696,69.2561488230001));
#21574=CARTESIAN_POINT('Ctrl Pts',(88.9671556757048,155.412061378825,69.1637022638884));
#21575=CARTESIAN_POINT('Ctrl Pts',(90.2783893218386,154.255869801442,69.0641054510097));
#21576=CARTESIAN_POINT('Ctrl Pts',(91.5830443271285,153.105478997367,68.965008329138));
#21577=CARTESIAN_POINT('Ctrl Pts',(92.8735740567254,151.938288542509,68.8588323958833));
#21578=CARTESIAN_POINT('Ctrl Pts',(94.1499446972401,150.75423258277,68.7458677221814));
#21579=CARTESIAN_POINT('Ctrl Pts',(94.7541325596118,150.193743163368,68.6923943167606));
#21580=CARTESIAN_POINT('Ctrl Pts',(95.3551476204497,149.629474299346,68.6373990733229));
#21581=CARTESIAN_POINT('Ctrl Pts',(95.9529854143453,149.061417131568,68.580909239356));
#21582=CARTESIAN_POINT('Ctrl Pts',(97.2460239280367,147.832789896195,68.4587297256198));
#21583=CARTESIAN_POINT('Ctrl Pts',(98.5241919067625,146.586439424219,68.3295643380909));
#21584=CARTESIAN_POINT('Ctrl Pts',(99.7874001697264,145.322239383386,68.1936707789836));
#21585=CARTESIAN_POINT('Ctrl Pts',(100.053145131183,145.056285778606,68.1650824379429));
#21586=CARTESIAN_POINT('Ctrl Pts',(100.318227953058,144.789542120827,68.1361961843661));
#21587=CARTESIAN_POINT('Ctrl Pts',(100.582647686213,144.52200709186,68.1070141873093));
#21588=CARTESIAN_POINT('Ctrl Pts',(101.343311973865,143.752380938002,68.0230654489202));
#21589=CARTESIAN_POINT('Ctrl Pts',(102.098086743775,142.97660336885,67.9367123807548));
#21590=CARTESIAN_POINT('Ctrl Pts',(102.84621774979,142.195462929158,67.8481059844437));
#21591=CARTESIAN_POINT('Ctrl Pts',(103.594348755805,141.414322489467,67.7594995881325));
#21592=CARTESIAN_POINT('Ctrl Pts',(104.335835838317,140.627819279647,67.6686399227833));
#21593=CARTESIAN_POINT('Ctrl Pts',(105.069964998763,139.836787663453,67.5756929366653));
#21594=CARTESIAN_POINT('Ctrl Pts',(106.274691395938,138.538682751708,67.4231643439496));
#21595=CARTESIAN_POINT('Ctrl Pts',(107.460824156216,137.227126993047,67.2648585766541));
#21596=CARTESIAN_POINT('Ctrl Pts',(108.628481350401,135.902223981139,67.1010750526694));
#21597=CARTESIAN_POINT('Ctrl Pts',(109.79344823223,134.580373580015,66.9376688901572));
#21598=CARTESIAN_POINT('Ctrl Pts',(110.940024958247,133.245237386367,66.7688100565757));
#21599=CARTESIAN_POINT('Ctrl Pts',(112.068318136567,131.896884093635,66.5947584549084));
#21600=CARTESIAN_POINT('Ctrl Pts',(113.194372744947,130.551205977185,66.4210521772144));
#21601=CARTESIAN_POINT('Ctrl Pts',(114.302216644142,129.192363144643,66.2421735841328));
#21602=CARTESIAN_POINT('Ctrl Pts',(115.391939711775,127.820389677704,66.0583456279631));
#21603=CARTESIAN_POINT('Ctrl Pts',(116.477450936578,126.453718967751,65.8752281775008));
#21604=CARTESIAN_POINT('Ctrl Pts',(117.544981473468,125.07401887109,65.6871994023175));
#21605=CARTESIAN_POINT('Ctrl Pts',(118.594598963408,123.681289636736,65.4944466132403));
#21606=CARTESIAN_POINT('Ctrl Pts',(119.53611361456,122.432001213286,65.3215459358927));
#21607=CARTESIAN_POINT('Ctrl Pts',(120.463214920894,121.172228781595,65.1448437142406));
#21608=CARTESIAN_POINT('Ctrl Pts',(121.375933771032,119.901950188821,64.9644538185964));
#21609=CARTESIAN_POINT('Ctrl Pts',(122.433881518173,118.429548939232,64.7553608611377));
#21610=CARTESIAN_POINT('Ctrl Pts',(123.472473810833,116.943050420668,64.5413290851279));
#21611=CARTESIAN_POINT('Ctrl Pts',(124.491680181692,115.442410467452,64.3225371850261));
#21612=CARTESIAN_POINT('Ctrl Pts',(125.503830307995,113.952159855199,64.1052600411091));
#21613=CARTESIAN_POINT('Ctrl Pts',(126.496862295989,112.447962781688,63.8832882990187));
#21614=CARTESIAN_POINT('Ctrl Pts',(127.470711714623,110.929748092818,63.6567711904821));
#21615=CARTESIAN_POINT('Ctrl Pts',(127.83402354599,110.363351123772,63.5722649578308));
#21616=CARTESIAN_POINT('Ctrl Pts',(128.194665186969,109.795002921474,63.4871258563392));
#21617=CARTESIAN_POINT('Ctrl Pts',(128.552631924842,109.224698859508,63.4013607746513));
#21618=CARTESIAN_POINT('Ctrl Pts',(129.336349318664,107.976099015325,63.2135902943521));
#21619=CARTESIAN_POINT('Ctrl Pts',(130.107456590396,106.717775301267,63.0227682840443));
#21620=CARTESIAN_POINT('Ctrl Pts',(130.865437062443,105.450406778866,62.8290762477486));
#21621=CARTESIAN_POINT('Ctrl Pts',(131.211808809534,104.871261714447,62.740565459564));
#21622=CARTESIAN_POINT('Ctrl Pts',(131.555439991089,104.290228375938,62.6514554438038));
#21623=CARTESIAN_POINT('Ctrl Pts',(131.896284148027,103.707373770585,62.5617639394275));
#21624=CARTESIAN_POINT('Ctrl Pts',(132.769178417835,102.214696150074,62.332066000863));
#21625=CARTESIAN_POINT('Ctrl Pts',(133.621557467831,100.71390800504,62.0991453921073));
#21626=CARTESIAN_POINT('Ctrl Pts',(134.453641402604,99.2050793476407,61.8631619225103));
#21627=CARTESIAN_POINT('Ctrl Pts',(134.657478130989,98.8354595480436,61.8053527323728));
#21628=CARTESIAN_POINT('Ctrl Pts',(134.860096801376,98.4653570557965,61.7473596212806));
#21629=CARTESIAN_POINT('Ctrl Pts',(135.061500391748,98.0947725661239,61.6891847168399));
#21630=CARTESIAN_POINT('Ctrl Pts',(135.918476370644,96.517928751097,61.4416494291702));
#21631=CARTESIAN_POINT('Ctrl Pts',(136.753474751504,94.9323379967978,61.1908139275639));
#21632=CARTESIAN_POINT('Ctrl Pts',(137.566662089513,93.3380809660457,60.9368477650047));
#21633=CARTESIAN_POINT('Ctrl Pts',(138.380360599555,91.742821780475,60.6827219585432));
#21634=CARTESIAN_POINT('Ctrl Pts',(139.172220905911,90.1388852411411,60.4254614269076));
#21635=CARTESIAN_POINT('Ctrl Pts',(139.942377264237,88.5263181774426,60.1652136179345));
#21636=CARTESIAN_POINT('Ctrl Pts',(140.712233804798,86.914378877507,59.9050671220462));
#21637=CARTESIAN_POINT('Ctrl Pts',(141.460403539085,85.2938155678344,59.6419355415775));
#21638=CARTESIAN_POINT('Ctrl Pts',(142.186984131365,83.6646439519117,59.3759457057129));
#21639=CARTESIAN_POINT('Ctrl Pts',(142.912502334737,82.0378544720814,59.110344793877));
#21640=CARTESIAN_POINT('Ctrl Pts',(143.616494706017,80.4024816159027,58.8418938423145));
#21641=CARTESIAN_POINT('Ctrl Pts',(144.299018648534,78.758513255544,58.5707007575231));
#21642=CARTESIAN_POINT('Ctrl Pts',(144.830588555321,77.4781418961833,58.3594875328673));
#21643=CARTESIAN_POINT('Ctrl Pts',(145.349135473784,76.1925561244661,58.1466106118989));
#21644=CARTESIAN_POINT('Ctrl Pts',(145.85466847965,74.9017398842795,57.9321140413525));
#21645=CARTESIAN_POINT('Ctrl Pts',(146.516232013982,73.2125189152811,57.6514140521017));
#21646=CARTESIAN_POINT('Ctrl Pts',(147.155497232843,71.5143630118513,57.3679509334573));
#21647=CARTESIAN_POINT('Ctrl Pts',(147.772428977714,69.807239987182,57.0818271781275));
#21648=CARTESIAN_POINT('Ctrl Pts',(148.386770152708,68.1072853754217,56.7969048905253));
#21649=CARTESIAN_POINT('Ctrl Pts',(148.978965174465,66.398438517869,56.5093441244595));
#21650=CARTESIAN_POINT('Ctrl Pts',(149.548932147378,64.6806505934696,56.2192337314343));
#21651=CARTESIAN_POINT('Ctrl Pts',(149.749721271601,64.0755047704084,56.1170330522513));
#21652=CARTESIAN_POINT('Ctrl Pts',(149.947751397002,63.4692492021539,56.0145158552573));
#21653=CARTESIAN_POINT('Ctrl Pts',(150.1430174875,62.8618813470188,55.911685707308));
#21654=CARTESIAN_POINT('Ctrl Pts',(150.692594437047,61.1524428458079,55.6222699726696));
#21655=CARTESIAN_POINT('Ctrl Pts',(151.220279633146,59.4341937070619,55.3303766976904));
#21656=CARTESIAN_POINT('Ctrl Pts',(151.725928605588,57.7070595737709,55.0360816657165));
#21657=CARTESIAN_POINT('Ctrl Pts',(151.821168551398,57.3817505743925,54.9806506366331));
#21658=CARTESIAN_POINT('Ctrl Pts',(151.915626585807,57.0561263418963,54.9251343787327));
#21659=CARTESIAN_POINT('Ctrl Pts',(152.009301540551,56.7301863473222,54.8695333676534));
#21660=CARTESIAN_POINT('Ctrl Pts',(152.264011555342,55.8439283174525,54.7183495811949));
#21661=CARTESIAN_POINT('Ctrl Pts',(152.513007414861,54.9550568431241,54.5664917271939));
#21662=CARTESIAN_POINT('Ctrl Pts',(152.755993471224,54.0645582860792,54.4141395690049));
#21663=CARTESIAN_POINT('Ctrl Pts',(152.998916131407,53.1742920642056,54.261827160195));
#21664=CARTESIAN_POINT('Ctrl Pts',(153.23583207891,52.2823997307104,54.1090207462948));
#21665=CARTESIAN_POINT('Ctrl Pts',(153.466495510062,51.3898821467467,53.9559047087908));
#21666=CARTESIAN_POINT('Ctrl Pts',(153.540466822289,51.1036612380325,53.9068020219861));
#21667=CARTESIAN_POINT('Ctrl Pts',(153.613795499395,50.8173761372881,53.8576675269881));
#21668=CARTESIAN_POINT('Ctrl Pts',(153.686474525376,50.5310601534892,53.8085073975534));
#21669=CARTESIAN_POINT('Ctrl Pts',(154.128896893156,48.7881557353863,53.5092526872527));
#21670=CARTESIAN_POINT('Ctrl Pts',(154.547717548931,47.0422790819696,53.2087305243606));
#21671=CARTESIAN_POINT('Ctrl Pts',(154.943135950867,45.2934692031631,52.9070433704346));
#21672=CARTESIAN_POINT('Ctrl Pts',(155.339941312342,43.538525243262,52.6042980263133));
#21673=CARTESIAN_POINT('Ctrl Pts',(155.713180124024,41.7806271784725,52.3003793805853));
#21674=CARTESIAN_POINT('Ctrl Pts',(156.063008646656,40.0197906561065,51.9953791652994));
#21675=CARTESIAN_POINT('Ctrl Pts',(156.413237885962,38.2569371553939,51.6900295826407));
#21676=CARTESIAN_POINT('Ctrl Pts',(156.740003301058,36.4911381757485,51.3835958217297));
#21677=CARTESIAN_POINT('Ctrl Pts',(157.043414214413,34.7223897964007,51.0761600223204));
#21678=CARTESIAN_POINT('Ctrl Pts',(157.34707364086,32.9521926981324,50.7684724131767));
#21679=CARTESIAN_POINT('Ctrl Pts',(157.627340398481,31.1790410720362,50.4597809926956));
#21680=CARTESIAN_POINT('Ctrl Pts',(157.884274805064,29.402915704594,50.1501601383299));
#21681=CARTESIAN_POINT('Ctrl Pts',(158.073892018425,28.0921378012609,49.9216604041597));
#21682=CARTESIAN_POINT('Ctrl Pts',(158.250800442238,26.7797399355903,49.6926542872569));
#21683=CARTESIAN_POINT('Ctrl Pts',(158.415006661951,25.4657104901417,49.463169537153));
#21684=CARTESIAN_POINT('Ctrl Pts',(158.639828857533,23.6666130777445,49.148971539896));
#21685=CARTESIAN_POINT('Ctrl Pts',(158.840838866152,21.8644778479518,48.8338827881402));
#21686=CARTESIAN_POINT('Ctrl Pts',(159.01800742211,20.0592853583608,48.5179779687453));
#21687=CARTESIAN_POINT('Ctrl Pts',(159.194796131046,18.2579631774022,48.2027504450717));
#21688=CARTESIAN_POINT('Ctrl Pts',(159.347845539902,16.4535965187214,47.8867102164476));
#21689=CARTESIAN_POINT('Ctrl Pts',(159.477074839366,14.6461632758025,47.5699289235262));
#21690=CARTESIAN_POINT('Ctrl Pts',(159.521446942324,14.0255639668495,47.4611590686801));
#21691=CARTESIAN_POINT('Ctrl Pts',(159.563010305271,13.4046031180388,47.3523018323499));
#21692=CARTESIAN_POINT('Ctrl Pts',(159.60176023808,12.7832798613223,47.2433600880803));
#21693=CARTESIAN_POINT('Ctrl Pts',(159.713375040897,10.9936284282252,46.929565703839));
#21694=CARTESIAN_POINT('Ctrl Pts',(159.801651714041,9.20096871886184,46.6150701364191));
#21695=CARTESIAN_POINT('Ctrl Pts',(159.866444427471,7.40526826756703,46.2999402754388));
#21696=CARTESIAN_POINT('Ctrl Pts',(159.878482139281,7.07164858436365,46.2413929134261));
#21697=CARTESIAN_POINT('Ctrl Pts',(159.889709106815,6.73792395991809,46.182823660671));
#21698=CARTESIAN_POINT('Ctrl Pts',(159.900124197961,6.40409421188559,46.1242329519068));
#21699=CARTESIAN_POINT('Ctrl Pts',(159.933361240614,5.33876377760979,45.937256010576));
#21700=CARTESIAN_POINT('Ctrl Pts',(159.958330637681,4.27236229656624,45.7500604690855));
#21701=CARTESIAN_POINT('Ctrl Pts',(159.974991372694,3.20488185158275,45.5626601505172));
#21702=CARTESIAN_POINT('Ctrl Pts',(159.9833217402,2.67114162909094,45.468959991233));
#21703=CARTESIAN_POINT('Ctrl Pts',(159.989574840371,2.13713166462133,45.3752086357616));
#21704=CARTESIAN_POINT('Ctrl Pts',(159.993744929012,1.60285087169006,45.2814078106192));
#21705=CARTESIAN_POINT('Ctrl Pts',(159.995829973332,1.33571047522442,45.234507398048));
#21706=CARTESIAN_POINT('Ctrl Pts',(159.997394258275,1.0685023715434,45.1875946178656));
#21707=CARTESIAN_POINT('Ctrl Pts',(159.998437026632,0.80122642143114,45.1406696856376));
#21708=CARTESIAN_POINT('Ctrl Pts',(159.999479794988,0.533950471318885,45.0937447534096));
#21709=CARTESIAN_POINT('Ctrl Pts',(160.,0.265592952447147,45.0466296899014));
#21710=CARTESIAN_POINT('Ctrl Pts',(160.,3.36777869765522E-14,45.));
#21711=CARTESIAN_POINT('Ctrl Pts',(65.4243934602224,173.04853626372,69.9999998857046));
#21712=CARTESIAN_POINT('Ctrl Pts',(56.5824686834193,149.661031129524,69.9968988863329));
#21713=CARTESIAN_POINT('Ctrl Pts',(56.5812975378023,149.661473897575,94.9999996631391));
#21714=CARTESIAN_POINT('Ctrl Pts',(69.2022850192574,170.614767694469,70.0001026648394));
#21715=CARTESIAN_POINT('Ctrl Pts',(60.0163277184471,148.362786737093,70.9204251271389));
#21716=CARTESIAN_POINT('Ctrl Pts',(60.4989568014547,148.180355676071,95.0002407754135));
#21717=CARTESIAN_POINT('Ctrl Pts',(72.867487114648,168.080831911,69.9354862567983));
#21718=CARTESIAN_POINT('Ctrl Pts',(63.529881785745,146.900483832406,71.6775178358105));
#21719=CARTESIAN_POINT('Ctrl Pts',(64.3290816927398,146.556845898137,94.871040775192));
#21720=CARTESIAN_POINT('Ctrl Pts',(79.9886618889852,162.815535315842,69.6989874325338));
#21721=CARTESIAN_POINT('Ctrl Pts',(70.5057678662081,143.683924978654,72.8662379282042));
#21722=CARTESIAN_POINT('Ctrl Pts',(71.8188031734396,143.035546027714,94.3981030531638));
#21723=CARTESIAN_POINT('Ctrl Pts',(83.4448180787027,160.084321402834,69.5270912439842));
#21724=CARTESIAN_POINT('Ctrl Pts',(73.9797811265126,141.934709130391,73.3100631633681));
#21725=CARTESIAN_POINT('Ctrl Pts',(75.4785580886896,141.137975699511,94.0543379212644));
#21726=CARTESIAN_POINT('Ctrl Pts',(90.1649508888079,154.418488187676,69.0903834186758));
#21727=CARTESIAN_POINT('Ctrl Pts',(80.8468574617034,138.140544889064,73.9275707376667));
#21728=CARTESIAN_POINT('Ctrl Pts',(82.6353585459653,137.070560054605,93.180971287852));
#21729=CARTESIAN_POINT('Ctrl Pts',(93.4288956283072,151.483876143982,68.8255110458721));
#21730=CARTESIAN_POINT('Ctrl Pts',(84.250544779031,136.099279342344,74.1094550058665));
#21731=CARTESIAN_POINT('Ctrl Pts',(86.1323917334847,134.9007094904,92.6512484049633));
#21732=CARTESIAN_POINT('Ctrl Pts',(98.1868895196157,146.923477254202,68.3655653196807));
#21733=CARTESIAN_POINT('Ctrl Pts',(89.3086164492795,132.791122112537,74.2087035772314));
#21734=CARTESIAN_POINT('Ctrl Pts',(91.2562278085006,131.440284798265,91.7313856490923));
#21735=CARTESIAN_POINT('Ctrl Pts',(99.7498644441552,145.376897980895,68.2017775273551));
#21736=CARTESIAN_POINT('Ctrl Pts',(90.9728032557208,131.658236954755,74.2136476432942));
#21737=CARTESIAN_POINT('Ctrl Pts',(92.9438609765903,130.252495749627,91.4038190220956));
#21738=CARTESIAN_POINT('Ctrl Pts',(102.830397761921,142.229443429941,67.8540969995271));
#21739=CARTESIAN_POINT('Ctrl Pts',(94.2736611523608,129.316493185164,74.1697160096125));
#21740=CARTESIAN_POINT('Ctrl Pts',(96.2782413450362,127.80756701287,90.7084745843661));
#21741=CARTESIAN_POINT('Ctrl Pts',(104.340526689813,140.636086286616,67.6710267247838));
#21742=CARTESIAN_POINT('Ctrl Pts',(95.9037030178137,128.113362455015,74.1215224810223));
#21743=CARTESIAN_POINT('Ctrl Pts',(97.9169503291095,126.556249426087,90.3423416598691));
#21744=CARTESIAN_POINT('Ctrl Pts',(108.773784815397,135.80766015676,67.0972794963739));
#21745=CARTESIAN_POINT('Ctrl Pts',(100.689275594125,124.436982180208,73.9049733062588));
#21746=CARTESIAN_POINT('Ctrl Pts',(102.73863706313,122.725817074548,89.194868194963));
#21747=CARTESIAN_POINT('Ctrl Pts',(111.604568491427,132.519638863472,66.6816419373888));
#21748=CARTESIAN_POINT('Ctrl Pts',(103.806017905932,121.852642889054,73.6651628390201));
#21749=CARTESIAN_POINT('Ctrl Pts',(105.832302044554,120.066719009531,88.3636043219205));
#21750=CARTESIAN_POINT('Ctrl Pts',(117.032367731531,125.801765879975,65.791893690712));
#21751=CARTESIAN_POINT('Ctrl Pts',(109.828742610535,116.451539928799,73.0190491317221));
#21752=CARTESIAN_POINT('Ctrl Pts',(111.787252032969,114.543020095861,86.5841254176761));
#21753=CARTESIAN_POINT('Ctrl Pts',(119.62934181667,122.371918899055,65.3177549901836));
#21754=CARTESIAN_POINT('Ctrl Pts',(112.74472984579,113.63381946986,72.615217563022));
#21755=CARTESIAN_POINT('Ctrl Pts',(114.648510013565,111.6784057416,85.6358543715796));
#21756=CARTESIAN_POINT('Ctrl Pts',(124.599146009151,115.364277479383,64.3161618719215));
#21757=CARTESIAN_POINT('Ctrl Pts',(118.360419512033,107.768760881291,71.6629242936508));
#21758=CARTESIAN_POINT('Ctrl Pts',(120.142754803448,105.745286540605,83.6326763250999));
#21759=CARTESIAN_POINT('Ctrl Pts',(126.971956044848,111.786495074342,63.7886914051919));
#21760=CARTESIAN_POINT('Ctrl Pts',(121.068699600671,104.720063055232,71.1159985294063));
#21761=CARTESIAN_POINT('Ctrl Pts',(122.775732250521,102.676780126252,82.5777372262751));
#21762=CARTESIAN_POINT('Ctrl Pts',(129.80075461093,107.216308621383,63.0980550220973));
#21763=CARTESIAN_POINT('Ctrl Pts',(124.331930740369,100.74355600257,70.3475688232352));
#21764=CARTESIAN_POINT('Ctrl Pts',(125.924058053992,98.7124951748074,81.1964639412214));
#21765=CARTESIAN_POINT('Ctrl Pts',(130.359642034789,106.297366146314,62.9583586603758));
#21766=CARTESIAN_POINT('Ctrl Pts',(124.974276453257,99.9453785304544,70.1907346207442));
#21767=CARTESIAN_POINT('Ctrl Pts',(126.546567681517,97.9131968052432,80.9170710194551));
#21768=CARTESIAN_POINT('Ctrl Pts',(131.463698410258,104.449503828761,62.6758629251867));
#21769=CARTESIAN_POINT('Ctrl Pts',(126.245180402254,98.3344969993201,69.8692369403547));
#21770=CARTESIAN_POINT('Ctrl Pts',(127.777227456477,96.3016513053162,80.3520788936282));
#21771=CARTESIAN_POINT('Ctrl Pts',(132.009235466058,103.519919452344,62.5329597002741));
#21772=CARTESIAN_POINT('Ctrl Pts',(126.874283999707,97.5211676540206,69.7044590655436));
#21773=CARTESIAN_POINT('Ctrl Pts',(128.38578921301,95.488818477239,80.0662719859412));
#21774=CARTESIAN_POINT('Ctrl Pts',(133.619372483136,100.726336503739,62.1012543515074));
#21775=CARTESIAN_POINT('Ctrl Pts',(128.730630620049,95.0726690744142,69.2014135825394));
#21776=CARTESIAN_POINT('Ctrl Pts',(130.183236617943,93.0399172816863,79.202859577207));
#21777=CARTESIAN_POINT('Ctrl Pts',(134.65924893846,98.8546953904331,61.8090337480645));
#21778=CARTESIAN_POINT('Ctrl Pts',(129.936019779115,93.4178260914866,68.8522667873865));
#21779=CARTESIAN_POINT('Ctrl Pts',(131.345830830391,91.3910083774188,78.6184167040672));
#21780=CARTESIAN_POINT('Ctrl Pts',(139.695933192192,89.4486190475415,60.3271033697907));
#21781=CARTESIAN_POINT('Ctrl Pts',(135.733435509069,85.1282711403168,67.062675590899));
#21782=CARTESIAN_POINT('Ctrl Pts',(136.984252256805,83.0663208160601,75.6545459910273));
#21783=CARTESIAN_POINT('Ctrl Pts',(143.208042277038,81.7712744795915,59.0755984870333));
#21784=CARTESIAN_POINT('Ctrl Pts',(139.892479129903,78.114080631359,65.4234070469369));
#21785=CARTESIAN_POINT('Ctrl Pts',(140.93966573095,76.1514359803153,73.1515201301065));
#21786=CARTESIAN_POINT('Ctrl Pts',(147.752894591533,69.9881927629273,57.1141792462043));
#21787=CARTESIAN_POINT('Ctrl Pts',(145.300074704311,67.1397517789991,62.7372455796463));
#21788=CARTESIAN_POINT('Ctrl Pts',(146.0744422133,65.4065361919382,69.2286486638968));
#21789=CARTESIAN_POINT('Ctrl Pts',(149.146622556606,66.0158544859077,56.4462099795947));
#21790=CARTESIAN_POINT('Ctrl Pts',(146.96016515084,63.4242781036387,61.8087879512217));
#21791=CARTESIAN_POINT('Ctrl Pts',(147.652339743588,61.762547280548,67.8926978272171));
#21792=CARTESIAN_POINT('Ctrl Pts',(151.056362852687,59.9840340597369,55.4238420750756));
#21793=CARTESIAN_POINT('Ctrl Pts',(149.242347721897,57.7367729866036,60.3647058331654));
#21794=CARTESIAN_POINT('Ctrl Pts',(149.817529237813,56.2019959846749,65.8479415997114));
#21795=CARTESIAN_POINT('Ctrl Pts',(151.662764458627,57.9611955519339,55.0796443921211));
#21796=CARTESIAN_POINT('Ctrl Pts',(149.967111817518,55.8263294589246,59.8759432129804));
#21797=CARTESIAN_POINT('Ctrl Pts',(150.50561314431,54.3327017344974,65.1595391420191));
#21798=CARTESIAN_POINT('Ctrl Pts',(152.526890246365,54.9076662578491,54.558287841893));
#21799=CARTESIAN_POINT('Ctrl Pts',(151.001777270768,52.931823465264,59.1304989048559));
#21800=CARTESIAN_POINT('Ctrl Pts',(151.486795724971,51.5048176135938,64.1168149427384));
#21801=CARTESIAN_POINT('Ctrl Pts',(152.807586251953,53.8857006221939,54.3835026198272));
#21802=CARTESIAN_POINT('Ctrl Pts',(151.337862433964,51.9624117285674,58.8800286279954));
#21803=CARTESIAN_POINT('Ctrl Pts',(151.805631706264,50.5573531931399,63.7672407289973));
#21804=CARTESIAN_POINT('Ctrl Pts',(153.352185443809,51.8411536782466,54.0332742455136));
#21805=CARTESIAN_POINT('Ctrl Pts',(151.990284568509,50.020368862806,58.37674383573));
#21806=CARTESIAN_POINT('Ctrl Pts',(152.424429813258,48.6599319331303,63.0667763221949));
#21807=CARTESIAN_POINT('Ctrl Pts',(153.616167010543,50.8183589242819,53.8577952672846));
#21808=CARTESIAN_POINT('Ctrl Pts',(152.30677555528,49.0474544806264,58.1238602884326));
#21809=CARTESIAN_POINT('Ctrl Pts',(152.724480699868,47.7097795578358,62.7158144756579));
#21810=CARTESIAN_POINT('Ctrl Pts',(155.917931196388,41.6079957482047,52.2752944335229));
#21811=CARTESIAN_POINT('Ctrl Pts',(155.053646875237,40.3201454128714,55.8492067253227));
#21812=CARTESIAN_POINT('Ctrl Pts',(155.34153850921,39.1455096493191,59.5507777164435));
#21813=CARTESIAN_POINT('Ctrl Pts',(157.440541638506,33.3840425923826,50.8461835808945));
#21814=CARTESIAN_POINT('Ctrl Pts',(156.901981554525,32.3845089234026,53.7374746717279));
#21815=CARTESIAN_POINT('Ctrl Pts',(157.078106276928,31.4415608589374,56.6925206006809));
#21816=CARTESIAN_POINT('Ctrl Pts',(158.971479743602,20.9484526935852,48.6740963454106));
#21817=CARTESIAN_POINT('Ctrl Pts',(158.754292373091,20.3422965289589,50.5031839548515));
#21818=CARTESIAN_POINT('Ctrl Pts',(158.825192956881,19.7505414459351,52.3482901787236));
#21819=CARTESIAN_POINT('Ctrl Pts',(159.355678878882,16.7866326262453,47.9452859172134));
#21820=CARTESIAN_POINT('Ctrl Pts',(159.219812677019,16.305216939573,49.413970141234));
#21821=CARTESIAN_POINT('Ctrl Pts',(159.263969037536,15.8309336665831,50.8906501976363));
#21822=CARTESIAN_POINT('Ctrl Pts',(159.741443596581,10.5129289469729,46.8452406498883));
#21823=CARTESIAN_POINT('Ctrl Pts',(159.686873998274,10.2140889507991,47.7668807512895));
#21824=CARTESIAN_POINT('Ctrl Pts',(159.704601275429,9.91705122717507,48.690530528023));
#21825=CARTESIAN_POINT('Ctrl Pts',(159.83823957573,8.41652647465408,46.4774188977111));
#21826=CARTESIAN_POINT('Ctrl Pts',(159.804111416692,8.17781928499459,47.2156464811373));
#21827=CARTESIAN_POINT('Ctrl Pts',(159.81518566301,7.9400062771006,47.9548772375799));
#21828=CARTESIAN_POINT('Ctrl Pts',(159.967567107828,4.21229224956273,45.7395342706948));
#21829=CARTESIAN_POINT('Ctrl Pts',(159.960706191155,4.09363866390366,46.1094110069741));
#21830=CARTESIAN_POINT('Ctrl Pts',(159.962941406069,3.97424771515215,46.4790883103916));
#21831=CARTESIAN_POINT('Ctrl Pts',(160.,2.10288127196593,45.3691939815787));
#21832=CARTESIAN_POINT('Ctrl Pts',(160.,2.04346271816514,45.5537959647716));
#21833=CARTESIAN_POINT('Ctrl Pts',(160.,1.98404404900769,45.7383979488414));
#21834=CARTESIAN_POINT('Ctrl Pts',(160.,0.,45.));
#21835=CARTESIAN_POINT('Ctrl Pts',(160.,0.,45.));
#21836=CARTESIAN_POINT('Ctrl Pts',(160.,0.,45.));
#21837=CARTESIAN_POINT('Origin',(65.4347826086958,173.041293409847,95.));
#21838=CARTESIAN_POINT('Origin',(0.,0.,95.));
#21839=CARTESIAN_POINT('Origin',(-14.5652173913043,184.425742352699,95.));
#21840=CARTESIAN_POINT('Ctrl Pts',(-12.5969447708577,159.503344737469,95.));
#21841=CARTESIAN_POINT('Ctrl Pts',(-12.5969447708577,159.503344737469,70.));
#21842=CARTESIAN_POINT('Ctrl Pts',(-14.5652173913043,184.425742352699,70.));
#21843=CARTESIAN_POINT('Ctrl Pts',(-16.5078129272362,159.194479802674,95.));
#21844=CARTESIAN_POINT('Ctrl Pts',(-15.9020915295028,159.242317288254,68.9408032477129));
#21845=CARTESIAN_POINT('Ctrl Pts',(-18.4950032706578,185.155983850241,70.));
#21846=CARTESIAN_POINT('Ctrl Pts',(-20.3710100863973,158.744819305304,94.8172074050833));
#21847=CARTESIAN_POINT('Ctrl Pts',(-18.9874545935604,158.899342445268,67.6784855507893));
#21848=CARTESIAN_POINT('Ctrl Pts',(-22.4253844615201,185.7615463294,69.908603702539));
#21849=CARTESIAN_POINT('Ctrl Pts',(-28.0013011400224,157.577989715187,94.060173223671));
#21850=CARTESIAN_POINT('Ctrl Pts',(-24.7902939337038,158.128801235359,64.714494728495));
#21851=CARTESIAN_POINT('Ctrl Pts',(-30.2945131193187,186.732665530968,69.5300866118382));
#21852=CARTESIAN_POINT('Ctrl Pts',(-31.7684865197378,156.860742338829,93.4863288792126));
#21853=CARTESIAN_POINT('Ctrl Pts',(-27.4990355473887,157.695444326737,62.9860517551233));
#21854=CARTESIAN_POINT('Ctrl Pts',(-34.2333599633667,187.09818816358,69.2431644395594));
#21855=CARTESIAN_POINT('Ctrl Pts',(-37.343678752542,155.592679657295,92.2879046923386));
#21856=CARTESIAN_POINT('Ctrl Pts',(-31.1436763210525,157.073827933375,60.0699145363268));
#21857=CARTESIAN_POINT('Ctrl Pts',(-40.1512716292601,187.470074489004,68.6439523461928));
#21858=CARTESIAN_POINT('Ctrl Pts',(-39.1894418276195,155.137945593457,91.8318643970813));
#21859=CARTESIAN_POINT('Ctrl Pts',(-32.3097589079898,156.867332358696,59.0181216219914));
#21860=CARTESIAN_POINT('Ctrl Pts',(-42.12548806774,187.564605345407,68.4159321985189));
#21861=CARTESIAN_POINT('Ctrl Pts',(-41.9382629795998,154.408810392036,91.0538818796549));
#21862=CARTESIAN_POINT('Ctrl Pts',(-33.9340426077785,156.58074776089,57.3545260494391));
#21863=CARTESIAN_POINT('Ctrl Pts',(-45.0892214588785,187.662475916888,68.0269409398383));
#21864=CARTESIAN_POINT('Ctrl Pts',(-42.8512294298429,154.157926593345,90.7788716538768));
#21865=CARTESIAN_POINT('Ctrl Pts',(-34.4599536442302,156.48817082939,56.7786869254312));
#21866=CARTESIAN_POINT('Ctrl Pts',(-46.0775309162799,187.687777109309,67.889435826931));
#21867=CARTESIAN_POINT('Ctrl Pts',(-44.6703555627358,153.640663657467,90.1955588967012));
#21868=CARTESIAN_POINT('Ctrl Pts',(-35.4696360776896,156.313503350392,55.593044712447));
#21869=CARTESIAN_POINT('Ctrl Pts',(-48.0549067566625,187.723758078197,67.597779448358));
#21870=CARTESIAN_POINT('Ctrl Pts',(-45.5780239544002,153.373821576854,89.8867032935461));
#21871=CARTESIAN_POINT('Ctrl Pts',(-35.9536596323359,156.231426864416,54.9814880064992));
#21872=CARTESIAN_POINT('Ctrl Pts',(-49.0456292326158,187.734439396951,67.4433516467711));
#21873=CARTESIAN_POINT('Ctrl Pts',(-48.2791863488088,152.553799743575,88.9109268015102));
#21874=CARTESIAN_POINT('Ctrl Pts',(-37.3406875913855,156.005960339725,53.0878622163732));
#21875=CARTESIAN_POINT('Ctrl Pts',(-52.006426339423,187.744558869217,66.9554634007591));
#21876=CARTESIAN_POINT('Ctrl Pts',(-50.0455010806815,151.982872872988,88.1971446848615));
#21877=CARTESIAN_POINT('Ctrl Pts',(-38.149975496957,155.888609930498,51.7769554149645));
#21878=CARTESIAN_POINT('Ctrl Pts',(-53.9592290714755,187.722159051229,66.5985723423992));
#21879=CARTESIAN_POINT('Ctrl Pts',(-53.5069789484465,150.799035238803,86.6315720785634));
#21880=CARTESIAN_POINT('Ctrl Pts',(-39.5296138424305,155.747546552728,49.058766931388));
#21881=CARTESIAN_POINT('Ctrl Pts',(-57.8192032663729,187.623216674501,65.8157860393133));
#21882=CARTESIAN_POINT('Ctrl Pts',(-55.2021601069382,150.186106336222,85.7798428475361));
#21883=CARTESIAN_POINT('Ctrl Pts',(-40.0921001658277,155.727065431804,47.6468076105207));
#21884=CARTESIAN_POINT('Ctrl Pts',(-59.7264018532888,187.546662547939,65.3899214237434));
#21885=CARTESIAN_POINT('Ctrl Pts',(-58.5174766142274,148.925652416265,83.9219691980032));
#21886=CARTESIAN_POINT('Ctrl Pts',(-40.9305626227692,155.823418532223,44.7505274971452));
#21887=CARTESIAN_POINT('Ctrl Pts',(-63.4894147199849,187.343877463659,64.4609845990262));
#21888=CARTESIAN_POINT('Ctrl Pts',(-60.1376466369853,148.278097849358,82.9159377469876));
#21889=CARTESIAN_POINT('Ctrl Pts',(-41.1959635800001,155.945547490035,43.261778192548));
#21890=CARTESIAN_POINT('Ctrl Pts',(-65.3452788129041,187.217628898092,63.9579688734417));
#21891=CARTESIAN_POINT('Ctrl Pts',(-62.5068712240698,147.2875546711,81.2731565607321));
#21892=CARTESIAN_POINT('Ctrl Pts',(-41.329056222797,156.271451344433,41.0337957981935));
#21893=CARTESIAN_POINT('Ctrl Pts',(-68.0836879900484,186.994915337258,63.1365782803921));
#21894=CARTESIAN_POINT('Ctrl Pts',(-63.2864190238013,146.954186749042,80.7032055873364));
#21895=CARTESIAN_POINT('Ctrl Pts',(-41.3272321247111,156.407028503944,40.2806421489842));
#21896=CARTESIAN_POINT('Ctrl Pts',(-68.9888958579059,186.915128162852,62.8516027936408));
#21897=CARTESIAN_POINT('Ctrl Pts',(-64.8239857104685,146.282448409019,79.514506063713));
#21898=CARTESIAN_POINT('Ctrl Pts',(-41.2235309507544,156.736842986134,38.7791997063422));
#21899=CARTESIAN_POINT('Ctrl Pts',(-70.7824898970565,186.745236566641,62.257253031884));
#21900=CARTESIAN_POINT('Ctrl Pts',(-65.5807923985165,145.944570108018,78.8965035406746));
#21901=CARTESIAN_POINT('Ctrl Pts',(-41.1193059140031,156.932266944476,38.0321782287653));
#21902=CARTESIAN_POINT('Ctrl Pts',(-71.669484323248,186.655232604801,61.9482517703102));
#21903=CARTESIAN_POINT('Ctrl Pts',(-67.795210035115,144.935989315356,76.9821802471142));
#21904=CARTESIAN_POINT('Ctrl Pts',(-40.6409532007916,157.620893025833,35.8178318542641));
#21905=CARTESIAN_POINT('Ctrl Pts',(-74.2765779917833,186.374146071458,60.9910901236114));
#21906=CARTESIAN_POINT('Ctrl Pts',(-69.2040289876185,144.267167110464,75.62063975569));
#21907=CARTESIAN_POINT('Ctrl Pts',(-40.0961119414972,158.21220805087,34.4207109664872));
#21908=CARTESIAN_POINT('Ctrl Pts',(-75.951232725749,186.171160493749,60.3103198777859));
#21909=CARTESIAN_POINT('Ctrl Pts',(-71.2069497472747,143.283368159876,73.4306585921975));
#21910=CARTESIAN_POINT('Ctrl Pts',(-38.9366264227514,159.316107000538,32.5645400570154));
#21911=CARTESIAN_POINT('Ctrl Pts',(-78.3523532248388,185.852751159626,59.2153292961283));
#21912=CARTESIAN_POINT('Ctrl Pts',(-71.856153509367,142.958707172039,72.6759694271163));
#21913=CARTESIAN_POINT('Ctrl Pts',(-38.4828035089153,159.728767083945,31.9784787713152));
#21914=CARTESIAN_POINT('Ctrl Pts',(-79.1341783828994,185.74431020609,58.8379847135414));
#21915=CARTESIAN_POINT('Ctrl Pts',(-73.1153413914611,142.318816769507,71.1125766454393));
#21916=CARTESIAN_POINT('Ctrl Pts',(-37.4500708169756,160.636987281432,30.9149848733693));
#21917=CARTESIAN_POINT('Ctrl Pts',(-80.6569760131837,185.524679875126,58.0562883227365));
#21918=CARTESIAN_POINT('Ctrl Pts',(-73.7253342774642,142.003581480544,70.3038873576441));
#21919=CARTESIAN_POINT('Ctrl Pts',(-36.8684153167661,161.134321354495,30.4403150385843));
#21920=CARTESIAN_POINT('Ctrl Pts',(-81.3979600403437,185.413487572967,57.6519436787834));
#21921=CARTESIAN_POINT('Ctrl Pts',(-74.9029624412775,141.385955049099,68.6265804660936));
#21922=CARTESIAN_POINT('Ctrl Pts',(-35.5797893182526,162.213781149297,29.6428068354536));
#21923=CARTESIAN_POINT('Ctrl Pts',(-82.8342463013922,185.190488834526,56.8132902330855));
#21924=CARTESIAN_POINT('Ctrl Pts',(-75.4717796014841,141.082897321633,67.755569241579));
#21925=CARTESIAN_POINT('Ctrl Pts',(-34.8681706018876,162.799215603146,29.3240421033952));
#21926=CARTESIAN_POINT('Ctrl Pts',(-83.5310202701526,185.078415158267,56.3777846207694));
#21927=CARTESIAN_POINT('Ctrl Pts',(-76.5472441445947,140.502287692226,65.9735353866643));
#21928=CARTESIAN_POINT('Ctrl Pts',(-33.3511237074772,164.031531871629,28.8970199109168));
#21929=CARTESIAN_POINT('Ctrl Pts',(-84.8533571151316,184.859437149692,55.4867676933523));
#21930=CARTESIAN_POINT('Ctrl Pts',(-77.0558663375507,140.223721881846,65.0600083704848));
#21931=CARTESIAN_POINT('Ctrl Pts',(-32.5426488911884,164.680643187567,28.7922370175357));
#21932=CARTESIAN_POINT('Ctrl Pts',(-85.4813144285751,184.752179051019,55.0300041852196));
#21933=CARTESIAN_POINT('Ctrl Pts',(-78.0120454916522,139.694020894368,63.1847493041814));
#21934=CARTESIAN_POINT('Ctrl Pts',(-30.8564359524551,166.023964520988,28.8369857496512));
#21935=CARTESIAN_POINT('Ctrl Pts',(-86.6658003364468,184.544904934636,54.0923746521136));
#21936=CARTESIAN_POINT('Ctrl Pts',(-78.4596142273092,139.44287884185,62.2230271057913));
#21937=CARTESIAN_POINT('Ctrl Pts',(-29.9787416594907,166.717911624714,28.9922485335044));
#21938=CARTESIAN_POINT('Ctrl Pts',(-87.2223435128929,184.444886160955,53.6115135528724));
#21939=CARTESIAN_POINT('Ctrl Pts',(-79.2896319659011,138.972593654695,60.2472126840058));
#21940=CARTESIAN_POINT('Ctrl Pts',(-28.1983849287021,168.118768320068,29.6042074660882));
#21941=CARTESIAN_POINT('Ctrl Pts',(-88.2574884412621,184.255114157391,52.6236063420261));
#21942=CARTESIAN_POINT('Ctrl Pts',(-79.672099531494,138.753440210982,59.2331358058206));
#21943=CARTESIAN_POINT('Ctrl Pts',(-27.297364480468,168.824245091024,30.0665548817476));
#21944=CARTESIAN_POINT('Ctrl Pts',(-88.7361129449165,184.165357043077,52.1165679028911));
#21945=CARTESIAN_POINT('Ctrl Pts',(-80.1926695171554,138.45279307131,57.668598294985));
#21946=CARTESIAN_POINT('Ctrl Pts',(-25.9814571746451,169.851558160624,31.0113827393965));
#21947=CARTESIAN_POINT('Ctrl Pts',(-89.3891560196825,184.04094680916,51.3342991475022));
#21948=CARTESIAN_POINT('Ctrl Pts',(-80.3577007193496,138.3570444551,57.1383954883763));
#21949=CARTESIAN_POINT('Ctrl Pts',(-25.5454666502937,170.191393781686,31.3722996228226));
#21950=CARTESIAN_POINT('Ctrl Pts',(-89.5964791741451,184.001090877233,51.0691977441812));
#21951=CARTESIAN_POINT('Ctrl Pts',(-80.6659819895472,138.177534950197,56.0739089930283));
#21952=CARTESIAN_POINT('Ctrl Pts',(-24.7029234986323,170.847361230438,32.1739158547286));
#21953=CARTESIAN_POINT('Ctrl Pts',(-89.9842031495538,183.926020864336,50.5369544965211));
#21954=CARTESIAN_POINT('Ctrl Pts',(-80.8095563275921,138.093589167787,55.5388388898697));
#21955=CARTESIAN_POINT('Ctrl Pts',(-24.2962688576142,171.163570352953,32.6151710790885));
#21956=CARTESIAN_POINT('Ctrl Pts',(-90.1650091326306,183.890731563919,50.2694194449313));
#21957=CARTESIAN_POINT('Ctrl Pts',(-81.2084719518345,137.859635628646,53.9250716815212));
#21958=CARTESIAN_POINT('Ctrl Pts',(-23.1286439767822,172.070717278649,34.0596081714576));
#21959=CARTESIAN_POINT('Ctrl Pts',(-90.6678576024157,183.792000424905,49.4625358407677));
#21960=CARTESIAN_POINT('Ctrl Pts',(-81.4320538801261,137.727501177533,52.8378286338531));
#21961=CARTESIAN_POINT('Ctrl Pts',(-22.4329377587908,172.610133759847,35.1736153870478));
#21962=CARTESIAN_POINT('Ctrl Pts',(-90.9503795006326,183.735700011795,48.9189143169189));
#21963=CARTESIAN_POINT('Ctrl Pts',(-81.792814884011,137.513560833443,50.639890051958));
#21964=CARTESIAN_POINT('Ctrl Pts',(-21.2676444399461,173.512933127601,37.6575994990932));
#21965=CARTESIAN_POINT('Ctrl Pts',(-91.4067479064495,183.644151612346,47.8199450259868));
#21966=CARTESIAN_POINT('Ctrl Pts',(-81.9300025600908,137.431751226209,49.5291966979117));
#21967=CARTESIAN_POINT('Ctrl Pts',(-20.803417489149,173.872150439349,39.0242467263608));
#21968=CARTESIAN_POINT('Ctrl Pts',(-91.5806039650975,183.608903080856,47.2645983489531));
#21969=CARTESIAN_POINT('Ctrl Pts',(-82.1146690690122,137.321493904945,47.2833282524998));
#21970=CARTESIAN_POINT('Ctrl Pts',(-20.16786749127,174.363820312557,41.9243194792464));
#21971=CARTESIAN_POINT('Ctrl Pts',(-91.8147222258894,183.561326025264,46.1416641262527));
#21972=CARTESIAN_POINT('Ctrl Pts',(-82.1621621619488,137.293041006723,46.1481485313624));
#21973=CARTESIAN_POINT('Ctrl Pts',(-20.0000000006397,174.493598372083,43.4505009035421));
#21974=CARTESIAN_POINT('Ctrl Pts',(-91.8749999997178,183.54899720507,45.5740742656792));
#21975=CARTESIAN_POINT('Ctrl Pts',(-82.1621621621622,137.293041006595,45.0000000000001));
#21976=CARTESIAN_POINT('Ctrl Pts',(-20.0000000000001,174.493598372593,45.));
#21977=CARTESIAN_POINT('Ctrl Pts',(-91.875,183.548997205106,45.0000000000001));
#21978=CARTESIAN_POINT('Ctrl Pts',(-82.1621621621622,137.293041006595,-45.));
#21979=CARTESIAN_POINT('Ctrl Pts',(-20.,174.493598372593,-45.));
#21980=CARTESIAN_POINT('Ctrl Pts',(-91.875,183.548997205106,-45.));
#21981=CARTESIAN_POINT('Ctrl Pts',(-82.1621621620694,137.29304100665,-46.1481557420891));
#21982=CARTESIAN_POINT('Ctrl Pts',(-20.0000000008088,174.493598372051,-43.4504962324451));
#21983=CARTESIAN_POINT('Ctrl Pts',(-91.8749999998195,183.548997205083,-45.5740778710447));
#21984=CARTESIAN_POINT('Ctrl Pts',(-82.1146674891305,137.321494909959,-47.2836204764629));
#21985=CARTESIAN_POINT('Ctrl Pts',(-20.1678750458358,174.363814523666,-41.9239156869814));
#21986=CARTESIAN_POINT('Ctrl Pts',(-91.8147201804456,183.561326491592,-46.1418102382312));
#21987=CARTESIAN_POINT('Ctrl Pts',(-81.9298687787757,137.431831040152,-49.5305505033));
#21988=CARTESIAN_POINT('Ctrl Pts',(-20.8038733338462,173.87179773671,-39.0225342454562));
#21989=CARTESIAN_POINT('Ctrl Pts',(-91.5804344010687,183.608937488634,-47.2652752516501));
#21990=CARTESIAN_POINT('Ctrl Pts',(-81.7925509092854,137.513718286535,-50.6420203314529));
#21991=CARTESIAN_POINT('Ctrl Pts',(-21.2685350175652,173.512244042647,-37.6549923514553));
#21992=CARTESIAN_POINT('Ctrl Pts',(-91.4064133506295,183.64421947132,-47.8210101657326));
#21993=CARTESIAN_POINT('Ctrl Pts',(-81.4312911519869,137.727952582462,-52.8419520617065));
#21994=CARTESIAN_POINT('Ctrl Pts',(-22.4353472619568,172.608266146777,-35.1691826276842));
#21995=CARTESIAN_POINT('Ctrl Pts',(-90.9494152627793,183.73589269126,-48.9209760308471));
#21996=CARTESIAN_POINT('Ctrl Pts',(-81.2073409782417,137.86030323698,-53.930411905424));
#21997=CARTESIAN_POINT('Ctrl Pts',(-23.1321166236791,172.068023990567,-34.0542643968245));
#21998=CARTESIAN_POINT('Ctrl Pts',(-90.6664290227458,183.792284465073,-49.4652059527151));
#21999=CARTESIAN_POINT('Ctrl Pts',(-80.8076155883356,138.094725179005,-55.5463038168551));
#22000=CARTESIAN_POINT('Ctrl Pts',(-24.3018243019137,171.159251906869,-32.608821652411));
#22001=CARTESIAN_POINT('Ctrl Pts',(-90.1625642421299,183.891209812319,-50.273151908426));
#22002=CARTESIAN_POINT('Ctrl Pts',(-80.6637284362082,138.178851055812,-56.0821321396214));
#22003=CARTESIAN_POINT('Ctrl Pts',(-24.7092393480367,170.8424484307,-32.1672993257694));
#22004=CARTESIAN_POINT('Ctrl Pts',(-89.9813662332113,183.926573325791,-50.5410660698153));
#22005=CARTESIAN_POINT('Ctrl Pts',(-80.3547223160008,138.358774806128,-57.1482305947251));
#22006=CARTESIAN_POINT('Ctrl Pts',(-25.5534323448973,170.185187553971,-31.3653336068408));
#22007=CARTESIAN_POINT('Ctrl Pts',(-89.5927359269015,184.001812393928,-51.0741152973578));
#22008=CARTESIAN_POINT('Ctrl Pts',(-80.1897157463767,138.454503844763,-57.6778553276653));
#22009=CARTESIAN_POINT('Ctrl Pts',(-25.9891497436588,169.845558624407,-31.0053311458501));
#22010=CARTESIAN_POINT('Ctrl Pts',(-89.3854472959172,184.041657349327,-51.3389276638432));
#22011=CARTESIAN_POINT('Ctrl Pts',(-79.6691857343974,138.755113166885,-59.2411239335854));
#22012=CARTESIAN_POINT('Ctrl Pts',(-27.3043824228755,168.818754356815,-30.0625716779723));
#22013=CARTESIAN_POINT('Ctrl Pts',(-88.7324643102342,184.166044042608,-52.1205619667716));
#22014=CARTESIAN_POINT('Ctrl Pts',(-79.2865367003683,138.974361582824,-60.2551804226534));
#22015=CARTESIAN_POINT('Ctrl Pts',(-28.2054764565281,168.113208434832,-29.6008985931059));
#22016=CARTESIAN_POINT('Ctrl Pts',(-88.2536187741394,184.2558352071,-52.6275902113403));
#22017=CARTESIAN_POINT('Ctrl Pts',(-78.4554952448704,139.44519835826,-62.2322272830292));
#22018=CARTESIAN_POINT('Ctrl Pts',(-29.9870871732745,166.711325253611,-28.9902411417199));
#22019=CARTESIAN_POINT('Ctrl Pts',(-87.2172161146977,184.445814432147,-53.616113641501));
#22020=CARTESIAN_POINT('Ctrl Pts',(-78.0070853906616,139.696796360684,-63.1952037501853));
#22021=CARTESIAN_POINT('Ctrl Pts',(-30.8659062634836,166.016465199281,-28.8356077015459));
#22022=CARTESIAN_POINT('Ctrl Pts',(-86.6596376820301,184.54600608238,-54.0976018751081));
#22023=CARTESIAN_POINT('Ctrl Pts',(-77.048374490535,140.227844142847,-65.0739651883141));
#22024=CARTESIAN_POINT('Ctrl Pts',(-32.5550498620837,164.670719156008,-28.7930246590335));
#22025=CARTESIAN_POINT('Ctrl Pts',(-85.4720522235598,184.753776814215,-55.0369825941415));
#22026=CARTESIAN_POINT('Ctrl Pts',(-76.5380623346242,140.507300416309,-65.9897411795777));
#22027=CARTESIAN_POINT('Ctrl Pts',(-33.3652850012716,164.020134276596,-28.8993088042511));
#22028=CARTESIAN_POINT('Ctrl Pts',(-84.8420314669778,184.861358481738,-55.4948705898156));
#22029=CARTESIAN_POINT('Ctrl Pts',(-75.728170044288,140.944451383507,-67.3302212152897));
#22030=CARTESIAN_POINT('Ctrl Pts',(-34.5122899170826,163.088248299172,-29.2247287175038));
#22031=CARTESIAN_POINT('Ctrl Pts',(-83.8462836568007,185.026184135095,-56.1651106076315));
#22032=CARTESIAN_POINT('Ctrl Pts',(-75.4504275008882,141.093358021468,-67.7720166440731));
#22033=CARTESIAN_POINT('Ctrl Pts',(-34.8806149643643,162.787129232841,-29.3592240626014));
#22034=CARTESIAN_POINT('Ctrl Pts',(-83.5054586515878,185.081771633102,-56.3860083220514));
#22035=CARTESIAN_POINT('Ctrl Pts',(-74.8846583831958,141.394450480466,-68.638474298271));
#22036=CARTESIAN_POINT('Ctrl Pts',(-35.5848353719522,162.207090776343,-29.6738942085392));
#22037=CARTESIAN_POINT('Ctrl Pts',(-82.8126262261615,185.192937470074,-56.8192371491206));
#22038=CARTESIAN_POINT('Ctrl Pts',(-74.5961940186673,141.546875246922,-69.0639054241725));
#22039=CARTESIAN_POINT('Ctrl Pts',(-35.9216661334723,161.92746439315,-29.8536204285411));
#22040=CARTESIAN_POINT('Ctrl Pts',(-82.4600788359989,185.248607363413,-57.0319527121015));
#22041=CARTESIAN_POINT('Ctrl Pts',(-73.7147852409945,142.009051309513,-70.3181048368547));
#22042=CARTESIAN_POINT('Ctrl Pts',(-36.8788387621073,161.125452934343,-30.448321955934));
#22043=CARTESIAN_POINT('Ctrl Pts',(-81.3851340173047,185.415427325518,-57.6590524183968));
#22044=CARTESIAN_POINT('Ctrl Pts',(-73.1058526825644,142.323686171231,-71.1248228832094));
#22045=CARTESIAN_POINT('Ctrl Pts',(-37.4586012957459,160.629612122475,-30.9226581436019));
#22046=CARTESIAN_POINT('Ctrl Pts',(-80.6454711362611,185.526378252561,-58.0624114416317));
#22047=CARTESIAN_POINT('Ctrl Pts',(-71.8484094427491,142.962594416718,-72.6851127793295));
#22048=CARTESIAN_POINT('Ctrl Pts',(-38.4884482750362,159.723677205105,-31.9853928652137));
#22049=CARTESIAN_POINT('Ctrl Pts',(-79.1248432297244,185.745617009401,-58.8425563896376));
#22050=CARTESIAN_POINT('Ctrl Pts',(-71.1998903691279,143.28687342725,-73.4386712566775));
#22051=CARTESIAN_POINT('Ctrl Pts',(-38.9412443107916,159.311835992123,-32.571024190995));
#22052=CARTESIAN_POINT('Ctrl Pts',(-78.3438671457771,185.853907640827,-59.2193356283638));
#22053=CARTESIAN_POINT('Ctrl Pts',(-69.1983701639693,144.269870406751,-75.6262347306282));
#22054=CARTESIAN_POINT('Ctrl Pts',(-40.098518501438,158.209672336637,-34.4263336337102));
#22055=CARTESIAN_POINT('Ctrl Pts',(-75.9444956785313,186.171991112866,-60.313117365264));
#22056=CARTESIAN_POINT('Ctrl Pts',(-67.789611337796,144.938619930464,-76.9874494541838));
#22057=CARTESIAN_POINT('Ctrl Pts',(-40.6428501902966,157.618722485761,-35.8233464689691));
#22058=CARTESIAN_POINT('Ctrl Pts',(-74.2699390339847,186.374928413795,-60.9937247271315));
#22059=CARTESIAN_POINT('Ctrl Pts',(-65.5736968005695,145.947761291759,-78.9024214954926));
#22060=CARTESIAN_POINT('Ctrl Pts',(-41.1204746256597,156.930311424546,-38.039180340206));
#22061=CARTESIAN_POINT('Ctrl Pts',(-71.6611543736691,186.656097205558,-61.9512107477265));
#22062=CARTESIAN_POINT('Ctrl Pts',(-64.8158802459753,146.286035214527,-79.5209801538095));
#22063=CARTESIAN_POINT('Ctrl Pts',(-41.2244105509083,156.734894047821,-38.7871825470194));
#22064=CARTESIAN_POINT('Ctrl Pts',(-70.7730084836254,186.746172400419,-62.2604900769237));
#22065=CARTESIAN_POINT('Ctrl Pts',(-63.2798154046224,146.957025668062,-80.708101155254));
#22066=CARTESIAN_POINT('Ctrl Pts',(-41.3273505057767,156.405812865881,-40.28705578889));
#22067=CARTESIAN_POINT('Ctrl Pts',(-68.9812191627737,186.915817204625,-62.854050577608));
#22068=CARTESIAN_POINT('Ctrl Pts',(-62.5011418348097,147.28997967661,-81.2772464428291));
#22069=CARTESIAN_POINT('Ctrl Pts',(-41.3289113131743,156.270545080631,-41.0393070509114));
#22070=CARTESIAN_POINT('Ctrl Pts',(-68.0770491726709,186.995479791273,-63.1386232214322));
#22071=CARTESIAN_POINT('Ctrl Pts',(-60.1349066172685,148.279183910951,-82.9176021366126));
#22072=CARTESIAN_POINT('Ctrl Pts',(-41.1954499968666,155.945365284604,-43.2643582639517));
#22073=CARTESIAN_POINT('Ctrl Pts',(-65.3421452709541,187.21783448214,-63.9588010682709));
#22074=CARTESIAN_POINT('Ctrl Pts',(-58.5172177905218,148.925716472836,-83.9220069329356));
#22075=CARTESIAN_POINT('Ctrl Pts',(-40.9303152653076,155.823488084658,-44.7507715365026));
#22076=CARTESIAN_POINT('Ctrl Pts',(-63.4891393214523,187.343863770612,-64.4610034664955));
#22077=CARTESIAN_POINT('Ctrl Pts',(-55.2078389271008,150.183981588884,-85.7767676195814));
#22078=CARTESIAN_POINT('Ctrl Pts',(-40.0936579164813,155.727150148364,-47.6420141653999));
#22079=CARTESIAN_POINT('Ctrl Pts',(-59.7328291881618,187.546344672458,-65.388383809763));
#22080=CARTESIAN_POINT('Ctrl Pts',(-53.5161142772202,150.795743533889,-86.6270094856871));
#22081=CARTESIAN_POINT('Ctrl Pts',(-39.532641345483,155.7474211318,-49.0512964022449));
#22082=CARTESIAN_POINT('Ctrl Pts',(-57.8294753314208,187.622813755709,-65.8135047428673));
#22083=CARTESIAN_POINT('Ctrl Pts',(-50.0625427301627,151.977210695096,-88.1898645846761));
#22084=CARTESIAN_POINT('Ctrl Pts',(-38.1572551119495,155.887688976429,-51.7640573981651));
#22085=CARTESIAN_POINT('Ctrl Pts',(-53.9781482037484,187.721812660418,-66.5949322923142));
#22086=CARTESIAN_POINT('Ctrl Pts',(-48.300677812312,152.546933899424,-88.902415984378));
#22087=CARTESIAN_POINT('Ctrl Pts',(-37.3506839361543,156.004473544864,-53.0722212299062));
#22088=CARTESIAN_POINT('Ctrl Pts',(-52.0301478787376,187.744353908368,-66.9512079922001));
#22089=CARTESIAN_POINT('Ctrl Pts',(-45.6069622945489,153.365203420054,-89.8766149078073));
#22090=CARTESIAN_POINT('Ctrl Pts',(-35.968800254378,156.228899730153,-54.9617694105439));
#22091=CARTESIAN_POINT('Ctrl Pts',(-49.0772687551371,187.734687416337,-67.438307453898));
#22092=CARTESIAN_POINT('Ctrl Pts',(-44.6988593852777,153.632385143467,-90.1860654079167));
#22093=CARTESIAN_POINT('Ctrl Pts',(-35.4850829390786,156.310864009055,-55.574055857639));
#22094=CARTESIAN_POINT('Ctrl Pts',(-48.085971399696,187.724177624307,-67.5930327039756));
#22095=CARTESIAN_POINT('Ctrl Pts',(-42.8761650692597,154.151004745895,-90.7712192710136));
#22096=CARTESIAN_POINT('Ctrl Pts',(-34.4741829322119,156.485677849815,-56.7627908597524));
#22097=CARTESIAN_POINT('Ctrl Pts',(-46.1045568957785,187.688410388535,-67.8856096354897));
#22098=CARTESIAN_POINT('Ctrl Pts',(-41.961505308882,154.402506184776,-91.0470382563051));
#22099=CARTESIAN_POINT('Ctrl Pts',(-33.9476129855026,156.57835701425,-57.340037903017));
#22100=CARTESIAN_POINT('Ctrl Pts',(-45.1143442223383,187.663188471079,-68.0235191281666));
#22101=CARTESIAN_POINT('Ctrl Pts',(-39.2078728242664,155.133330023901,-91.8271696738661));
#22102=CARTESIAN_POINT('Ctrl Pts',(-32.3213222389258,156.865285274486,-59.0074115145415));
#22103=CARTESIAN_POINT('Ctrl Pts',(-42.1452357351134,187.565487512066,-68.413584836905));
#22104=CARTESIAN_POINT('Ctrl Pts',(-37.3592600401471,155.588971030372,-92.2842750101778));
#22105=CARTESIAN_POINT('Ctrl Pts',(-31.1537789584207,157.072069906232,-60.0612788653556));
#22106=CARTESIAN_POINT('Ctrl Pts',(-40.1678814465501,187.470978958484,-68.6421375051228));
#22107=CARTESIAN_POINT('Ctrl Pts',(-31.7765730898505,156.859230747872,-93.4851484356314));
#22108=CARTESIAN_POINT('Ctrl Pts',(-27.5050829333197,157.694479721468,-62.9822688779818));
#22109=CARTESIAN_POINT('Ctrl Pts',(-34.2418029492231,187.098995873263,-69.2425742177477));
#22110=CARTESIAN_POINT('Ctrl Pts',(-28.0057930465495,157.577245982649,-94.0596464150218));
#22111=CARTESIAN_POINT('Ctrl Pts',(-24.7937282524838,158.12831660148,-64.712605314168));
#22112=CARTESIAN_POINT('Ctrl Pts',(-30.2991672680022,186.733191336003,-69.5298232075278));
#22113=CARTESIAN_POINT('Ctrl Pts',(-20.3711181309634,158.744859575788,-94.8172777838099));
#22114=CARTESIAN_POINT('Ctrl Pts',(-18.9876739109975,158.899340600304,-67.6785024920399));
#22115=CARTESIAN_POINT('Ctrl Pts',(-22.4254742611568,185.761605939772,-69.9086388918881));
#22116=CARTESIAN_POINT('Ctrl Pts',(-16.5071336512573,159.19453344921,-95.));
#22117=CARTESIAN_POINT('Ctrl Pts',(-15.9015003142952,159.242363980563,-68.9409927140224));
#22118=CARTESIAN_POINT('Ctrl Pts',(-18.4943215078181,185.15585716373,-70.));
#22119=CARTESIAN_POINT('Ctrl Pts',(-12.5969447708578,159.503344737469,-95.));
#22120=CARTESIAN_POINT('Ctrl Pts',(-12.5969447708578,159.503344737469,-70.));
#22121=CARTESIAN_POINT('Ctrl Pts',(-14.5652173913043,184.425742352699,-70.));
#22122=CARTESIAN_POINT('Origin',(-14.5652173913044,184.425742352699,-95.));
#22123=CARTESIAN_POINT('Origin',(0.,0.,-95.));
#22124=CARTESIAN_POINT('Origin',(65.4347826086956,173.041293409847,-95.));
#22125=CARTESIAN_POINT('Ctrl Pts',(56.5812969309658,149.661474126996,-94.999999663102));
#22126=CARTESIAN_POINT('Ctrl Pts',(56.5824681415181,149.661031334401,-69.9968987143965));
#22127=CARTESIAN_POINT('Ctrl Pts',(65.4243928842982,173.048536665204,-69.9999998856919));
#22128=CARTESIAN_POINT('Ctrl Pts',(60.4989564059575,148.180355843715,-95.0002407886545));
#22129=CARTESIAN_POINT('Ctrl Pts',(60.0163273489374,148.362786890788,-70.9204250223862));
#22130=CARTESIAN_POINT('Ctrl Pts',(69.2022846505335,170.614767979795,-70.0001026705298));
#22131=CARTESIAN_POINT('Ctrl Pts',(64.3290814992657,146.556845989099,-94.8710407874072));
#22132=CARTESIAN_POINT('Ctrl Pts',(63.5298815986881,146.90048391857,-71.6775177805552));
#22133=CARTESIAN_POINT('Ctrl Pts',(72.8674869407948,168.080832069929,-69.9354862610261));
#22134=CARTESIAN_POINT('Ctrl Pts',(71.8188031734667,143.035546027701,-94.3981030531637));
#22135=CARTESIAN_POINT('Ctrl Pts',(70.5057678650493,143.683924979291,-72.8662379072352));
#22136=CARTESIAN_POINT('Ctrl Pts',(79.9886618996876,162.815535337367,-69.6989874289698));
#22137=CARTESIAN_POINT('Ctrl Pts',(75.4785580886895,141.137975699511,-94.0543379212976));
#22138=CARTESIAN_POINT('Ctrl Pts',(73.9797811251018,141.934709131226,-73.3100631433763));
#22139=CARTESIAN_POINT('Ctrl Pts',(83.4448180894751,160.084321423497,-69.5270912396781));
#22140=CARTESIAN_POINT('Ctrl Pts',(82.6353585459652,137.070560054605,-93.1809712878189));
#22141=CARTESIAN_POINT('Ctrl Pts',(80.8468574599951,138.140544890001,-73.9275707196295));
#22142=CARTESIAN_POINT('Ctrl Pts',(90.1649508997293,154.41848820675,-69.0903834130075));
#22143=CARTESIAN_POINT('Ctrl Pts',(86.1323917334308,134.900709490437,-92.6512484049633));
#22144=CARTESIAN_POINT('Ctrl Pts',(84.2505447772597,136.099279343518,-74.1094549887923));
#22145=CARTESIAN_POINT('Ctrl Pts',(93.4288956391719,151.483876162247,-68.8255110396083));
#22146=CARTESIAN_POINT('Ctrl Pts',(91.2562278085275,131.440284798247,-91.7313856490923));
#22147=CARTESIAN_POINT('Ctrl Pts',(89.3086164475295,132.791122113729,-74.2087035613002));
#22148=CARTESIAN_POINT('Ctrl Pts',(98.1868895303702,146.923477271295,-68.3655653126085));
#22149=CARTESIAN_POINT('Ctrl Pts',(92.9438609765793,130.252495749635,-91.4038190221124));
#22150=CARTESIAN_POINT('Ctrl Pts',(90.9728032539421,131.658236956057,-74.2136476278089));
#22151=CARTESIAN_POINT('Ctrl Pts',(99.7498644548314,145.376897997586,-68.2017775200415));
#22152=CARTESIAN_POINT('Ctrl Pts',(96.2782413450471,127.807567012862,-90.7084745843493));
#22153=CARTESIAN_POINT('Ctrl Pts',(94.2736611505731,129.316493186476,-74.1697159948556));
#22154=CARTESIAN_POINT('Ctrl Pts',(102.830397772462,142.229443445845,-67.8540969917478));
#22155=CARTESIAN_POINT('Ctrl Pts',(97.9169503291257,126.556249426074,-90.3423416598691));
#22156=CARTESIAN_POINT('Ctrl Pts',(95.903703016047,128.113362456395,-74.1215224666304));
#22157=CARTESIAN_POINT('Ctrl Pts',(104.340526700227,140.636086302123,-67.67102671681));
#22158=CARTESIAN_POINT('Ctrl Pts',(102.738637063097,122.725817074573,-89.194868194963));
#22159=CARTESIAN_POINT('Ctrl Pts',(100.689275592308,124.436982181698,-73.9049732929621));
#22160=CARTESIAN_POINT('Ctrl Pts',(108.773784825643,135.807660171076,-67.0972794877753));
#22161=CARTESIAN_POINT('Ctrl Pts',(105.832302044602,120.066719009486,-88.3636043219205));
#22162=CARTESIAN_POINT('Ctrl Pts',(103.806017904117,121.852642890427,-73.6651628264369));
#22163=CARTESIAN_POINT('Ctrl Pts',(111.604568501322,132.519638876911,-66.6816419285586));
#22164=CARTESIAN_POINT('Ctrl Pts',(111.787252032921,114.543020095905,-86.5841254176761));
#22165=CARTESIAN_POINT('Ctrl Pts',(109.828742608944,116.451539930578,-73.0190491201399));
#22166=CARTESIAN_POINT('Ctrl Pts',(117.032367740893,125.801765892224,-65.7918936812914));
#22167=CARTESIAN_POINT('Ctrl Pts',(114.648510013566,111.678405741599,-85.6358543716459));
#22168=CARTESIAN_POINT('Ctrl Pts',(112.744729844124,113.633819471468,-72.6152175520978));
#22169=CARTESIAN_POINT('Ctrl Pts',(119.629341825712,122.371918910437,-65.3177549806292));
#22170=CARTESIAN_POINT('Ctrl Pts',(120.142754803447,105.745286540606,-83.6326763250335));
#22171=CARTESIAN_POINT('Ctrl Pts',(118.360419510627,107.768760882995,-71.6629242837753));
#22172=CARTESIAN_POINT('Ctrl Pts',(124.599146017412,115.364277489534,-64.3161618621584));
#22173=CARTESIAN_POINT('Ctrl Pts',(122.775732250518,102.676780126255,-82.5777372261749));
#22174=CARTESIAN_POINT('Ctrl Pts',(121.068699599138,104.720063056805,-71.1159985199901));
#22175=CARTESIAN_POINT('Ctrl Pts',(126.971956052825,111.786495083743,-63.7886913953421));
#22176=CARTESIAN_POINT('Ctrl Pts',(125.924058053993,98.7124951748066,-81.1964639412465));
#22177=CARTESIAN_POINT('Ctrl Pts',(124.331930739111,100.743556004242,-70.3475688144439));
#22178=CARTESIAN_POINT('Ctrl Pts',(129.800754618314,107.216308630159,-63.0980550122952));
#22179=CARTESIAN_POINT('Ctrl Pts',(126.546567681521,97.9131968052379,-80.9170710194467));
#22180=CARTESIAN_POINT('Ctrl Pts',(124.974276451984,99.9453785320827,-70.1907346120513));
#22181=CARTESIAN_POINT('Ctrl Pts',(130.35964204207,106.297366154906,-62.958358650597));
#22182=CARTESIAN_POINT('Ctrl Pts',(127.777227456473,96.3016513053215,-80.3520788936366));
#22183=CARTESIAN_POINT('Ctrl Pts',(126.245180401018,98.3344970009766,-69.8692369319056));
#22184=CARTESIAN_POINT('Ctrl Pts',(131.463698417375,104.449503837098,-62.6758629153771));
#22185=CARTESIAN_POINT('Ctrl Pts',(128.385789213004,95.488818477247,-80.0662719859161));
#22186=CARTESIAN_POINT('Ctrl Pts',(126.874283998473,97.5211676556489,-69.7044590571902));
#22187=CARTESIAN_POINT('Ctrl Pts',(132.009235473065,103.519919460513,-62.5329596904946));
#22188=CARTESIAN_POINT('Ctrl Pts',(130.183236617954,93.0399172816704,-79.2028595772572));
#22189=CARTESIAN_POINT('Ctrl Pts',(128.730630618919,95.0726690760594,-69.2014135745425));
#22190=CARTESIAN_POINT('Ctrl Pts',(133.619372489814,100.726336511492,-62.1012543417964));
#22191=CARTESIAN_POINT('Ctrl Pts',(131.345830830401,91.3910083774034,-78.6184167040505));
#22192=CARTESIAN_POINT('Ctrl Pts',(129.936019778023,93.4178260930886,-68.8522667795203));
#22193=CARTESIAN_POINT('Ctrl Pts',(134.659248944961,98.8546953978921,-61.8090337383792));
#22194=CARTESIAN_POINT('Ctrl Pts',(136.984252256763,83.066320816122,-75.6545459910939));
#22195=CARTESIAN_POINT('Ctrl Pts',(135.733435507954,85.1282711420036,-67.0626755844076));
#22196=CARTESIAN_POINT('Ctrl Pts',(139.69593319768,89.4486190536225,-60.3271033604134));
#22197=CARTESIAN_POINT('Ctrl Pts',(140.939665730898,76.1514359804232,-73.1515201298415));
#22198=CARTESIAN_POINT('Ctrl Pts',(139.892479128959,78.1140806329442,-65.4234070407235));
#22199=CARTESIAN_POINT('Ctrl Pts',(143.208042281703,81.7712744848519,-59.0755984780511));
#22200=CARTESIAN_POINT('Ctrl Pts',(146.074442213326,65.4065361918843,-69.2286486640292));
#22201=CARTESIAN_POINT('Ctrl Pts',(145.300074703784,67.1397517802941,-62.7372455747638));
#22202=CARTESIAN_POINT('Ctrl Pts',(147.752894595048,69.9881927669513,-57.1141792381744));
#22203=CARTESIAN_POINT('Ctrl Pts',(147.652339743601,61.7625472805127,-67.8926978272171));
#22204=CARTESIAN_POINT('Ctrl Pts',(146.960165150244,63.4242781048417,-61.8087879465894));
#22205=CARTESIAN_POINT('Ctrl Pts',(149.146622559743,66.0158544895779,-56.4462099719241));
#22206=CARTESIAN_POINT('Ctrl Pts',(149.817529237806,56.2019959846926,-65.8479415997114));
#22207=CARTESIAN_POINT('Ctrl Pts',(149.242347721494,57.7367729878032,-60.3647058289904));
#22208=CARTESIAN_POINT('Ctrl Pts',(151.056362855309,59.9840340630083,-55.4238420679245));
#22209=CARTESIAN_POINT('Ctrl Pts',(150.505613144304,54.3327017345152,-65.1595391420024));
#22210=CARTESIAN_POINT('Ctrl Pts',(149.967111817076,55.8263294600576,-59.8759432089222));
#22211=CARTESIAN_POINT('Ctrl Pts',(151.662764461086,57.9611955550307,-55.0796443851654));
#22212=CARTESIAN_POINT('Ctrl Pts',(151.486795724974,51.5048176135849,-64.1168149427468));
#22213=CARTESIAN_POINT('Ctrl Pts',(151.001777270418,52.9318234663437,-59.1304989011081));
#22214=CARTESIAN_POINT('Ctrl Pts',(152.526890248574,54.9076662607108,-54.5582878352699));
#22215=CARTESIAN_POINT('Ctrl Pts',(151.805631706267,50.5573531931324,-63.7672407289972));
#22216=CARTESIAN_POINT('Ctrl Pts',(151.337862433627,51.9624117296005,-58.8800286243506));
#22217=CARTESIAN_POINT('Ctrl Pts',(152.807586254088,53.8857006249786,-54.3835026132985));
#22218=CARTESIAN_POINT('Ctrl Pts',(152.424429813256,48.6599319331378,-63.0667763221948));
#22219=CARTESIAN_POINT('Ctrl Pts',(151.990284568165,50.0203688638623,-58.3767438321395));
#22220=CARTESIAN_POINT('Ctrl Pts',(153.352185445787,51.8411536809008,-54.0332742392006));
#22221=CARTESIAN_POINT('Ctrl Pts',(152.724480699873,47.7097795578204,-62.7158144756994));
#22222=CARTESIAN_POINT('Ctrl Pts',(152.306775554914,49.0474544815894,-58.1238602850607));
#22223=CARTESIAN_POINT('Ctrl Pts',(153.616167012447,50.8183589268311,-53.8577952610939));
#22224=CARTESIAN_POINT('Ctrl Pts',(155.341538509173,39.1455096494411,-59.5507777161094));
#22225=CARTESIAN_POINT('Ctrl Pts',(155.053646875419,40.3201454141209,-55.8492067218196));
#22226=CARTESIAN_POINT('Ctrl Pts',(155.917931197662,41.6079957503088,-52.2752944281586));
#22227=CARTESIAN_POINT('Ctrl Pts',(157.07810627687,31.4415608593237,-56.6925205993872));
#22228=CARTESIAN_POINT('Ctrl Pts',(156.90198155413,32.3845089243095,-53.737474669054));
#22229=CARTESIAN_POINT('Ctrl Pts',(157.44054163938,33.3840425942794,-50.8461835759691));
#22230=CARTESIAN_POINT('Ctrl Pts',(158.82519295691,19.7505414457421,-52.3482901793705));
#22231=CARTESIAN_POINT('Ctrl Pts',(158.754292373171,20.3422965292876,-50.5031839537118));
#22232=CARTESIAN_POINT('Ctrl Pts',(158.971479743882,20.9484526942674,-48.6740963430449));
#22233=CARTESIAN_POINT('Ctrl Pts',(159.263969037573,15.8309336660904,-50.8906501993346));
#22234=CARTESIAN_POINT('Ctrl Pts',(159.219812676319,16.3052169394273,-49.4139701412218));
#22235=CARTESIAN_POINT('Ctrl Pts',(159.355678879032,16.7866326264316,-47.9452859158802));
#22236=CARTESIAN_POINT('Ctrl Pts',(159.704601275411,9.91705122742161,-48.6905305271729));
#22237=CARTESIAN_POINT('Ctrl Pts',(159.686873998594,10.2140889512697,-47.7668807500635));
#22238=CARTESIAN_POINT('Ctrl Pts',(159.741443596687,10.5129289476784,-46.845240648104));
#22239=CARTESIAN_POINT('Ctrl Pts',(159.815185663009,7.94000627714555,-47.9548772374033));
#22240=CARTESIAN_POINT('Ctrl Pts',(159.804111417455,8.17781928521151,-47.2156464805718));
#22241=CARTESIAN_POINT('Ctrl Pts',(159.838239575783,8.41652647505475,-46.4774188965339));
#22242=CARTESIAN_POINT('Ctrl Pts',(159.962941406071,3.97424771510734,-46.4790883105662));
#22243=CARTESIAN_POINT('Ctrl Pts',(159.960706190386,4.09363866395126,-46.109411006716));
#22244=CARTESIAN_POINT('Ctrl Pts',(159.967567107836,4.21229224969148,-45.7395342702298));
#22245=CARTESIAN_POINT('Ctrl Pts',(160.,1.98404404958242,-45.7383979472562));
#22246=CARTESIAN_POINT('Ctrl Pts',(160.,2.04346271857147,-45.5537959634005));
#22247=CARTESIAN_POINT('Ctrl Pts',(160.,2.10288127222745,-45.3691939804612));
#22248=CARTESIAN_POINT('Ctrl Pts',(160.,0.,-45.));
#22249=CARTESIAN_POINT('Ctrl Pts',(160.,0.,-45.));
#22250=CARTESIAN_POINT('Ctrl Pts',(160.,0.,-45.));
#22251=CARTESIAN_POINT('Origin',(180.,-125.,85.));
#22252=CARTESIAN_POINT('',(180.,-137.5,73.9644660940673));
#22253=CARTESIAN_POINT('',(180.,-137.5,-73.9644660940672));
#22254=CARTESIAN_POINT('',(180.,-137.5,85.));
#22255=CARTESIAN_POINT('',(180.,-127.5,-73.9644660940672));
#22256=CARTESIAN_POINT('',(180.,-125.,-73.9644660940672));
#22257=CARTESIAN_POINT('',(180.,-127.5,73.9644660940673));
#22258=CARTESIAN_POINT('',(180.,-127.5,85.));
#22259=CARTESIAN_POINT('',(180.,-125.,73.9644660940673));
#22260=CARTESIAN_POINT('Origin',(180.,-140.,85.));
#22261=CARTESIAN_POINT('',(168.964466094067,-140.,82.5));
#22262=CARTESIAN_POINT('',(97.2111104761179,-140.,82.5));
#22263=CARTESIAN_POINT('',(180.,-140.,82.5));
#22264=CARTESIAN_POINT('',(97.2111104761179,-140.,-82.5));
#22265=CARTESIAN_POINT('',(97.2111104761179,-140.,85.));
#22266=CARTESIAN_POINT('',(168.964466094067,-140.,-82.5));
#22267=CARTESIAN_POINT('',(170.,-140.,-82.5));
#22268=CARTESIAN_POINT('',(177.5,-140.,-73.9644660940671));
#22269=CARTESIAN_POINT('',(258.232233047034,-140.,6.76776695296644));
#22270=CARTESIAN_POINT('',(177.5,-140.,73.9644660940673));
#22271=CARTESIAN_POINT('',(177.5,-140.,85.));
#22272=CARTESIAN_POINT('',(173.232233047034,-140.,78.2322330470336));
#22273=CARTESIAN_POINT('Origin',(0.,0.,85.));
#22274=CARTESIAN_POINT('',(104.163333279998,-137.5,85.));
#22275=CARTESIAN_POINT('',(168.964466094067,-137.5,85.));
#22276=CARTESIAN_POINT('',(0.,-137.5,85.));
#22277=CARTESIAN_POINT('',(168.964466094067,-127.5,85.));
#22278=CARTESIAN_POINT('',(168.964466094067,0.,85.));
#22279=CARTESIAN_POINT('',(116.189500386222,-127.5,85.));
#22280=CARTESIAN_POINT('',(0.,-127.5,85.));
#22281=CARTESIAN_POINT('Origin',(0.,0.,85.));
#22282=CARTESIAN_POINT('Origin',(0.,0.,-85.));
#22283=CARTESIAN_POINT('',(168.964466094067,-137.5,-85.));
#22284=CARTESIAN_POINT('',(104.163333279998,-137.5,-85.));
#22285=CARTESIAN_POINT('',(96.4365076099295,-137.5,-85.));
#22286=CARTESIAN_POINT('',(116.189500386223,-127.5,-85.));
#22287=CARTESIAN_POINT('Origin',(0.,0.,-85.));
#22288=CARTESIAN_POINT('',(168.964466094067,-127.5,-85.));
#22289=CARTESIAN_POINT('',(170.,-127.5,-85.));
#22290=CARTESIAN_POINT('',(168.964466094067,-140.,-85.));
#22291=CARTESIAN_POINT('Origin',(150.,-79.9999999999999,-47.));
#22292=CARTESIAN_POINT('',(150.,-122.5,-44.5));
#22293=CARTESIAN_POINT('',(150.,-80.6225774829854,-44.5));
#22294=CARTESIAN_POINT('',(150.,-79.9999999999999,-44.5));
#22295=CARTESIAN_POINT('',(150.,-80.6225774829854,-37.5));
#22296=CARTESIAN_POINT('',(150.,-80.6225774829854,-35.));
#22297=CARTESIAN_POINT('',(150.,-122.5,-37.5));
#22298=CARTESIAN_POINT('',(150.,-125.,-37.5));
#22299=CARTESIAN_POINT('',(150.,-122.5,-47.));
#22300=CARTESIAN_POINT('Origin',(0.,0.,-47.));
#22301=CARTESIAN_POINT('',(147.5,-122.5,-47.));
#22302=CARTESIAN_POINT('',(121.449578014911,-122.5,-47.));
#22303=CARTESIAN_POINT('',(0.,-122.5,-47.));
#22304=CARTESIAN_POINT('',(147.5,-89.4427190999916,-47.));
#22305=CARTESIAN_POINT('Origin',(0.,0.,-47.));
#22306=CARTESIAN_POINT('',(147.5,0.,-47.));
#22307=CARTESIAN_POINT('Origin',(0.,0.,-35.));
#22308=CARTESIAN_POINT('',(147.5,-122.5,-35.));
#22309=CARTESIAN_POINT('',(147.5,-89.4427190999916,-35.));
#22310=CARTESIAN_POINT('',(147.5,-79.9999999999999,-35.));
#22311=CARTESIAN_POINT('',(121.449578014911,-122.5,-35.));
#22312=CARTESIAN_POINT('Origin',(0.,0.,-35.));
#22313=CARTESIAN_POINT('',(150.,-122.5,-35.));
#22314=CARTESIAN_POINT('Origin',(150.,-79.9999999999999,47.));
#22315=CARTESIAN_POINT('',(150.,-122.5,37.5));
#22316=CARTESIAN_POINT('',(150.,-80.6225774829854,37.5));
#22317=CARTESIAN_POINT('',(150.,-79.9999999999999,37.5));
#22318=CARTESIAN_POINT('',(150.,-80.6225774829854,44.5));
#22319=CARTESIAN_POINT('',(150.,-80.6225774829854,47.));
#22320=CARTESIAN_POINT('',(150.,-122.5,44.5));
#22321=CARTESIAN_POINT('',(150.,-125.,44.5));
#22322=CARTESIAN_POINT('',(150.,-122.5,35.));
#22323=CARTESIAN_POINT('Origin',(0.,0.,47.));
#22324=CARTESIAN_POINT('',(147.5,-122.5,47.));
#22325=CARTESIAN_POINT('',(147.5,-89.4427190999916,47.));
#22326=CARTESIAN_POINT('',(147.5,-79.9999999999999,47.));
#22327=CARTESIAN_POINT('',(121.449578014911,-122.5,47.));
#22328=CARTESIAN_POINT('Origin',(0.,0.,47.));
#22329=CARTESIAN_POINT('',(0.,-122.5,47.));
#22330=CARTESIAN_POINT('Origin',(0.,0.,35.));
#22331=CARTESIAN_POINT('',(147.5,-122.5,35.));
#22332=CARTESIAN_POINT('',(121.449578014911,-122.5,35.));
#22333=CARTESIAN_POINT('',(115.217186218029,-122.5,35.));
#22334=CARTESIAN_POINT('',(147.5,-89.4427190999916,35.));
#22335=CARTESIAN_POINT('Origin',(0.,0.,35.));
#22336=CARTESIAN_POINT('',(147.5,0.,35.));
#22337=CARTESIAN_POINT('Origin',(-180.,-125.,85.));
#22338=CARTESIAN_POINT('',(-180.,-127.5,73.9644660940671));
#22339=CARTESIAN_POINT('',(-180.,-127.5,-73.9644660940673));
#22340=CARTESIAN_POINT('',(-180.,-127.5,85.));
#22341=CARTESIAN_POINT('',(-180.,-137.5,-73.9644660940673));
#22342=CARTESIAN_POINT('',(-180.,-140.,-73.9644660940673));
#22343=CARTESIAN_POINT('',(-180.,-137.5,73.9644660940671));
#22344=CARTESIAN_POINT('',(-180.,-137.5,85.));
#22345=CARTESIAN_POINT('',(-180.,-125.,73.9644660940671));
#22346=CARTESIAN_POINT('Origin',(0.,0.,85.));
#22347=CARTESIAN_POINT('',(-168.964466094067,-127.5,85.));
#22348=CARTESIAN_POINT('',(-168.964466094067,-137.5,85.));
#22349=CARTESIAN_POINT('',(-168.964466094067,0.,85.));
#22350=CARTESIAN_POINT('',(-104.163333279998,-137.5,85.));
#22351=CARTESIAN_POINT('',(-96.4365076099295,-137.5,85.));
#22352=CARTESIAN_POINT('',(-116.189500386222,-127.5,85.));
#22353=CARTESIAN_POINT('Origin',(0.,0.,85.));
#22354=CARTESIAN_POINT('',(-170.,-127.5,85.));
#22355=CARTESIAN_POINT('Origin',(0.,0.,-85.));
#22356=CARTESIAN_POINT('',(-168.964466094067,-127.5,-85.));
#22357=CARTESIAN_POINT('',(-116.189500386223,-127.5,-85.));
#22358=CARTESIAN_POINT('',(0.,-127.5,-85.));
#22359=CARTESIAN_POINT('',(-104.163333279998,-137.5,-85.));
#22360=CARTESIAN_POINT('Origin',(0.,0.,-85.));
#22361=CARTESIAN_POINT('',(-168.964466094067,-137.5,-85.));
#22362=CARTESIAN_POINT('',(0.,-137.5,-85.));
#22363=CARTESIAN_POINT('',(-168.964466094067,-125.,-85.));
#22364=CARTESIAN_POINT('Origin',(-150.,-79.9999999999999,-47.));
#22365=CARTESIAN_POINT('',(-150.,-122.5,-44.5));
#22366=CARTESIAN_POINT('',(-150.,-122.5,-37.5));
#22367=CARTESIAN_POINT('',(-150.,-122.5,-47.));
#22368=CARTESIAN_POINT('',(-150.,-80.6225774829854,-37.5));
#22369=CARTESIAN_POINT('',(-150.,-79.9999999999999,-37.5));
#22370=CARTESIAN_POINT('',(-150.,-80.6225774829854,-44.5));
#22371=CARTESIAN_POINT('',(-150.,-80.6225774829854,-47.));
#22372=CARTESIAN_POINT('',(-150.,-125.,-44.5));
#22373=CARTESIAN_POINT('Origin',(0.,0.,-47.));
#22374=CARTESIAN_POINT('',(-147.5,-122.5,-47.));
#22375=CARTESIAN_POINT('',(-147.5,-89.4427190999916,-47.));
#22376=CARTESIAN_POINT('',(-147.5,-79.9999999999999,-47.));
#22377=CARTESIAN_POINT('Origin',(0.,0.,-47.));
#22378=CARTESIAN_POINT('',(-150.,-122.5,-47.));
#22379=CARTESIAN_POINT('Origin',(0.,0.,-35.));
#22380=CARTESIAN_POINT('',(-147.5,-122.5,-35.));
#22381=CARTESIAN_POINT('',(0.,-122.5,-35.));
#22382=CARTESIAN_POINT('',(-147.5,-89.4427190999916,-35.));
#22383=CARTESIAN_POINT('Origin',(0.,0.,-35.));
#22384=CARTESIAN_POINT('',(-147.5,0.,-35.));
#22385=CARTESIAN_POINT('Origin',(-150.,-79.9999999999999,47.));
#22386=CARTESIAN_POINT('',(-150.,-122.5,37.5));
#22387=CARTESIAN_POINT('',(-150.,-122.5,44.5));
#22388=CARTESIAN_POINT('',(-150.,-122.5,47.));
#22389=CARTESIAN_POINT('',(-150.,-80.6225774829854,44.5));
#22390=CARTESIAN_POINT('',(-150.,-79.9999999999999,44.5));
#22391=CARTESIAN_POINT('',(-150.,-80.6225774829854,37.5));
#22392=CARTESIAN_POINT('',(-150.,-80.6225774829854,35.));
#22393=CARTESIAN_POINT('',(-150.,-125.,37.5));
#22394=CARTESIAN_POINT('Origin',(0.,0.,47.));
#22395=CARTESIAN_POINT('',(-147.5,-122.5,47.));
#22396=CARTESIAN_POINT('',(-115.217186218029,-122.5,47.));
#22397=CARTESIAN_POINT('',(-147.5,-89.4427190999916,47.));
#22398=CARTESIAN_POINT('Origin',(0.,0.,47.));
#22399=CARTESIAN_POINT('',(-147.5,0.,47.));
#22400=CARTESIAN_POINT('Origin',(0.,0.,35.));
#22401=CARTESIAN_POINT('',(-147.5,-122.5,35.));
#22402=CARTESIAN_POINT('',(-147.5,-89.4427190999916,35.));
#22403=CARTESIAN_POINT('',(-147.5,-79.9999999999999,35.));
#22404=CARTESIAN_POINT('Origin',(0.,0.,35.));
#22405=CARTESIAN_POINT('',(0.,-122.5,35.));
#22406=CARTESIAN_POINT('Origin',(-170.,0.,85.));
#22407=CARTESIAN_POINT('',(-170.732233047034,-127.5,84.2677669529664));
#22408=CARTESIAN_POINT('',(-179.267766952966,-127.5,75.7322330470335));
#22409=CARTESIAN_POINT('',(-180.,-127.5,74.9999999999999));
#22410=CARTESIAN_POINT('',(-179.267766952966,-137.5,75.7322330470335));
#22411=CARTESIAN_POINT('',(-179.267766952966,-140.,75.7322330470335));
#22412=CARTESIAN_POINT('',(-170.732233047034,-137.5,84.2677669529664));
#22413=CARTESIAN_POINT('',(-170.,-137.5,85.));
#22414=CARTESIAN_POINT('',(-170.732233047034,0.,84.2677669529664));
#22415=CARTESIAN_POINT('Origin',(-180.,-125.,-75.));
#22416=CARTESIAN_POINT('',(-179.267766952966,-127.5,-75.7322330470336));
#22417=CARTESIAN_POINT('',(-170.732233047034,-127.5,-84.2677669529664));
#22418=CARTESIAN_POINT('',(-170.,-127.5,-85.));
#22419=CARTESIAN_POINT('',(-170.732233047034,-137.5,-84.2677669529664));
#22420=CARTESIAN_POINT('',(-170.732233047034,-140.,-84.2677669529664));
#22421=CARTESIAN_POINT('',(-179.267766952966,-137.5,-75.7322330470336));
#22422=CARTESIAN_POINT('',(-180.,-137.5,-75.));
#22423=CARTESIAN_POINT('',(-179.267766952966,-125.,-75.7322330470336));
#22424=CARTESIAN_POINT('Origin',(180.,-125.,75.));
#22425=CARTESIAN_POINT('',(170.732233047034,-137.5,84.2677669529664));
#22426=CARTESIAN_POINT('',(179.267766952966,-137.5,75.7322330470336));
#22427=CARTESIAN_POINT('',(180.,-137.5,75.));
#22428=CARTESIAN_POINT('',(179.267766952966,-127.5,75.7322330470336));
#22429=CARTESIAN_POINT('',(179.267766952966,-125.,75.7322330470336));
#22430=CARTESIAN_POINT('',(170.732233047034,-127.5,84.2677669529664));
#22431=CARTESIAN_POINT('',(180.,-127.5,75.));
#22432=CARTESIAN_POINT('',(170.732233047034,-125.,84.2677669529664));
#22433=CARTESIAN_POINT('Origin',(170.,0.,-85.));
#22434=CARTESIAN_POINT('',(179.267766952966,-127.5,-75.7322330470335));
#22435=CARTESIAN_POINT('',(179.267766952966,-137.5,-75.7322330470335));
#22436=CARTESIAN_POINT('',(179.267766952966,0.,-75.7322330470335));
#22437=CARTESIAN_POINT('',(170.732233047034,-137.5,-84.2677669529664));
#22438=CARTESIAN_POINT('',(170.,-137.5,-85.));
#22439=CARTESIAN_POINT('',(170.732233047034,-127.5,-84.2677669529664));
#22440=CARTESIAN_POINT('',(170.732233047034,-125.,-84.2677669529664));
#22441=CARTESIAN_POINT('',(170.,-127.5,-85.));
#22442=CARTESIAN_POINT('Origin',(0.,0.,115.));
#22443=CARTESIAN_POINT('Origin',(0.,0.,125.));
#22444=CARTESIAN_POINT('Origin',(0.,-122.5,-49.5));
#22445=CARTESIAN_POINT('Origin',(-147.5,-122.5,-49.5));
#22446=CARTESIAN_POINT('Origin',(-147.5,-79.9999999999999,-44.5));
#22447=CARTESIAN_POINT('Ctrl Pts',(-147.5,-89.4427190999916,-47.));
#22448=CARTESIAN_POINT('Ctrl Pts',(-147.692029124167,-88.8093685912607,
-47.));
#22449=CARTESIAN_POINT('Ctrl Pts',(-147.881019325447,-88.1768396525117,
-46.9784293604652));
#22450=CARTESIAN_POINT('Ctrl Pts',(-148.067032921855,-87.5451886197927,
-46.9349710385975));
#22451=CARTESIAN_POINT('Ctrl Pts',(-148.113199638035,-87.3884191442505,
-46.9241851172987));
#22452=CARTESIAN_POINT('Ctrl Pts',(-148.159182993745,-87.2317038217232,
-46.9120507147773));
#22453=CARTESIAN_POINT('Ctrl Pts',(-148.204983936061,-87.075043664733,-46.8985625026983));
#22454=CARTESIAN_POINT('Ctrl Pts',(-148.227650188964,-86.9975147197269,
-46.8918873730891));
#22455=CARTESIAN_POINT('Ctrl Pts',(-148.250265804087,-86.9200215223737,
-46.8848824575639));
#22456=CARTESIAN_POINT('Ctrl Pts',(-148.272833473781,-86.8425552539348,
-46.877546723474));
#22457=CARTESIAN_POINT('Ctrl Pts',(-148.349179005414,-86.5804899398113,
-46.8527302259542));
#22458=CARTESIAN_POINT('Ctrl Pts',(-148.42497434185,-86.3187382386177,-46.8240687356948));
#22459=CARTESIAN_POINT('Ctrl Pts',(-148.500300623518,-86.0570314559301,
-46.7911753910845));
#22460=CARTESIAN_POINT('Ctrl Pts',(-148.548487711945,-85.8896146181409,
-46.7701331403549));
#22461=CARTESIAN_POINT('Ctrl Pts',(-148.596482723484,-85.7222162995132,
-46.7473581833852));
#22462=CARTESIAN_POINT('Ctrl Pts',(-148.644305530043,-85.5547679896948,
-46.7227381433699));
#22463=CARTESIAN_POINT('Ctrl Pts',(-148.705029122316,-85.3421484547092,
-46.6914765470896));
#22464=CARTESIAN_POINT('Ctrl Pts',(-148.765481316907,-85.1294146681287,
-46.6572181679748));
#22465=CARTESIAN_POINT('Ctrl Pts',(-148.825445173605,-84.9173615305767,
-46.6197236282395));
#22466=CARTESIAN_POINT('Ctrl Pts',(-148.844370664369,-84.8504343861742,
-46.6078897902489));
#22467=CARTESIAN_POINT('Ctrl Pts',(-148.863247416388,-84.7835753431854,
-46.5957333861149));
#22468=CARTESIAN_POINT('Ctrl Pts',(-148.882068323811,-84.7168103169457,
-46.5832463102145));
#22469=CARTESIAN_POINT('Ctrl Pts',(-148.922791444531,-84.5723496827009,
-46.5562278095707));
#22470=CARTESIAN_POINT('Ctrl Pts',(-148.963298334261,-84.4281714850036,
-46.5276326949765));
#22471=CARTESIAN_POINT('Ctrl Pts',(-149.003534667861,-84.2844711674245,
-46.4973441122003));
#22472=CARTESIAN_POINT('Ctrl Pts',(-149.04618468001,-84.1321506217299,-46.4652385919447));
#22473=CARTESIAN_POINT('Ctrl Pts',(-149.088661184858,-83.9798999176171,
-46.431152727177));
#22474=CARTESIAN_POINT('Ctrl Pts',(-149.130874866099,-83.8280577825329,
-46.3948300518332));
#22475=CARTESIAN_POINT('Ctrl Pts',(-149.153428770871,-83.7469316415657,
-46.3754235907832));
#22476=CARTESIAN_POINT('Ctrl Pts',(-149.175907457634,-83.6659227742882,
-46.3553781599173));
#22477=CARTESIAN_POINT('Ctrl Pts',(-149.198295785931,-83.5850879913779,
-46.3346512081709));
#22478=CARTESIAN_POINT('Ctrl Pts',(-149.227912989408,-83.4781527981097,
-46.3072318162821));
#22479=CARTESIAN_POINT('Ctrl Pts',(-149.257371929218,-83.3715229743104,
-46.2786215766946));
#22480=CARTESIAN_POINT('Ctrl Pts',(-149.286670239298,-83.265210223348,-46.2486743918971));
#22481=CARTESIAN_POINT('Ctrl Pts',(-149.30536712493,-83.1973661278873,-46.2295634231207));
#22482=CARTESIAN_POINT('Ctrl Pts',(-149.323998297478,-83.1296521693962,
-46.2099077590292));
#22483=CARTESIAN_POINT('Ctrl Pts',(-149.342561050911,-83.0620783213206,
-46.1896652845064));
#22484=CARTESIAN_POINT('Ctrl Pts',(-149.371267458519,-82.95757860723,-46.1583612688204));
#22485=CARTESIAN_POINT('Ctrl Pts',(-149.399774767598,-82.8535435891935,
-46.1257402426392));
#22486=CARTESIAN_POINT('Ctrl Pts',(-149.428061694081,-82.7500633861384,
-46.0915220141326));
#22487=CARTESIAN_POINT('Ctrl Pts',(-149.454923581065,-82.6517963113774,
-46.0590276324095));
#22488=CARTESIAN_POINT('Ctrl Pts',(-149.48158676368,-82.5540293874111,-46.0250930589968));
#22489=CARTESIAN_POINT('Ctrl Pts',(-149.508023085913,-82.4568752754022,
-45.9894478142867));
#22490=CARTESIAN_POINT('Ctrl Pts',(-149.512553176896,-82.4402270834634,
-45.9833396953057));
#22491=CARTESIAN_POINT('Ctrl Pts',(-149.517076580988,-82.4235969779237,
-45.9771812656855));
#22492=CARTESIAN_POINT('Ctrl Pts',(-149.521593124104,-82.406985643267,-45.9709710636017));
#22493=CARTESIAN_POINT('Ctrl Pts',(-149.546047412515,-82.3170455368253,
-45.9373466590614));
#22494=CARTESIAN_POINT('Ctrl Pts',(-149.570311794236,-82.2276143985462,
-45.9021926455905));
#22495=CARTESIAN_POINT('Ctrl Pts',(-149.594353719118,-82.1388178247614,
-45.8652538583403));
#22496=CARTESIAN_POINT('Ctrl Pts',(-149.612438155897,-82.07202466936,-45.8374683475715));
#22497=CARTESIAN_POINT('Ctrl Pts',(-149.63039654831,-82.0055912015912,-45.8086724394745));
#22498=CARTESIAN_POINT('Ctrl Pts',(-149.648211128679,-81.9395854582945,
-45.7787450670962));
#22499=CARTESIAN_POINT('Ctrl Pts',(-149.655934224025,-81.9109702095313,
-45.7657707536098));
#22500=CARTESIAN_POINT('Ctrl Pts',(-149.663637104736,-81.8824099165123,
-45.7525620980052));
#22501=CARTESIAN_POINT('Ctrl Pts',(-149.67131055004,-81.8539394834478,-45.7391147562166));
#22502=CARTESIAN_POINT('Ctrl Pts',(-149.685698655415,-81.8005559543078,
-45.7139002973917));
#22503=CARTESIAN_POINT('Ctrl Pts',(-149.699999360789,-81.7474243597972,
-45.6878211143421));
#22504=CARTESIAN_POINT('Ctrl Pts',(-149.714175605301,-81.6946906272146,
-45.6607798441796));
#22505=CARTESIAN_POINT('Ctrl Pts',(-149.727286670739,-81.6459192182512,
-45.6357704093948));
#22506=CARTESIAN_POINT('Ctrl Pts',(-149.740291333114,-81.5974878781543,
-45.6099378953754));
#22507=CARTESIAN_POINT('Ctrl Pts',(-149.75314895044,-81.549552803929,-45.583195140044));
#22508=CARTESIAN_POINT('Ctrl Pts',(-149.76292982072,-81.5130882918071,-45.5628517580484));
#22509=CARTESIAN_POINT('Ctrl Pts',(-149.772625404106,-81.4769116545282,
-45.5419814455611));
#22510=CARTESIAN_POINT('Ctrl Pts',(-149.782212501331,-81.4411109947051,
-45.5205420615612));
#22511=CARTESIAN_POINT('Ctrl Pts',(-149.792712453297,-81.4019015030656,
-45.4970612835013));
#22512=CARTESIAN_POINT('Ctrl Pts',(-149.80309231573,-81.3631061432697,-45.4728977376122));
#22513=CARTESIAN_POINT('Ctrl Pts',(-149.813325028167,-81.3248298095044,
-45.4479419883158));
#22514=CARTESIAN_POINT('Ctrl Pts',(-149.822817814989,-81.2893212306204,
-45.4247907848088));
#22515=CARTESIAN_POINT('Ctrl Pts',(-149.832167251568,-81.2543175533045,
-45.4010004533823));
#22516=CARTESIAN_POINT('Ctrl Pts',(-149.841373631764,-81.2198208404939,
-45.3764055282848));
#22517=CARTESIAN_POINT('Ctrl Pts',(-149.850444720927,-81.1858310691553,
-45.352172034365));
#22518=CARTESIAN_POINT('Ctrl Pts',(-149.859377062136,-81.1523329411743,
-45.3271576500975));
#22519=CARTESIAN_POINT('Ctrl Pts',(-149.868158592942,-81.1193744240714,
-45.3011827166068));
#22520=CARTESIAN_POINT('Ctrl Pts',(-149.876313696672,-81.0887669899374,
-45.2770606948705));
#22521=CARTESIAN_POINT('Ctrl Pts',(-149.884338741479,-81.0586248955663,
-45.2521102789363));
#22522=CARTESIAN_POINT('Ctrl Pts',(-149.8922125854,-81.0290296766821,-45.2261677408448));
#22523=CARTESIAN_POINT('Ctrl Pts',(-149.892817407753,-81.0267563461319,
-45.2241749877375));
#22524=CARTESIAN_POINT('Ctrl Pts',(-149.893421331922,-81.0244862651328,
-45.2221763702828));
#22525=CARTESIAN_POINT('Ctrl Pts',(-149.894024345238,-81.0222194822742,
-45.2201718089514));
#22526=CARTESIAN_POINT('Ctrl Pts',(-149.901678691384,-80.9934460867894,
-45.194726920949));
#22527=CARTESIAN_POINT('Ctrl Pts',(-149.909127380051,-80.9654260581732,
-45.1685200129132));
#22528=CARTESIAN_POINT('Ctrl Pts',(-149.916327644768,-80.9383234966228,
-45.1414142231911));
#22529=CARTESIAN_POINT('Ctrl Pts',(-149.922896825408,-80.9135964026004,
-45.1166841839377));
#22530=CARTESIAN_POINT('Ctrl Pts',(-149.929259164437,-80.8896331987158,
-45.0912058787197));
#22531=CARTESIAN_POINT('Ctrl Pts',(-149.935369835439,-80.8666055523403,
-45.0648643182037));
#22532=CARTESIAN_POINT('Ctrl Pts',(-149.935956871689,-80.864393346322,-45.0623337530841));
#22533=CARTESIAN_POINT('Ctrl Pts',(-149.936541575424,-80.8621898122599,
-45.0597952121657));
#22534=CARTESIAN_POINT('Ctrl Pts',(-149.937123900464,-80.8599951269442,
-45.0572485877254));
#22535=CARTESIAN_POINT('Ctrl Pts',(-149.949888621083,-80.8118870379003,
-45.0014258989527));
#22536=CARTESIAN_POINT('Ctrl Pts',(-149.961572072671,-80.7677918263995,
-44.9414473167645));
#22537=CARTESIAN_POINT('Ctrl Pts',(-149.971367310254,-80.7307169524392,
-44.8772845402088));
#22538=CARTESIAN_POINT('Ctrl Pts',(-149.975158206732,-80.7163684480826,
-44.8524526316788));
#22539=CARTESIAN_POINT('Ctrl Pts',(-149.978650998302,-80.7031305919437,
-44.8269091212123));
#22540=CARTESIAN_POINT('Ctrl Pts',(-149.981796037926,-80.6911891223571,
-44.8007713404859));
#22541=CARTESIAN_POINT('Ctrl Pts',(-149.985757876155,-80.6761463323222,
-44.767845313702));
#22542=CARTESIAN_POINT('Ctrl Pts',(-149.989179977686,-80.6631984113658,
-44.7338784466372));
#22543=CARTESIAN_POINT('Ctrl Pts',(-149.991954976262,-80.6527310533633,
-44.6991041970813));
#22544=CARTESIAN_POINT('Ctrl Pts',(-149.993127423005,-80.6483085574693,
-44.6844119532658));
#22545=CARTESIAN_POINT('Ctrl Pts',(-149.994184300917,-80.6443291875704,
-44.669576131169));
#22546=CARTESIAN_POINT('Ctrl Pts',(-149.995117265699,-80.6408234431072,
-44.6546167402297));
#22547=CARTESIAN_POINT('Ctrl Pts',(-149.997168971269,-80.6331138750976,
-44.6217191793725));
#22548=CARTESIAN_POINT('Ctrl Pts',(-149.998622294847,-80.62769656615,-44.5882207958789));
#22549=CARTESIAN_POINT('Ctrl Pts',(-149.999384955835,-80.6248606269888,
-44.5543174102316));
#22550=CARTESIAN_POINT('Ctrl Pts',(-149.999789923498,-80.6233547630872,
-44.5363149490749));
#22551=CARTESIAN_POINT('Ctrl Pts',(-150.,-80.6225774829854,-44.5181985965764));
#22552=CARTESIAN_POINT('Ctrl Pts',(-150.,-80.6225774829854,-44.5));
#22553=CARTESIAN_POINT('Origin',(-147.5,-122.5,-44.5));
#22554=CARTESIAN_POINT('Origin',(0.,0.,-49.5));
#22555=CARTESIAN_POINT('Origin',(-147.5,-89.4427190999916,-49.5));
#22556=CARTESIAN_POINT('Origin',(-177.5,-137.5,-73.9644660940673));
#22557=CARTESIAN_POINT('Origin',(-177.5,-137.5,-73.9644660940673));
#22558=CARTESIAN_POINT('Origin',(-177.5,-137.5,-73.9644660940673));
#22559=CARTESIAN_POINT('Origin',(-177.5,-137.5,-73.9644660940673));
#22560=CARTESIAN_POINT('Origin',(-168.964466094067,-127.5,-82.5));
#22561=CARTESIAN_POINT('Origin',(-168.964466094067,-127.5,-82.5));
#22562=CARTESIAN_POINT('Origin',(-168.964466094067,-127.5,-82.5));
#22563=CARTESIAN_POINT('Origin',(-168.964466094067,-127.5,-82.5));
#22564=CARTESIAN_POINT('Origin',(-147.5,-122.5,-44.5));
#22565=CARTESIAN_POINT('Origin',(-152.5,-122.5,-44.5));
#22566=CARTESIAN_POINT('Ctrl Pts',(-145.36231884058,-88.1464478086873,-49.5));
#22567=CARTESIAN_POINT('Ctrl Pts',(-145.36231884058,-88.1464478086873,-47.));
#22568=CARTESIAN_POINT('Ctrl Pts',(-147.5,-89.4427190999916,-47.));
#22569=CARTESIAN_POINT('Ctrl Pts',(-145.88328041902,-87.2873300001825,-49.4999999990697));
#22570=CARTESIAN_POINT('Ctrl Pts',(-145.793011707092,-87.4361921450511,
-47.2163561992337));
#22571=CARTESIAN_POINT('Ctrl Pts',(-147.764311380887,-88.5709672327986,
-47.));
#22572=CARTESIAN_POINT('Ctrl Pts',(-146.390924783419,-86.432995377738,-49.4182529717019));
#22573=CARTESIAN_POINT('Ctrl Pts',(-146.25636627112,-86.6602829701382,-47.3466184200069));
#22574=CARTESIAN_POINT('Ctrl Pts',(-148.021866250329,-87.7040688391623,
-46.959126485635));
#22575=CARTESIAN_POINT('Ctrl Pts',(-147.13295559207,-85.1594666843921,-49.1735002410464));
#22576=CARTESIAN_POINT('Ctrl Pts',(-146.95625485105,-85.4644664729224,-47.393964945865));
#22577=CARTESIAN_POINT('Ctrl Pts',(-148.398337763665,-86.4118117826985,
-46.8367501206312));
#22578=CARTESIAN_POINT('Ctrl Pts',(-147.377049426154,-84.7363019818542,
-49.0712223542218));
#22579=CARTESIAN_POINT('Ctrl Pts',(-147.185340564392,-85.0695699101127,
-47.3871528892726));
#22580=CARTESIAN_POINT('Ctrl Pts',(-148.522179488132,-85.9824240698147,
-46.7856111768689));
#22581=CARTESIAN_POINT('Ctrl Pts',(-147.858493843555,-83.8933928830767,
-48.8197197604928));
#22582=CARTESIAN_POINT('Ctrl Pts',(-147.640340054158,-84.2776371924664,
-47.3236601563046));
#22583=CARTESIAN_POINT('Ctrl Pts',(-148.766441729588,-85.1271192490123,
-46.6598598804885));
#22584=CARTESIAN_POINT('Ctrl Pts',(-148.095887496716,-83.4735259621086,
-48.670309617217));
#22585=CARTESIAN_POINT('Ctrl Pts',(-147.866955151253,-83.8795640251351,
-47.2682201155608));
#22586=CARTESIAN_POINT('Ctrl Pts',(-148.886884097334,-84.7010778144719,
-46.5851548082849));
#22587=CARTESIAN_POINT('Ctrl Pts',(-148.555727425865,-82.65238822296,-48.3190668315844));
#22588=CARTESIAN_POINT('Ctrl Pts',(-148.307824862021,-83.0977615436487,
-47.1034791582529));
#22589=CARTESIAN_POINT('Ctrl Pts',(-149.120185238387,-83.867864520377,-46.4095334161157));
#22590=CARTESIAN_POINT('Ctrl Pts',(-148.780093861296,-82.2476812683581,
-48.1160600755383));
#22591=CARTESIAN_POINT('Ctrl Pts',(-148.524727773055,-82.7095240936236,
-46.9949635047617));
#22592=CARTESIAN_POINT('Ctrl Pts',(-149.234018208522,-83.457205992854,-46.308030037322));
#22593=CARTESIAN_POINT('Ctrl Pts',(-149.207972890121,-81.4688789012013,
-47.6426010624872));
#22594=CARTESIAN_POINT('Ctrl Pts',(-148.93931728545,-81.9607628458225,-46.713912421055));
#22595=CARTESIAN_POINT('Ctrl Pts',(-149.4511038933,-82.6669506497871,-46.0713005316908));
#22596=CARTESIAN_POINT('Ctrl Pts',(-149.410469407752,-81.0966396786721,
-47.3745618678272));
#22597=CARTESIAN_POINT('Ctrl Pts',(-149.13707735126,-81.6002642788733,-46.5440613352092));
#22598=CARTESIAN_POINT('Ctrl Pts',(-149.553841095111,-82.2892373209608,
-45.9372809330665));
#22599=CARTESIAN_POINT('Ctrl Pts',(-149.689478100498,-80.5797647052593,
-46.8989514695024));
#22600=CARTESIAN_POINT('Ctrl Pts',(-149.410828634125,-81.0973762069276,
-46.2235340082297));
#22601=CARTESIAN_POINT('Ctrl Pts',(-149.695396978193,-81.7647612450649,
-45.6994757351747));
#22602=CARTESIAN_POINT('Ctrl Pts',(-149.778860900691,-80.4134491496535,
-46.7265495064604));
#22603=CARTESIAN_POINT('Ctrl Pts',(-149.498351131341,-80.935915280146,-46.1055106385897));
#22604=CARTESIAN_POINT('Ctrl Pts',(-149.74074560314,-81.5959998724055,-45.6132747528471));
#22605=CARTESIAN_POINT('Ctrl Pts',(-149.942345818684,-80.1081950067706,
-46.3555706163427));
#22606=CARTESIAN_POINT('Ctrl Pts',(-149.658443692203,-80.6395711160542,
-45.8467452989258));
#22607=CARTESIAN_POINT('Ctrl Pts',(-149.823690158896,-81.2862566980837,
-45.4277853085544));
#22608=CARTESIAN_POINT('Ctrl Pts',(-150.016754772459,-79.9686937648418,
-46.1569684467915));
#22609=CARTESIAN_POINT('Ctrl Pts',(-149.731542660712,-80.5037270542566,
-45.7060159661836));
#22610=CARTESIAN_POINT('Ctrl Pts',(-149.861441758745,-81.144703967216,-45.3284842231662));
#22611=CARTESIAN_POINT('Ctrl Pts',(-150.145196691125,-79.7272764209246,
-45.7237173672864));
#22612=CARTESIAN_POINT('Ctrl Pts',(-149.857607243134,-80.2688649285009,
-45.3951674418671));
#22613=CARTESIAN_POINT('Ctrl Pts',(-149.926607145573,-80.8997363683411,
-45.1118586838727));
#22614=CARTESIAN_POINT('Ctrl Pts',(-150.197080555724,-79.6294105444985,
-45.4961190800877));
#22615=CARTESIAN_POINT('Ctrl Pts',(-149.908727602392,-80.1732994372084,
-45.2298837812697));
#22616=CARTESIAN_POINT('Ctrl Pts',(-149.952930574586,-80.8004312877628,
-44.9980595398227));
#22617=CARTESIAN_POINT('Ctrl Pts',(-150.269771338359,-79.4921496315481,
-45.0129350155497));
#22618=CARTESIAN_POINT('Ctrl Pts',(-149.980179574577,-80.0395829024242,
-44.8770900280323));
#22619=CARTESIAN_POINT('Ctrl Pts',(-149.989810459912,-80.6611518320492,
-44.756467507996));
#22620=CARTESIAN_POINT('Ctrl Pts',(-150.289855071895,-79.4541343321333,
-44.7534294495147));
#22621=CARTESIAN_POINT('Ctrl Pts',(-149.99999999943,-80.0024038110911,-44.686188272212));
#22622=CARTESIAN_POINT('Ctrl Pts',(-150.,-80.6225774840775,-44.6267147245865));
#22623=CARTESIAN_POINT('Ctrl Pts',(-150.289855072464,-79.4541343310581,
-44.5));
#22624=CARTESIAN_POINT('Ctrl Pts',(-150.,-80.0024038100394,-44.5));
#22625=CARTESIAN_POINT('Ctrl Pts',(-150.,-80.6225774829855,-44.5));
#22626=CARTESIAN_POINT('Origin',(-152.5,-80.6225774829854,-44.5));
#22627=CARTESIAN_POINT('Origin',(-121.449578014911,-122.5,115.));
#22628=CARTESIAN_POINT('Origin',(-121.449578014911,-122.5,-82.5));
#22629=CARTESIAN_POINT('Origin',(-115.217186218029,-127.5,-82.5));
#22630=CARTESIAN_POINT('Ctrl Pts',(-116.189500386223,-127.5,-85.));
#22631=CARTESIAN_POINT('Ctrl Pts',(-116.448008540164,-127.38221202645,-85.));
#22632=CARTESIAN_POINT('Ctrl Pts',(-116.705458596259,-127.264170864129,
-84.9919054816514));
#22633=CARTESIAN_POINT('Ctrl Pts',(-116.961798715611,-127.145925914751,
-84.9750282599707));
#22634=CARTESIAN_POINT('Ctrl Pts',(-117.203993378032,-127.034206002666,
-84.959082363488));
#22635=CARTESIAN_POINT('Ctrl Pts',(-117.44519709589,-126.922304462312,-84.9352961056291));
#22636=CARTESIAN_POINT('Ctrl Pts',(-117.685352831461,-126.810270252905,
-84.9030396156349));
#22637=CARTESIAN_POINT('Ctrl Pts',(-117.699379204216,-126.803726858975,
-84.901155664992));
#22638=CARTESIAN_POINT('Ctrl Pts',(-117.713401998462,-126.797183013924,
-84.8992428065339));
#22639=CARTESIAN_POINT('Ctrl Pts',(-117.727421201482,-126.790638727993,
-84.8973009093819));
#22640=CARTESIAN_POINT('Ctrl Pts',(-117.801716706967,-126.755956939694,
-84.8870097230497));
#22641=CARTESIAN_POINT('Ctrl Pts',(-117.875811770812,-126.72130622253,-84.8759163529927));
#22642=CARTESIAN_POINT('Ctrl Pts',(-117.949766484241,-126.686659174449,
-84.8639959183808));
#22643=CARTESIAN_POINT('Ctrl Pts',(-118.068035959454,-126.631251100991,
-84.8449325824487));
#22644=CARTESIAN_POINT('Ctrl Pts',(-118.186129688152,-126.575765453047,
-84.8236742085077));
#22645=CARTESIAN_POINT('Ctrl Pts',(-118.304009972751,-126.520223268687,
-84.8000156545));
#22646=CARTESIAN_POINT('Ctrl Pts',(-118.414673338124,-126.468081512646,
-84.7778055350109));
#22647=CARTESIAN_POINT('Ctrl Pts',(-118.525149041405,-126.415889691706,
-84.7534800370882));
#22648=CARTESIAN_POINT('Ctrl Pts',(-118.635381578983,-126.363674712058,
-84.7268318519906));
#22649=CARTESIAN_POINT('Ctrl Pts',(-118.688420413233,-126.338551262016,
-84.7140099692372));
#22650=CARTESIAN_POINT('Ctrl Pts',(-118.741402540235,-126.313422617281,
-84.7006497952816));
#22651=CARTESIAN_POINT('Ctrl Pts',(-118.794319125547,-126.288292874884,
-84.6867249125821));
#22652=CARTESIAN_POINT('Ctrl Pts',(-118.89901828691,-126.238571923717,-84.6591735592185));
#22653=CARTESIAN_POINT('Ctrl Pts',(-119.002876811888,-126.18912499207,-84.6295858023532));
#22654=CARTESIAN_POINT('Ctrl Pts',(-119.105920148863,-126.139946013055,
-84.5977086876026));
#22655=CARTESIAN_POINT('Ctrl Pts',(-119.148229575834,-126.119753204066,
-84.5846199960073));
#22656=CARTESIAN_POINT('Ctrl Pts',(-119.190401214652,-126.099605728962,
-84.5711448947655));
#22657=CARTESIAN_POINT('Ctrl Pts',(-119.232435280194,-126.079503870074,
-84.5572639252337));
#22658=CARTESIAN_POINT('Ctrl Pts',(-119.332253758365,-126.031767898387,
-84.5243007265441));
#22659=CARTESIAN_POINT('Ctrl Pts',(-119.431308801215,-125.984284516973,
-84.4890488616581));
#22660=CARTESIAN_POINT('Ctrl Pts',(-119.529560384293,-125.937075343597,
-84.4512249355449));
#22661=CARTESIAN_POINT('Ctrl Pts',(-119.549179492618,-125.927648504279,
-84.4436721645821));
#22662=CARTESIAN_POINT('Ctrl Pts',(-119.568766466804,-125.918232645452,
-84.4360167122206));
#22663=CARTESIAN_POINT('Ctrl Pts',(-119.588320838716,-125.908828011419,
-84.4282561299978));
#22664=CARTESIAN_POINT('Ctrl Pts',(-119.676176605187,-125.866573965367,
-84.3933886383424));
#22665=CARTESIAN_POINT('Ctrl Pts',(-119.763367641033,-125.824549754932,
-84.3563903280335));
#22666=CARTESIAN_POINT('Ctrl Pts',(-119.849778269352,-125.78281394182,-84.3169432874789));
#22667=CARTESIAN_POINT('Ctrl Pts',(-119.884154184046,-125.766210582034,
-84.3012504482132));
#22668=CARTESIAN_POINT('Ctrl Pts',(-119.918406261835,-125.749653027024,
-84.285169643908));
#22669=CARTESIAN_POINT('Ctrl Pts',(-119.952525858354,-125.73314564101,-84.2686790921246));
#22670=CARTESIAN_POINT('Ctrl Pts',(-119.954356344091,-125.732260034563,
-84.2677943888192));
#22671=CARTESIAN_POINT('Ctrl Pts',(-119.956186462171,-125.731374563089,
-84.2669084964012));
#22672=CARTESIAN_POINT('Ctrl Pts',(-119.95801621397,-125.730489226021,-84.2660214100551));
#22673=CARTESIAN_POINT('Ctrl Pts',(-120.016911873287,-125.701992185948,
-84.2374680645811));
#22674=CARTESIAN_POINT('Ctrl Pts',(-120.075514267379,-125.673592123274,
-84.2076160589801));
#22675=CARTESIAN_POINT('Ctrl Pts',(-120.133520234545,-125.645440552611,
-84.1764738678679));
#22676=CARTESIAN_POINT('Ctrl Pts',(-120.185326529737,-125.620297819008,
-84.1486601510297));
#22677=CARTESIAN_POINT('Ctrl Pts',(-120.236657062529,-125.59535329509,-84.1198170380798));
#22678=CARTESIAN_POINT('Ctrl Pts',(-120.287252932554,-125.570735521226,
-84.0899486389992));
#22679=CARTESIAN_POINT('Ctrl Pts',(-120.293307752653,-125.567789506227,
-84.0863742804003));
#22680=CARTESIAN_POINT('Ctrl Pts',(-120.299351995995,-125.564848197422,
-84.0827852386968));
#22681=CARTESIAN_POINT('Ctrl Pts',(-120.305385171906,-125.561911837745,
-84.079181521328));
#22682=CARTESIAN_POINT('Ctrl Pts',(-120.360569807383,-125.535053357107,
-84.0462188110888));
#22683=CARTESIAN_POINT('Ctrl Pts',(-120.414989618108,-125.50853101205,-84.0119891408405));
#22684=CARTESIAN_POINT('Ctrl Pts',(-120.468555276039,-125.482393019766,
-83.9762964268604));
#22685=CARTESIAN_POINT('Ctrl Pts',(-120.521845432248,-125.456389461785,
-83.9407872895329));
#22686=CARTESIAN_POINT('Ctrl Pts',(-120.574290544884,-125.430766130918,
-83.9038303719348));
#22687=CARTESIAN_POINT('Ctrl Pts',(-120.625763505242,-125.405589684656,
-83.8652058122217));
#22688=CARTESIAN_POINT('Ctrl Pts',(-120.669724343266,-125.384087566487,
-83.8322182396883));
#22689=CARTESIAN_POINT('Ctrl Pts',(-120.712919977839,-125.362939699074,
-83.7980586074073));
#22690=CARTESIAN_POINT('Ctrl Pts',(-120.755308589257,-125.342167431334,
-83.7625256624013));
#22691=CARTESIAN_POINT('Ctrl Pts',(-120.796119057648,-125.322168522485,
-83.7283156215319));
#22692=CARTESIAN_POINT('Ctrl Pts',(-120.836181594647,-125.302517695472,
-83.6928327066298));
#22693=CARTESIAN_POINT('Ctrl Pts',(-120.875421453446,-125.283252598417,
-83.6558720771509));
#22694=CARTESIAN_POINT('Ctrl Pts',(-120.882694505649,-125.279681839988,
-83.6490214768709));
#22695=CARTESIAN_POINT('Ctrl Pts',(-120.889939185328,-125.276124387981,
-83.6421200366566));
#22696=CARTESIAN_POINT('Ctrl Pts',(-120.897154862446,-125.27258055919,-83.6351663481079));
#22697=CARTESIAN_POINT('Ctrl Pts',(-120.930420737934,-125.256242720708,
-83.6031082981616));
#22698=CARTESIAN_POINT('Ctrl Pts',(-120.96296989403,-125.240243618619,-83.5699873691134));
#22699=CARTESIAN_POINT('Ctrl Pts',(-120.994602600046,-125.224682872272,
-83.5357995420531));
#22700=CARTESIAN_POINT('Ctrl Pts',(-121.02464265881,-125.209905580236,-83.5033330077842));
#22701=CARTESIAN_POINT('Ctrl Pts',(-121.053856347371,-125.195523551208,
-83.4699041219391));
#22702=CARTESIAN_POINT('Ctrl Pts',(-121.082031519278,-125.18164267959,-83.4355171689384));
#22703=CARTESIAN_POINT('Ctrl Pts',(-121.097985602238,-125.173782689309,
-83.416045688775));
#22704=CARTESIAN_POINT('Ctrl Pts',(-121.11360593729,-125.166083770046,-83.3962671746067));
#22705=CARTESIAN_POINT('Ctrl Pts',(-121.128847427401,-125.158568448299,
-83.376183935507));
#22706=CARTESIAN_POINT('Ctrl Pts',(-121.149706220237,-125.148283329307,
-83.3486989507179));
#22707=CARTESIAN_POINT('Ctrl Pts',(-121.169911626187,-125.138314491271,
-83.3205937206655));
#22708=CARTESIAN_POINT('Ctrl Pts',(-121.189383694811,-125.128702127376,
-83.2918112814196));
#22709=CARTESIAN_POINT('Ctrl Pts',(-121.219288926774,-125.113939444605,
-83.247607168403));
#22710=CARTESIAN_POINT('Ctrl Pts',(-121.247502565948,-125.100002690926,
-83.2017508061736));
#22711=CARTESIAN_POINT('Ctrl Pts',(-121.273533474804,-125.08713705477,-83.1542957064863));
#22712=CARTESIAN_POINT('Ctrl Pts',(-121.283706281802,-125.082109199836,
-83.135750385119));
#22713=CARTESIAN_POINT('Ctrl Pts',(-121.293546196394,-125.077244718342,
-83.1169610513985));
#22714=CARTESIAN_POINT('Ctrl Pts',(-121.303025858184,-125.072557339689,
-83.0979315436974));
#22715=CARTESIAN_POINT('Ctrl Pts',(-121.323095906427,-125.06263336584,-83.0576428555519));
#22716=CARTESIAN_POINT('Ctrl Pts',(-121.34152898982,-125.053514201558,-83.0161861526794));
#22717=CARTESIAN_POINT('Ctrl Pts',(-121.357996565739,-125.045363893213,
-82.973949637818));
#22718=CARTESIAN_POINT('Ctrl Pts',(-121.365145493274,-125.041825669735,
-82.9556138617733));
#22719=CARTESIAN_POINT('Ctrl Pts',(-121.371924242056,-125.038469923384,
-82.9371317587527));
#22720=CARTESIAN_POINT('Ctrl Pts',(-121.378307256223,-125.035309443556,
-82.9185377169621));
#22721=CARTESIAN_POINT('Ctrl Pts',(-121.391447468896,-125.028803210607,
-82.8802596155573));
#22722=CARTESIAN_POINT('Ctrl Pts',(-121.402999576331,-125.02308111907,-82.841245154545));
#22723=CARTESIAN_POINT('Ctrl Pts',(-121.41267276749,-125.018288884737,-82.8018442319799));
#22724=CARTESIAN_POINT('Ctrl Pts',(-121.42270975789,-125.013316419167,-82.7609614793284));
#22725=CARTESIAN_POINT('Ctrl Pts',(-121.430817047126,-125.009299023436,
-82.7195176677953));
#22726=CARTESIAN_POINT('Ctrl Pts',(-121.436839100795,-125.006314500192,
-82.677630304934));
#22727=CARTESIAN_POINT('Ctrl Pts',(-121.442766130955,-125.003377070495,
-82.6364038933766));
#22728=CARTESIAN_POINT('Ctrl Pts',(-121.446673152346,-125.00144020774,-82.5947478149961));
#22729=CARTESIAN_POINT('Ctrl Pts',(-121.448457146611,-125.00055573514,-82.5527767556245));
#22730=CARTESIAN_POINT('Ctrl Pts',(-121.449202695036,-125.000186105502,
-82.5352366447455));
#22731=CARTESIAN_POINT('Ctrl Pts',(-121.449578014744,-125.,-82.5176415553729));
#22732=CARTESIAN_POINT('Ctrl Pts',(-121.449578014911,-125.,-82.5));
#22733=CARTESIAN_POINT('Origin',(-168.964466094067,0.,-82.5));
#22734=CARTESIAN_POINT('Origin',(-168.964466094067,-137.5,-82.5));
#22735=CARTESIAN_POINT('Origin',(-258.232233047034,-137.5,6.76776695296637));
#22736=CARTESIAN_POINT('Origin',(-168.964466094067,-137.5,-82.5));
#22737=CARTESIAN_POINT('Origin',(-177.5,-137.5,85.));
#22738=CARTESIAN_POINT('Origin',(-177.5,-137.5,73.9644660940671));
#22739=CARTESIAN_POINT('Origin',(-177.5,-125.,-73.9644660940673));
#22740=CARTESIAN_POINT('Origin',(-177.5,-127.5,-73.9644660940673));
#22741=CARTESIAN_POINT('Origin',(-225.840826156048,-127.5,-25.6236399380191));
#22742=CARTESIAN_POINT('Origin',(-177.5,-127.5,-73.9644660940673));
#22743=CARTESIAN_POINT('Origin',(-152.5,-122.5,-47.));
#22744=CARTESIAN_POINT('Origin',(-152.5,-122.5,-37.5));
#22745=CARTESIAN_POINT('Origin',(-147.5,0.,-37.5));
#22746=CARTESIAN_POINT('Ctrl Pts',(-150.,-80.6225774829854,-37.5));
#22747=CARTESIAN_POINT('Ctrl Pts',(-150.,-80.6225774829854,-37.4687656111694));
#22748=CARTESIAN_POINT('Ctrl Pts',(-149.999418286665,-80.6247797743348,
-37.4378789835208));
#22749=CARTESIAN_POINT('Ctrl Pts',(-149.998293554945,-80.6290354954266,
-37.407427664437));
#22750=CARTESIAN_POINT('Ctrl Pts',(-149.997125538082,-80.6334549973543,
-37.3758044305615));
#22751=CARTESIAN_POINT('Ctrl Pts',(-149.995371936956,-80.6400888791783,
-37.3446506435411));
#22752=CARTESIAN_POINT('Ctrl Pts',(-149.993090530187,-80.6487160556982,
-37.3140587875661));
#22753=CARTESIAN_POINT('Ctrl Pts',(-149.992231155702,-80.6519657941863,
-37.3025352570627));
#22754=CARTESIAN_POINT('Ctrl Pts',(-149.991297028852,-80.6554978429528,
-37.2910914065902));
#22755=CARTESIAN_POINT('Ctrl Pts',(-149.990291719683,-80.6592985775913,
-37.2797319931106));
#22756=CARTESIAN_POINT('Ctrl Pts',(-149.987499102739,-80.6698565196466,
-37.2481770331612));
#22757=CARTESIAN_POINT('Ctrl Pts',(-149.984157100677,-80.6824881297729,
-37.2172858271412));
#22758=CARTESIAN_POINT('Ctrl Pts',(-149.980355786964,-80.6968505802923,
-37.1871743733059));
#22759=CARTESIAN_POINT('Ctrl Pts',(-149.977558137322,-80.7074209008703,
-37.1650132720595));
#22760=CARTESIAN_POINT('Ctrl Pts',(-149.974509955706,-80.7189351701335,
-37.1432550493073));
#22761=CARTESIAN_POINT('Ctrl Pts',(-149.971243495187,-80.7312708109916,
-37.1219053194033));
#22762=CARTESIAN_POINT('Ctrl Pts',(-149.965898079906,-80.7514575307658,
-37.0869674495522));
#22763=CARTESIAN_POINT('Ctrl Pts',(-149.960009186175,-80.7736866486582,
-37.0534295032029));
#22764=CARTESIAN_POINT('Ctrl Pts',(-149.953740444396,-80.7973352935883,
-37.0212984263663));
#22765=CARTESIAN_POINT('Ctrl Pts',(-149.948225014273,-80.8181420923422,
-36.9930285254284));
#22766=CARTESIAN_POINT('Ctrl Pts',(-149.942415420697,-80.8400482471093,
-36.9658474797142));
#22767=CARTESIAN_POINT('Ctrl Pts',(-149.936415096464,-80.8626613647233,
-36.9397533647229));
#22768=CARTESIAN_POINT('Ctrl Pts',(-149.930229230798,-80.8859737229203,
-36.9128523700925));
#22769=CARTESIAN_POINT('Ctrl Pts',(-149.923781601043,-80.910257863373,-36.8868469814865));
#22770=CARTESIAN_POINT('Ctrl Pts',(-149.917129634266,-80.9352949903568,
-36.8616578829437));
#22771=CARTESIAN_POINT('Ctrl Pts',(-149.910169623637,-80.9614915538333,
-36.8353023103049));
#22772=CARTESIAN_POINT('Ctrl Pts',(-149.902985851618,-80.9885126935554,
-36.8098403335372));
#22773=CARTESIAN_POINT('Ctrl Pts',(-149.895629953762,-81.0161619977779,
-36.7851874043746));
#22774=CARTESIAN_POINT('Ctrl Pts',(-149.894768894783,-81.0193985410422,
-36.7823016076404));
#22775=CARTESIAN_POINT('Ctrl Pts',(-149.893905462669,-81.0226437476004,
-36.7794269040105));
#22776=CARTESIAN_POINT('Ctrl Pts',(-149.893039728921,-81.0258973457803,
-36.776563163654));
#22777=CARTESIAN_POINT('Ctrl Pts',(-149.885294621978,-81.0550049852878,
-36.7509433060895));
#22778=CARTESIAN_POINT('Ctrl Pts',(-149.877335285321,-81.0848961910516,
-36.7261125791003));
#22779=CARTESIAN_POINT('Ctrl Pts',(-149.869211724908,-81.1153826082327,
-36.7020057411971));
#22780=CARTESIAN_POINT('Ctrl Pts',(-149.860756318488,-81.1471143901678,
-36.6769141432259));
#22781=CARTESIAN_POINT('Ctrl Pts',(-149.852122886993,-81.1794914281188,
-36.652606677046));
#22782=CARTESIAN_POINT('Ctrl Pts',(-149.843353240434,-81.2123567796228,
-36.6290138576759));
#22783=CARTESIAN_POINT('Ctrl Pts',(-149.83403385977,-81.2472823286997,-36.603942098724));
#22784=CARTESIAN_POINT('Ctrl Pts',(-149.824560562648,-81.2827596738303,
-36.5796772330309));
#22785=CARTESIAN_POINT('Ctrl Pts',(-149.814968902627,-81.3186560160361,
-36.5561425173624));
#22786=CARTESIAN_POINT('Ctrl Pts',(-149.814245534129,-81.3213631890505,
-36.5543676137582));
#22787=CARTESIAN_POINT('Ctrl Pts',(-149.813521486333,-81.3240727682797,
-36.5525968666158));
#22788=CARTESIAN_POINT('Ctrl Pts',(-149.812796771609,-81.3267847076915,
-36.550830244838));
#22789=CARTESIAN_POINT('Ctrl Pts',(-149.802161746897,-81.3665818053883,
-36.5249054696828));
#22790=CARTESIAN_POINT('Ctrl Pts',(-149.791378236576,-81.4068954418299,
-36.4998550500824));
#22791=CARTESIAN_POINT('Ctrl Pts',(-149.780505488345,-81.4474999785173,
-36.4756491236568));
#22792=CARTESIAN_POINT('Ctrl Pts',(-149.766212096435,-81.5008789903243,
-36.4438278411627));
#22793=CARTESIAN_POINT('Ctrl Pts',(-149.751731044149,-81.5548874755392,
-36.4133414348064));
#22794=CARTESIAN_POINT('Ctrl Pts',(-149.737090172798,-81.6094178533142,
-36.3839845210638));
#22795=CARTESIAN_POINT('Ctrl Pts',(-149.721679195216,-81.6668165155451,
-36.3530834408805));
#22796=CARTESIAN_POINT('Ctrl Pts',(-149.706091100879,-81.7247936014414,
-36.3234339148103));
#22797=CARTESIAN_POINT('Ctrl Pts',(-149.69034564287,-81.7832715017069,-36.2948268672517));
#22798=CARTESIAN_POINT('Ctrl Pts',(-149.684002656686,-81.8068290580035,
-36.2833026481829));
#22799=CARTESIAN_POINT('Ctrl Pts',(-149.677633997879,-81.8304683944444,
-36.2719479292499));
#22800=CARTESIAN_POINT('Ctrl Pts',(-149.671240444102,-81.8541863565932,
-36.2607502650746));
#22801=CARTESIAN_POINT('Ctrl Pts',(-149.663115656512,-81.8843266214972,
-36.2465205196002));
#22802=CARTESIAN_POINT('Ctrl Pts',(-149.654955183208,-81.9145791058626,
-36.2325522508595));
#22803=CARTESIAN_POINT('Ctrl Pts',(-149.646761444289,-81.9449339838539,
-36.2188226892616));
#22804=CARTESIAN_POINT('Ctrl Pts',(-149.629599044992,-82.0085145472293,
-36.1900650951265));
#22805=CARTESIAN_POINT('Ctrl Pts',(-149.612256027534,-82.0726719053156,
-36.1623178493706));
#22806=CARTESIAN_POINT('Ctrl Pts',(-149.594776281631,-82.1372383448625,
-36.1354843277007));
#22807=CARTESIAN_POINT('Ctrl Pts',(-149.575926055091,-82.2068670465097,
-36.1065469526865));
#22808=CARTESIAN_POINT('Ctrl Pts',(-149.556916727561,-82.2769718986875,
-36.0786720183562));
#22809=CARTESIAN_POINT('Ctrl Pts',(-149.537787182936,-82.3473991049003,
-36.0517539381258));
#22810=CARTESIAN_POINT('Ctrl Pts',(-149.532245072395,-82.3678029027717,
-36.0439553742236));
#22811=CARTESIAN_POINT('Ctrl Pts',(-149.52669278014,-82.3882340721045,-36.0362372267143));
#22812=CARTESIAN_POINT('Ctrl Pts',(-149.521131044556,-82.4086895813365,
-36.0285971804472));
#22813=CARTESIAN_POINT('Ctrl Pts',(-149.513307047731,-82.4374654619681,
-36.0178495106185));
#22814=CARTESIAN_POINT('Ctrl Pts',(-149.505462657807,-82.4662967316409,
-36.007254069327));
#22815=CARTESIAN_POINT('Ctrl Pts',(-149.497602582525,-82.4951656238998,
-35.9968087539204));
#22816=CARTESIAN_POINT('Ctrl Pts',(-149.466886299756,-82.6079819807508,
-35.955989645942));
#22817=CARTESIAN_POINT('Ctrl Pts',(-149.435949796466,-82.7213062383942,
-35.9174537341956));
#22818=CARTESIAN_POINT('Ctrl Pts',(-149.404819096582,-82.8350358340491,
-35.8808341284359));
#22819=CARTESIAN_POINT('Ctrl Pts',(-149.382928718802,-82.9150078174297,
-35.855084080822));
#22820=CARTESIAN_POINT('Ctrl Pts',(-149.360942099018,-82.9951810078626,
-35.8302825444958));
#22821=CARTESIAN_POINT('Ctrl Pts',(-149.338865605393,-83.0755291035975,
-35.8063136992629));
#22822=CARTESIAN_POINT('Ctrl Pts',(-149.302572702508,-83.2076182697917,
-35.7669098434218));
#22823=CARTESIAN_POINT('Ctrl Pts',(-149.266041574135,-83.340162369254,-35.7297345827364));
#22824=CARTESIAN_POINT('Ctrl Pts',(-149.229255373732,-83.4732146574342,
-35.6944829487595));
#22825=CARTESIAN_POINT('Ctrl Pts',(-149.222100057111,-83.4990947765716,
-35.6876261220217));
#22826=CARTESIAN_POINT('Ctrl Pts',(-149.214935059984,-83.5249942184477,
-35.6808421975269));
#22827=CARTESIAN_POINT('Ctrl Pts',(-149.207760216038,-83.550913508967,-35.674129103287));
#22828=CARTESIAN_POINT('Ctrl Pts',(-149.164019348341,-83.7089284101932,
-35.6332032560904));
#22829=CARTESIAN_POINT('Ctrl Pts',(-149.119950314828,-83.8675446159095,
-35.5949411222395));
#22830=CARTESIAN_POINT('Ctrl Pts',(-149.075578120357,-84.0266555942609,
-35.5589506769715));
#22831=CARTESIAN_POINT('Ctrl Pts',(-149.05085132556,-84.1153215833694,-35.5388946854792));
#22832=CARTESIAN_POINT('Ctrl Pts',(-149.026030206994,-84.2041418314535,
-35.5195449132868));
#22833=CARTESIAN_POINT('Ctrl Pts',(-149.001117827171,-84.2931021083258,
-35.5008388586839));
#22834=CARTESIAN_POINT('Ctrl Pts',(-148.961812515426,-84.4334584869733,
-35.4713255278453));
#22835=CARTESIAN_POINT('Ctrl Pts',(-148.922228706232,-84.5743409203764,
-35.4434175359833));
#22836=CARTESIAN_POINT('Ctrl Pts',(-148.882458149794,-84.7154243069166,
-35.4170237357497));
#22837=CARTESIAN_POINT('Ctrl Pts',(-148.823378479995,-84.9250054804708,
-35.3778154082267));
#22838=CARTESIAN_POINT('Ctrl Pts',(-148.763691428328,-85.1357176967391,
-35.3418193924504));
#22839=CARTESIAN_POINT('Ctrl Pts',(-148.703725142255,-85.3463732564986,
-35.3088731061832));
#22840=CARTESIAN_POINT('Ctrl Pts',(-148.683093735184,-85.4188493241311,
-35.2975379329057));
#22841=CARTESIAN_POINT('Ctrl Pts',(-148.662429146897,-85.4913191023785,
-35.2865639616344));
#22842=CARTESIAN_POINT('Ctrl Pts',(-148.64174438629,-85.5637353575988,-35.2759451993142));
#22843=CARTESIAN_POINT('Ctrl Pts',(-148.565624143803,-85.8302283092078,
-35.2368679879267));
#22844=CARTESIAN_POINT('Ctrl Pts',(-148.489028564946,-86.0967324998969,
-35.2024345741108));
#22845=CARTESIAN_POINT('Ctrl Pts',(-148.411875341856,-86.363523818803,-35.1722187734026));
#22846=CARTESIAN_POINT('Ctrl Pts',(-148.365096720872,-86.5252815456893,
-35.1538986899057));
#22847=CARTESIAN_POINT('Ctrl Pts',(-148.318112977961,-86.6871449973961,
-35.137130141918));
#22848=CARTESIAN_POINT('Ctrl Pts',(-148.270904619886,-86.8491769961468,
-35.1218271577707));
#22849=CARTESIAN_POINT('Ctrl Pts',(-148.249186544881,-86.9237193705388,
-35.1147870620957));
#22850=CARTESIAN_POINT('Ctrl Pts',(-148.227421070419,-86.9982969676296,
-35.1080522041554));
#22851=CARTESIAN_POINT('Ctrl Pts',(-148.205605817643,-87.0729174681583,
-35.1016219420906));
#22852=CARTESIAN_POINT('Ctrl Pts',(-148.101900684581,-87.4276476661539,
-35.0710538258322));
#22853=CARTESIAN_POINT('Ctrl Pts',(-147.997167488998,-87.7829762377465,
-35.0474026555606));
#22854=CARTESIAN_POINT('Ctrl Pts',(-147.891499227655,-88.138532391371,-35.0306489702423));
#22855=CARTESIAN_POINT('Ctrl Pts',(-147.78574533598,-88.4943766768485,-35.0138817082488));
#22856=CARTESIAN_POINT('Ctrl Pts',(-147.679054864753,-88.8504488623489,
-35.0040231183754));
#22857=CARTESIAN_POINT('Ctrl Pts',(-147.571529966672,-89.2063722165035,
-35.0010024709468));
#22858=CARTESIAN_POINT('Ctrl Pts',(-147.547727112024,-89.2851631943715,
-35.0003337883163));
#22859=CARTESIAN_POINT('Ctrl Pts',(-147.523883400841,-89.3639468609495,
-35.));
#22860=CARTESIAN_POINT('Ctrl Pts',(-147.5,-89.4427190999916,-35.));
#22861=CARTESIAN_POINT('Origin',(-147.5,-122.5,-37.5));
#22862=CARTESIAN_POINT('Origin',(-152.5,-80.6225774829854,115.));
#22863=CARTESIAN_POINT('Origin',(-152.5,-80.6225774829854,-37.5));
#22864=CARTESIAN_POINT('Ctrl Pts',(-114.505594583524,-125.652173913043,
-87.5));
#22865=CARTESIAN_POINT('Ctrl Pts',(-114.505594583524,-125.652173913043,
-85.));
#22866=CARTESIAN_POINT('Ctrl Pts',(-116.189500386223,-127.5,-85.));
#22867=CARTESIAN_POINT('Ctrl Pts',(-115.098666513068,-125.111713276284,
-87.4999999993277));
#22868=CARTESIAN_POINT('Ctrl Pts',(-114.980468455819,-125.21942600709,-84.7891971375595));
#22869=CARTESIAN_POINT('Ctrl Pts',(-116.791295074217,-127.225795199449,
-85.));
#22870=CARTESIAN_POINT('Ctrl Pts',(-115.677248330335,-124.576762485167,
-87.412213589489));
#22871=CARTESIAN_POINT('Ctrl Pts',(-115.390477170765,-124.841163526192,
-84.4869181320101));
#22872=CARTESIAN_POINT('Ctrl Pts',(-117.378384335172,-126.95438684932,-84.9561067940532));
#22873=CARTESIAN_POINT('Ctrl Pts',(-116.521921487208,-123.785260415244,
-87.135895140949));
#22874=CARTESIAN_POINT('Ctrl Pts',(-115.879476439131,-124.389591527247,
-83.9347335464694));
#22875=CARTESIAN_POINT('Ctrl Pts',(-118.235479156148,-126.552815945855,
-84.8179475708202));
#22876=CARTESIAN_POINT('Ctrl Pts',(-116.800657852351,-123.522253316272,
-87.0187226097842));
#22877=CARTESIAN_POINT('Ctrl Pts',(-116.025791458685,-124.254393807365,
-83.7225655755117));
#22878=CARTESIAN_POINT('Ctrl Pts',(-118.518314585434,-126.419378520878,
-84.759361304629));
#22879=CARTESIAN_POINT('Ctrl Pts',(-117.34468969422,-123.005546784032,-86.7281977784604));
#22880=CARTESIAN_POINT('Ctrl Pts',(-116.260513692639,-124.039299071365,
-83.2680355386611));
#22881=CARTESIAN_POINT('Ctrl Pts',(-119.070346895646,-126.157225941776,
-84.6140988894933));
#22882=CARTESIAN_POINT('Ctrl Pts',(-117.60597211412,-122.755671483611,-86.5572347078813));
#22883=CARTESIAN_POINT('Ctrl Pts',(-116.343854196174,-123.964200078234,
-83.0270891162966));
#22884=CARTESIAN_POINT('Ctrl Pts',(-119.335471703986,-126.03045097373,-84.5286173533875));
#22885=CARTESIAN_POINT('Ctrl Pts',(-117.979759695142,-122.396103662868,
-86.2561620132639));
#22886=CARTESIAN_POINT('Ctrl Pts',(-116.408893575194,-123.910132089278,
-82.6723188019287));
#22887=CARTESIAN_POINT('Ctrl Pts',(-119.714756161271,-125.848023181682,
-84.3780810069086));
#22888=CARTESIAN_POINT('Ctrl Pts',(-118.101314578112,-122.278806587616,
-86.1483179654515));
#22889=CARTESIAN_POINT('Ctrl Pts',(-116.420127652016,-123.902387828605,
-82.5524859464439));
#22890=CARTESIAN_POINT('Ctrl Pts',(-119.838098616001,-125.788512166127,
-84.3241589823631));
#22891=CARTESIAN_POINT('Ctrl Pts',(-118.337674566633,-122.050079163151,
-85.9157683721022));
#22892=CARTESIAN_POINT('Ctrl Pts',(-116.419552940988,-123.909688381786,
-82.3194835992922));
#22893=CARTESIAN_POINT('Ctrl Pts',(-120.077934486754,-125.672466633894,
-84.2078841864137));
#22894=CARTESIAN_POINT('Ctrl Pts',(-118.452813811182,-121.938320691335,
-85.7905474845089));
#22895=CARTESIAN_POINT('Ctrl Pts',(-116.406751222323,-123.925725220726,
-82.2063383456552));
#22896=CARTESIAN_POINT('Ctrl Pts',(-120.194766955425,-125.615765645109,
-84.1452737420412));
#22897=CARTESIAN_POINT('Ctrl Pts',(-118.779955786455,-121.619960181732,
-85.3940930246681));
#22898=CARTESIAN_POINT('Ctrl Pts',(-116.330634260069,-124.011396018774,
-81.8918489994245));
#22899=CARTESIAN_POINT('Ctrl Pts',(-120.526719842218,-125.454244503486,
-83.9470465127606));
#22900=CARTESIAN_POINT('Ctrl Pts',(-118.976188771633,-121.427849190968,
-85.1007432598167));
#22901=CARTESIAN_POINT('Ctrl Pts',(-116.226334686115,-124.121594328844,
-81.7284336163539));
#22902=CARTESIAN_POINT('Ctrl Pts',(-120.725838606432,-125.356776429138,
-83.8003716291909));
#22903=CARTESIAN_POINT('Ctrl Pts',(-119.229508592988,-121.178951530852,
-84.6051856591968));
#22904=CARTESIAN_POINT('Ctrl Pts',(-116.018327623084,-124.338324238805,
-81.6176595477855));
#22905=CARTESIAN_POINT('Ctrl Pts',(-120.982883719394,-125.230497467175,
-83.5525928299572));
#22906=CARTESIAN_POINT('Ctrl Pts',(-119.306430749595,-121.103197399823,
-84.4313845009826));
#22907=CARTESIAN_POINT('Ctrl Pts',(-115.938944698971,-124.420612015484,
-81.6055951047004));
#22908=CARTESIAN_POINT('Ctrl Pts',(-121.060937084107,-125.192063387035,
-83.4656922503483));
#22909=CARTESIAN_POINT('Ctrl Pts',(-119.440303841191,-120.971164568224,
-84.0733653040093));
#22910=CARTESIAN_POINT('Ctrl Pts',(-115.778652442949,-124.586368326783,
-81.6400246699534));
#22911=CARTESIAN_POINT('Ctrl Pts',(-121.196778897721,-125.125076140871,
-83.2866826521477));
#22912=CARTESIAN_POINT('Ctrl Pts',(-119.497839395063,-120.914311737671,
-83.8880856770369));
#22913=CARTESIAN_POINT('Ctrl Pts',(-115.697759349005,-124.669813047921,
-81.6878272780908));
#22914=CARTESIAN_POINT('Ctrl Pts',(-121.255160562605,-125.096231691082,
-83.1940428383556));
#22915=CARTESIAN_POINT('Ctrl Pts',(-119.592195409221,-120.82098824412,-83.5036466079758));
#22916=CARTESIAN_POINT('Ctrl Pts',(-115.551887637618,-124.820142027729,
-81.8435231238005));
#22917=CARTESIAN_POINT('Ctrl Pts',(-121.350904165271,-125.048883740856,
-83.0018233041507));
#22918=CARTESIAN_POINT('Ctrl Pts',(-119.628897626029,-120.784634828299,
-83.3034927483059));
#22919=CARTESIAN_POINT('Ctrl Pts',(-115.488159523427,-124.885734117082,
-81.9531151909483));
#22920=CARTESIAN_POINT('Ctrl Pts',(-121.388146120508,-125.030439729044,
-82.9017463741539));
#22921=CARTESIAN_POINT('Ctrl Pts',(-119.677240002648,-120.736735847766,
-82.9038841796134));
#22922=CARTESIAN_POINT('Ctrl Pts',(-115.400689666882,-124.975740417795,
-82.2081803578402));
#22923=CARTESIAN_POINT('Ctrl Pts',(-121.437199414473,-125.006138040429,
-82.7019420898058));
#22924=CARTESIAN_POINT('Ctrl Pts',(-119.689439202156,-120.724637682096,
-82.7026620014977));
#22925=CARTESIAN_POINT('Ctrl Pts',(-115.377099115996,-124.999999998111,
-82.3529550603246));
#22926=CARTESIAN_POINT('Ctrl Pts',(-121.449578013952,-125.,-82.6013310007496));
#22927=CARTESIAN_POINT('Ctrl Pts',(-119.689439203101,-120.724637681159,
-82.5));
#22928=CARTESIAN_POINT('Ctrl Pts',(-115.377099114166,-125.,-82.5));
#22929=CARTESIAN_POINT('Ctrl Pts',(-121.449578014911,-125.,-82.5));
#22930=CARTESIAN_POINT('Origin',(-116.189500386223,-127.5,-87.5));
#22931=CARTESIAN_POINT('Origin',(-168.964466094067,-137.5,-82.5));
#22932=CARTESIAN_POINT('Origin',(-168.964466094067,-137.5,-82.5));
#22933=CARTESIAN_POINT('Origin',(-177.5,-137.5,73.9644660940671));
#22934=CARTESIAN_POINT('Origin',(-177.5,-137.5,73.9644660940671));
#22935=CARTESIAN_POINT('Origin',(-177.5,-137.5,73.9644660940671));
#22936=CARTESIAN_POINT('Origin',(-177.5,-127.5,-73.9644660940673));
#22937=CARTESIAN_POINT('Origin',(-177.5,-127.5,-73.9644660940673));
#22938=CARTESIAN_POINT('Origin',(-147.5,-122.5,-37.5));
#22939=CARTESIAN_POINT('Origin',(-147.5,-122.5,-32.5));
#22940=CARTESIAN_POINT('Ctrl Pts',(-150.289855072464,-79.4541343310581,
-37.5));
#22941=CARTESIAN_POINT('Ctrl Pts',(-150.,-80.0024038100394,-37.5));
#22942=CARTESIAN_POINT('Ctrl Pts',(-150.,-80.6225774829855,-37.5));
#22943=CARTESIAN_POINT('Ctrl Pts',(-150.28985506853,-79.4541343384987,-37.2405761439445));
#22944=CARTESIAN_POINT('Ctrl Pts',(-149.999999996126,-80.0024038172978,
-37.3094148175651));
#22945=CARTESIAN_POINT('Ctrl Pts',(-150.,-80.6225774905387,-37.370288072025));
#22946=CARTESIAN_POINT('Ctrl Pts',(-150.2701197497,-79.4914922605523,-36.9888304197613));
#22947=CARTESIAN_POINT('Ctrl Pts',(-149.980519833119,-80.0389466368894,
-37.1241843229246));
#22948=CARTESIAN_POINT('Ctrl Pts',(-149.989987226484,-80.6604847938369,
-37.2444152098049));
#22949=CARTESIAN_POINT('Ctrl Pts',(-150.196231486306,-79.6310132970244,
-36.4987912993743));
#22950=CARTESIAN_POINT('Ctrl Pts',(-149.907890955038,-80.1748646486506,
-36.7663952057919));
#22951=CARTESIAN_POINT('Ctrl Pts',(-149.952499797667,-80.8020576101747,
-36.9993956497629));
#22952=CARTESIAN_POINT('Ctrl Pts',(-150.143050717943,-79.7313168859254,
-36.2679996568602));
#22953=CARTESIAN_POINT('Ctrl Pts',(-149.855501091412,-80.2727952833135,
-36.5988602080128));
#22954=CARTESIAN_POINT('Ctrl Pts',(-149.925518380098,-80.9038362519413,
-36.8839998280985));
#22955=CARTESIAN_POINT('Ctrl Pts',(-150.015028469708,-79.9719313539898,
-35.8382849920608));
#22956=CARTESIAN_POINT('Ctrl Pts',(-149.729850869406,-80.5068721381906,
-36.2906206071997));
#22957=CARTESIAN_POINT('Ctrl Pts',(-149.860565913637,-81.1479891679726,
-36.6691424963621));
#22958=CARTESIAN_POINT('Ctrl Pts',(-149.939105635844,-80.1142600764824,
-35.6362636343074));
#22959=CARTESIAN_POINT('Ctrl Pts',(-149.655266820466,-80.6454659181997,
-36.1475015807484));
#22960=CARTESIAN_POINT('Ctrl Pts',(-149.8220462428,-81.2924109599891,-36.5681318166794));
#22961=CARTESIAN_POINT('Ctrl Pts',(-149.775363670976,-80.4199633406166,
-35.2663619775736));
#22962=CARTESIAN_POINT('Ctrl Pts',(-149.494928348598,-80.9422362487731,
-35.8896065722342));
#22963=CARTESIAN_POINT('Ctrl Pts',(-149.738971273161,-81.6026098603025,
-36.3831809892611));
#22964=CARTESIAN_POINT('Ctrl Pts',(-149.686995608736,-80.5843780010491,
-35.096414733337));
#22965=CARTESIAN_POINT('Ctrl Pts',(-149.408398325687,-81.1018541496878,
-35.7733074247595));
#22966=CARTESIAN_POINT('Ctrl Pts',(-149.694137478568,-81.7694423834459,
-36.2982073663223));
#22967=CARTESIAN_POINT('Ctrl Pts',(-149.500255462679,-80.9302925286903,
-34.7789058669457));
#22968=CARTESIAN_POINT('Ctrl Pts',(-149.226078269656,-81.4367533718067,
-35.5604730905987));
#22969=CARTESIAN_POINT('Ctrl Pts',(-149.599394315017,-82.1204438893779,
-36.1394529338191));
#22970=CARTESIAN_POINT('Ctrl Pts',(-149.401347886677,-81.1127763961017,
-34.6307892928536));
#22971=CARTESIAN_POINT('Ctrl Pts',(-149.129574349821,-81.6133256610706,
-35.4636764520014));
#22972=CARTESIAN_POINT('Ctrl Pts',(-149.549213266549,-82.3056113431205,
-36.0653946460516));
#22973=CARTESIAN_POINT('Ctrl Pts',(-149.197899201606,-81.4863922312639,
-34.3564485886733));
#22974=CARTESIAN_POINT('Ctrl Pts',(-148.93165319989,-81.9738530462027,-35.2892543852097));
#22975=CARTESIAN_POINT('Ctrl Pts',(-149.445992976771,-82.6847215287652,
-35.9282242947119));
#22976=CARTESIAN_POINT('Ctrl Pts',(-149.093462145135,-81.6773447374821,
-34.2301909539054));
#22977=CARTESIAN_POINT('Ctrl Pts',(-148.830186520417,-82.1578926315274,
-35.2116962088616));
#22978=CARTESIAN_POINT('Ctrl Pts',(-149.393006529828,-82.8784821601051,
-35.8650954766799));
#22979=CARTESIAN_POINT('Ctrl Pts',(-148.773324875584,-82.2599185303359,
-33.8775006940139));
#22980=CARTESIAN_POINT('Ctrl Pts',(-148.518202139789,-82.721231742148,-35.0014947689296));
#22981=CARTESIAN_POINT('Ctrl Pts',(-149.230583943609,-83.4696232145796,
-35.6887503475526));
#22982=CARTESIAN_POINT('Ctrl Pts',(-148.550873607934,-82.6611103319686,
-33.6767887272455));
#22983=CARTESIAN_POINT('Ctrl Pts',(-148.30315471628,-83.1060920248233,-34.8943924369622));
#22984=CARTESIAN_POINT('Ctrl Pts',(-149.117722639557,-83.8767148956916,
-35.5883943633349));
#22985=CARTESIAN_POINT('Ctrl Pts',(-148.091214058597,-83.4818155627025,
-33.3265667074903));
#22986=CARTESIAN_POINT('Ctrl Pts',(-147.862495369544,-83.8874214153555,
-34.7305155227995));
#22987=CARTESIAN_POINT('Ctrl Pts',(-148.884513014786,-84.7094893209599,
-35.413283354033));
#22988=CARTESIAN_POINT('Ctrl Pts',(-147.853104568993,-83.9028862659571,
-33.1771134341839));
#22989=CARTESIAN_POINT('Ctrl Pts',(-147.635229789707,-84.286581928446,-34.6752930801302));
#22990=CARTESIAN_POINT('Ctrl Pts',(-148.763707465277,-85.1367522404598,
-35.338556716844));
#22991=CARTESIAN_POINT('Ctrl Pts',(-147.372342666232,-84.7444834282116,
-32.9266778278956));
#22992=CARTESIAN_POINT('Ctrl Pts',(-147.180928816256,-85.0771956930355,
-34.6125828689692));
#22993=CARTESIAN_POINT('Ctrl Pts',(-148.519791499653,-85.9907258315643,
-35.2133389141958));
#22994=CARTESIAN_POINT('Ctrl Pts',(-147.128665473948,-85.1668726405084,
-32.8248617968328));
#22995=CARTESIAN_POINT('Ctrl Pts',(-146.952267516985,-85.4713149459695,
-34.6060731019583));
#22996=CARTESIAN_POINT('Ctrl Pts',(-148.396161159612,-86.4193266499308,
-35.162430898305));
#22997=CARTESIAN_POINT('Ctrl Pts',(-146.388097896074,-86.4377602232233,
-32.58126559787));
#22998=CARTESIAN_POINT('Ctrl Pts',(-146.253862108749,-86.6644852388408,
-34.6540449090446));
#22999=CARTESIAN_POINT('Ctrl Pts',(-148.020432020732,-87.7089037559116,
-35.0406327991578));
#23000=CARTESIAN_POINT('Ctrl Pts',(-145.881711078453,-87.2899179999201,
-32.5000000009063));
#23001=CARTESIAN_POINT('Ctrl Pts',(-145.791767290395,-87.4382443129623,
-34.7842689266316));
#23002=CARTESIAN_POINT('Ctrl Pts',(-147.763515165392,-88.5735933110244,
-35.));
#23003=CARTESIAN_POINT('Ctrl Pts',(-145.36231884058,-88.1464478086875,-32.5));
#23004=CARTESIAN_POINT('Ctrl Pts',(-145.36231884058,-88.1464478086874,-35.0000000000001));
#23005=CARTESIAN_POINT('Ctrl Pts',(-147.5,-89.4427190999917,-35.));
#23006=CARTESIAN_POINT('Origin',(-147.5,-89.4427190999916,-32.5));
#23007=CARTESIAN_POINT('Origin',(0.,0.,-87.5));
#23008=CARTESIAN_POINT('Origin',(-104.163333279998,-137.5,-87.5));
#23009=CARTESIAN_POINT('Origin',(-180.,-137.5,-82.5));
#23010=CARTESIAN_POINT('Ctrl Pts',(-97.2111104761179,-140.,-82.5));
#23011=CARTESIAN_POINT('Ctrl Pts',(-97.2111104761179,-140.,-82.6755496768535));
#23012=CARTESIAN_POINT('Ctrl Pts',(-97.2669993053863,-139.980948398877,
-82.8433669193193));
#23013=CARTESIAN_POINT('Ctrl Pts',(-97.4416750152787,-139.921239210978,
-83.1407858319268));
#23014=CARTESIAN_POINT('Ctrl Pts',(-97.5528693408584,-139.883166869044,
-83.2647663586162));
#23015=CARTESIAN_POINT('Ctrl Pts',(-97.7975572341499,-139.799120034918,
-83.4891405228875));
#23016=CARTESIAN_POINT('Ctrl Pts',(-97.9325262666959,-139.752638285023,
-83.5889920461804));
#23017=CARTESIAN_POINT('Ctrl Pts',(-98.2091898573101,-139.657040028271,
-83.7678569462811));
#23018=CARTESIAN_POINT('Ctrl Pts',(-98.3521285688953,-139.607498613007,
-83.8477491623104));
#23019=CARTESIAN_POINT('Ctrl Pts',(-98.7901601853574,-139.455163852716,
-84.0681986935236));
#23020=CARTESIAN_POINT('Ctrl Pts',(-99.0953089605356,-139.348355708036,
-84.1900813067333));
#23021=CARTESIAN_POINT('Ctrl Pts',(-99.7103269532128,-139.131535702876,
-84.4002328533732));
#23022=CARTESIAN_POINT('Ctrl Pts',(-100.021642419245,-139.021028910904,
-84.4887015138217));
#23023=CARTESIAN_POINT('Ctrl Pts',(-100.963515042103,-138.68428076857,-84.7184070178217));
#23024=CARTESIAN_POINT('Ctrl Pts',(-101.60311676071,-138.452377890846,-84.8244784333066));
#23025=CARTESIAN_POINT('Ctrl Pts',(-102.880937057798,-137.982203598024,
-84.96529984463));
#23026=CARTESIAN_POINT('Ctrl Pts',(-103.521414707761,-137.743143193377,
-85.));
#23027=CARTESIAN_POINT('Ctrl Pts',(-104.163333279998,-137.5,-85.));
#23028=CARTESIAN_POINT('Origin',(-173.232233047034,-137.5,78.2322330470336));
#23029=CARTESIAN_POINT('Origin',(-168.964466094067,-137.5,82.5));
#23030=CARTESIAN_POINT('Origin',(-177.5,-125.,73.9644660940671));
#23031=CARTESIAN_POINT('Origin',(-177.5,-127.5,73.9644660940671));
#23032=CARTESIAN_POINT('Origin',(-177.5,-127.5,85.));
#23033=CARTESIAN_POINT('Origin',(-177.5,-127.5,73.9644660940672));
#23034=CARTESIAN_POINT('Origin',(-115.217186218029,-122.5,-32.5));
#23035=CARTESIAN_POINT('Origin',(0.,0.,-32.5));
#23036=CARTESIAN_POINT('Ctrl Pts',(-95.8063843937653,-140.431966711357,
-82.3302220946716));
#23037=CARTESIAN_POINT('Ctrl Pts',(-96.4436693342527,-139.997193891514,
-82.3767164474312));
#23038=CARTESIAN_POINT('Ctrl Pts',(-97.2155465823483,-139.998571769581,
-82.4151232270209));
#23039=CARTESIAN_POINT('Ctrl Pts',(-95.7923535903209,-140.44153068871,-82.6189757789389));
#23040=CARTESIAN_POINT('Ctrl Pts',(-96.4301984592198,-140.006470158917,
-82.5862803340843));
#23041=CARTESIAN_POINT('Ctrl Pts',(-97.2013093103816,-140.003422681504,
-82.5594793863893));
#23042=CARTESIAN_POINT('Ctrl Pts',(-95.8143433314505,-140.426549686738,
-82.8999538047632));
#23043=CARTESIAN_POINT('Ctrl Pts',(-96.4513705556942,-139.991898168234,
-82.7909496905929));
#23044=CARTESIAN_POINT('Ctrl Pts',(-97.2236226187953,-139.995824235922,
-82.6999480513205));
#23045=CARTESIAN_POINT('Ctrl Pts',(-95.9113524568369,-140.360304954438,
-83.3940569629634));
#23046=CARTESIAN_POINT('Ctrl Pts',(-96.5440906351143,-139.927939556875,
-83.1478648493756));
#23047=CARTESIAN_POINT('Ctrl Pts',(-97.3220593832045,-139.962224365005,
-82.9469649889257));
#23048=CARTESIAN_POINT('Ctrl Pts',(-95.9760732771133,-140.316081550096,
-83.6111084029453));
#23049=CARTESIAN_POINT('Ctrl Pts',(-96.6060933643896,-139.88514399948,-83.3040436736954));
#23050=CARTESIAN_POINT('Ctrl Pts',(-97.3877326179702,-139.939793891199,
-83.0554758102092));
#23051=CARTESIAN_POINT('Ctrl Pts',(-96.1359171968624,-140.206614708383,
-84.0186285797908));
#23052=CARTESIAN_POINT('Ctrl Pts',(-96.7586808353661,-139.779598324237,
-83.5942322269066));
#23053=CARTESIAN_POINT('Ctrl Pts',(-97.5499289003671,-139.884271165605,
-83.2592091881112));
#23054=CARTESIAN_POINT('Ctrl Pts',(-96.2312574439685,-140.141222656174,
-84.2116073129497));
#23055=CARTESIAN_POINT('Ctrl Pts',(-96.8497861981093,-139.716486932324,
-83.7303149679426));
#23056=CARTESIAN_POINT('Ctrl Pts',(-97.6466721866358,-139.851103576304,
-83.3556865024526));
#23057=CARTESIAN_POINT('Ctrl Pts',(-96.4473504048935,-139.992591935039,
-84.5797041056106));
#23058=CARTESIAN_POINT('Ctrl Pts',(-97.0555509298913,-139.573566933705,
-83.9861341719472));
#23059=CARTESIAN_POINT('Ctrl Pts',(-97.8659453704935,-139.775715999607,
-83.5397134594334));
#23060=CARTESIAN_POINT('Ctrl Pts',(-96.5679243919286,-139.909470610044,
-84.753989376282));
#23061=CARTESIAN_POINT('Ctrl Pts',(-97.1703586838473,-139.493647616232,
-84.1053449302004));
#23062=CARTESIAN_POINT('Ctrl Pts',(-97.988293803748,-139.733555567923,-83.6268467456611));
#23063=CARTESIAN_POINT('Ctrl Pts',(-96.9500803569865,-139.645185630461,
-85.2398999355243));
#23064=CARTESIAN_POINT('Ctrl Pts',(-97.5346293970093,-139.239315047688,
-84.432869704325));
#23065=CARTESIAN_POINT('Ctrl Pts',(-98.3760735528373,-139.599505523372,
-83.869778159324));
#23066=CARTESIAN_POINT('Ctrl Pts',(-97.2354525040936,-139.446786719831,
-85.5216876072799));
#23067=CARTESIAN_POINT('Ctrl Pts',(-97.8055901602077,-139.049145300856,
-84.6129417193589));
#23068=CARTESIAN_POINT('Ctrl Pts',(-98.6656453772933,-139.498873185455,
-84.0106618938592));
#23069=CARTESIAN_POINT('Ctrl Pts',(-97.8473613034821,-139.018104706213,
-86.0240708677861));
#23070=CARTESIAN_POINT('Ctrl Pts',(-98.3809815624785,-138.642451119717,
-84.9145219274105));
#23071=CARTESIAN_POINT('Ctrl Pts',(-99.2865604725273,-139.281432946433,
-84.261842700229));
#23072=CARTESIAN_POINT('Ctrl Pts',(-98.166043362077,-138.793333891558,-86.2379611602896));
#23073=CARTESIAN_POINT('Ctrl Pts',(-98.6796642081939,-138.429941914644,
-85.0311843476496));
#23074=CARTESIAN_POINT('Ctrl Pts',(-99.6099329912234,-139.167421255508,
-84.3687873468957));
#23075=CARTESIAN_POINT('Ctrl Pts',(-98.8213488187872,-138.327519386904,
-86.6110898616107));
#23076=CARTESIAN_POINT('Ctrl Pts',(-99.2879449246068,-137.99409288667,-85.2121201908135));
#23077=CARTESIAN_POINT('Ctrl Pts',(-100.27488438625,-138.931140045818,-84.5553582822015));
#23078=CARTESIAN_POINT('Ctrl Pts',(-99.158096702725,-138.086393592506,-86.7699896797119));
#23079=CARTESIAN_POINT('Ctrl Pts',(-99.5988267512419,-137.769758011627,
-85.2749349361932));
#23080=CARTESIAN_POINT('Ctrl Pts',(-100.616589177682,-138.808829045632,
-84.6348154491461));
#23081=CARTESIAN_POINT('Ctrl Pts',(-99.8465457819727,-137.589416498872,
-87.0407064600204));
#23082=CARTESIAN_POINT('Ctrl Pts',(-100.226641408904,-137.313468734571,
-85.3520865086701));
#23083=CARTESIAN_POINT('Ctrl Pts',(-101.315173303503,-138.556733152654,
-84.7701949757435));
#23084=CARTESIAN_POINT('Ctrl Pts',(-100.196958385718,-137.33447257932,-87.1516264431987));
#23085=CARTESIAN_POINT('Ctrl Pts',(-100.543205603967,-137.081667395925,
-85.3644982653947));
#23086=CARTESIAN_POINT('Ctrl Pts',(-101.670744758199,-138.427408643402,
-84.825669005131));
#23087=CARTESIAN_POINT('Ctrl Pts',(-101.28821838667,-136.53403653485,-87.424812055919));
#23088=CARTESIAN_POINT('Ctrl Pts',(-101.533114418462,-136.351795325561,
-85.3295920701886));
#23089=CARTESIAN_POINT('Ctrl Pts',(-102.778066848943,-138.021368555811,
-84.9623127946849));
#23090=CARTESIAN_POINT('Ctrl Pts',(-102.034252820327,-135.97755865104,-87.5102062320114));
#23091=CARTESIAN_POINT('Ctrl Pts',(-102.179857181136,-135.866853574869,
-85.1905835679741));
#23092=CARTESIAN_POINT('Ctrl Pts',(-103.535087152147,-137.73907034878,-85.0050578474458));
#23093=CARTESIAN_POINT('Ctrl Pts',(-102.783621163517,-135.408741267554,
-87.4990307673126));
#23094=CARTESIAN_POINT('Ctrl Pts',(-102.759250409398,-135.427238236657,
-84.9584361067278));
#23095=CARTESIAN_POINT('Ctrl Pts',(-104.295502567802,-137.450494181459,
-84.9995248789654));
#23096=CARTESIAN_POINT('Origin',(-97.2111104761179,-142.5,-82.5));
#23097=CARTESIAN_POINT('Origin',(-168.964466094067,-137.5,82.5));
#23098=CARTESIAN_POINT('Origin',(-168.964466094067,-137.5,82.5));
#23099=CARTESIAN_POINT('Origin',(-168.964466094067,-137.5,82.5));
#23100=CARTESIAN_POINT('Origin',(-177.5,-127.5,73.9644660940671));
#23101=CARTESIAN_POINT('Origin',(-177.5,-127.5,73.9644660940671));
#23102=CARTESIAN_POINT('Origin',(-97.2111104761179,-142.5,115.));
#23103=CARTESIAN_POINT('Origin',(-97.2111104761179,-142.5,82.5));
#23104=CARTESIAN_POINT('Origin',(0.,-137.5,82.5));
#23105=CARTESIAN_POINT('Ctrl Pts',(-104.163333279998,-137.5,85.));
#23106=CARTESIAN_POINT('Ctrl Pts',(-103.738099080441,-137.661068405961,
85.));
#23107=CARTESIAN_POINT('Ctrl Pts',(-103.313784132472,-137.820236149174,
84.9848502161634));
#23108=CARTESIAN_POINT('Ctrl Pts',(-102.890445132596,-137.977529707376,
84.9541805579568));
#23109=CARTESIAN_POINT('Ctrl Pts',(-102.674532847161,-138.057752913,84.9385383515953));
#23110=CARTESIAN_POINT('Ctrl Pts',(-102.458874713662,-138.137488523029,
84.9188583125581));
#23111=CARTESIAN_POINT('Ctrl Pts',(-102.243480097268,-138.216739650426,
84.8950864427477));
#23112=CARTESIAN_POINT('Ctrl Pts',(-102.169808729557,-138.243845894054,
84.8869557559584));
#23113=CARTESIAN_POINT('Ctrl Pts',(-102.096197177396,-138.270885582569,
84.8783493800412));
#23114=CARTESIAN_POINT('Ctrl Pts',(-102.022632569934,-138.297863659494,
84.8692643545073));
#23115=CARTESIAN_POINT('Ctrl Pts',(-101.824799549342,-138.370414232822,
84.8448325236913));
#23116=CARTESIAN_POINT('Ctrl Pts',(-101.627311999894,-138.442516995573,
84.8168822159707));
#23117=CARTESIAN_POINT('Ctrl Pts',(-101.42999704102,-138.514238577898,84.7850438375703));
#23118=CARTESIAN_POINT('Ctrl Pts',(-101.276966125295,-138.569863450352,
84.7603510508216));
#23119=CARTESIAN_POINT('Ctrl Pts',(-101.124039180306,-138.625258921571,
84.7333188027895));
#23120=CARTESIAN_POINT('Ctrl Pts',(-100.971140292634,-138.680453268945,
84.7037536341508));
#23121=CARTESIAN_POINT('Ctrl Pts',(-100.819413206494,-138.735224612453,
84.6744150499591));
#23122=CARTESIAN_POINT('Ctrl Pts',(-100.667483749192,-138.789877248555,
84.6424995110724));
#23123=CARTESIAN_POINT('Ctrl Pts',(-100.516166836934,-138.844125833747,
84.6079054671296));
#23124=CARTESIAN_POINT('Ctrl Pts',(-100.456828089701,-138.865399351931,
84.5943394539282));
#23125=CARTESIAN_POINT('Ctrl Pts',(-100.397584005817,-138.886610562357,
84.5803613497262));
#23126=CARTESIAN_POINT('Ctrl Pts',(-100.338485741259,-138.907741516914,
84.565964289852));
#23127=CARTESIAN_POINT('Ctrl Pts',(-100.220918177777,-138.949778535426,
84.5373233938226));
#23128=CARTESIAN_POINT('Ctrl Pts',(-100.103632370179,-138.991604254091,
84.5069540658058));
#23129=CARTESIAN_POINT('Ctrl Pts',(-99.9869935660692,-139.033088789031,
84.4747498712919));
#23130=CARTESIAN_POINT('Ctrl Pts',(-99.9720326094956,-139.038409902621,
84.4706191228734));
#23131=CARTESIAN_POINT('Ctrl Pts',(-99.9570823608136,-139.043725379489,
84.4664581642972));
#23132=CARTESIAN_POINT('Ctrl Pts',(-99.9421436485644,-139.049034924161,
84.4622667514209));
#23133=CARTESIAN_POINT('Ctrl Pts',(-99.8232112700053,-139.0913060896,84.4288974291803));
#23134=CARTESIAN_POINT('Ctrl Pts',(-99.7047475328351,-139.133296386698,
84.3935836754955));
#23135=CARTESIAN_POINT('Ctrl Pts',(-99.5868591110941,-139.174972397689,
84.3559924242641));
#23136=CARTESIAN_POINT('Ctrl Pts',(-99.5255437217676,-139.196648664126,
84.336440697551));
#23137=CARTESIAN_POINT('Ctrl Pts',(-99.4643844621158,-139.218239730484,
84.3162722626081));
#23138=CARTESIAN_POINT('Ctrl Pts',(-99.4033998553792,-139.239739634851,
84.2954359997591));
#23139=CARTESIAN_POINT('Ctrl Pts',(-99.3132315996693,-139.271528129989,
84.2646287259707));
#23140=CARTESIAN_POINT('Ctrl Pts',(-99.223535776852,-139.303085592255,84.2323955368028));
#23141=CARTESIAN_POINT('Ctrl Pts',(-99.1342049110009,-139.334451631701,
84.1984942631106));
#23142=CARTESIAN_POINT('Ctrl Pts',(-99.0808040909447,-139.353201838725,
84.1782285263033));
#23143=CARTESIAN_POINT('Ctrl Pts',(-99.0275342339471,-139.371883428182,
84.1573660209767));
#23144=CARTESIAN_POINT('Ctrl Pts',(-98.9743778992268,-139.390502757733,
84.1358481968094));
#23145=CARTESIAN_POINT('Ctrl Pts',(-98.8981671957289,-139.417197453882,
84.1049979034971));
#23146=CARTESIAN_POINT('Ctrl Pts',(-98.8224769045325,-139.443662996202,
84.0729177573328));
#23147=CARTESIAN_POINT('Ctrl Pts',(-98.7474387368693,-139.46985661819,84.0394249607335));
#23148=CARTESIAN_POINT('Ctrl Pts',(-98.6761330066818,-139.4947473558,84.0075981132516));
#23149=CARTESIAN_POINT('Ctrl Pts',(-98.6054159170073,-139.519392616372,
83.9744956741588));
#23150=CARTESIAN_POINT('Ctrl Pts',(-98.5354408951835,-139.543741578814,
83.9399393538181));
#23151=CARTESIAN_POINT('Ctrl Pts',(-98.5230520237326,-139.548052490877,
83.9338212591129));
#23152=CARTESIAN_POINT('Ctrl Pts',(-98.5106865249416,-139.552354076384,
83.9276575341684));
#23153=CARTESIAN_POINT('Ctrl Pts',(-98.4983453996891,-139.556646001529,
83.921447113738));
#23154=CARTESIAN_POINT('Ctrl Pts',(-98.4332103940779,-139.579298276965,
83.8886692461367));
#23155=CARTESIAN_POINT('Ctrl Pts',(-98.3686986921717,-139.601700795348,
83.8545667766362));
#23156=CARTESIAN_POINT('Ctrl Pts',(-98.3049498142096,-139.623806785601,
83.8189431096019));
#23157=CARTESIAN_POINT('Ctrl Pts',(-98.2461451146523,-139.644198299252,
83.7860823110428));
#23158=CARTESIAN_POINT('Ctrl Pts',(-98.1879895705334,-139.664337465922,
83.7519270259336));
#23159=CARTESIAN_POINT('Ctrl Pts',(-98.1306351301536,-139.684172991867,
83.7163018099732));
#23160=CARTESIAN_POINT('Ctrl Pts',(-98.1258128865628,-139.685840722163,
83.7133065149586));
#23161=CARTESIAN_POINT('Ctrl Pts',(-98.1209963324925,-139.687506296946,
83.710300816007));
#23162=CARTESIAN_POINT('Ctrl Pts',(-98.1161855731307,-139.689169680641,
83.7072846016472));
#23163=CARTESIAN_POINT('Ctrl Pts',(-98.1011329199801,-139.694374334612,
83.697847000393));
#23164=CARTESIAN_POINT('Ctrl Pts',(-98.0861233722941,-139.699562258723,
83.6882946516978));
#23165=CARTESIAN_POINT('Ctrl Pts',(-98.0711656112444,-139.704730507617,
83.6786258523484));
#23166=CARTESIAN_POINT('Ctrl Pts',(-98.0285985107537,-139.719438415389,
83.6511101865903));
#23167=CARTESIAN_POINT('Ctrl Pts',(-97.9864063827793,-139.734002420143,
83.6226254451987));
#23168=CARTESIAN_POINT('Ctrl Pts',(-97.9447745948348,-139.748359981237,
83.5930927466016));
#23169=CARTESIAN_POINT('Ctrl Pts',(-97.9055854441768,-139.761875149636,
83.5652928025733));
#23170=CARTESIAN_POINT('Ctrl Pts',(-97.8668926229667,-139.775207447803,
83.5365641602674));
#23171=CARTESIAN_POINT('Ctrl Pts',(-97.828893412403,-139.788290019043,83.5068350472078));
#23172=CARTESIAN_POINT('Ctrl Pts',(-97.804144005828,-139.796810876973,83.4874720684692));
#23173=CARTESIAN_POINT('Ctrl Pts',(-97.7796896932354,-139.805225503118,
83.4676845636184));
#23174=CARTESIAN_POINT('Ctrl Pts',(-97.7555963200441,-139.813511537342,
83.4474515115311));
#23175=CARTESIAN_POINT('Ctrl Pts',(-97.728363634325,-139.822877223255,83.424582138104));
#23176=CARTESIAN_POINT('Ctrl Pts',(-97.7016349752933,-139.832064017308,
83.4011923028985));
#23177=CARTESIAN_POINT('Ctrl Pts',(-97.6754851218662,-139.841046916235,
83.3772268830841));
#23178=CARTESIAN_POINT('Ctrl Pts',(-97.6463215006398,-139.851065093299,
83.3504994512098));
#23179=CARTESIAN_POINT('Ctrl Pts',(-97.6179056267942,-139.860816746996,
83.3230936650656));
#23180=CARTESIAN_POINT('Ctrl Pts',(-97.5902935806194,-139.87028550355,83.2948558990642));
#23181=CARTESIAN_POINT('Ctrl Pts',(-97.5639466259767,-139.879320433372,
83.2679118929831));
#23182=CARTESIAN_POINT('Ctrl Pts',(-97.5383314014496,-139.88809782761,83.2402104364255));
#23183=CARTESIAN_POINT('Ctrl Pts',(-97.5135388526037,-139.896588714057,
83.2116040346635));
#23184=CARTESIAN_POINT('Ctrl Pts',(-97.4980774724969,-139.901883886554,
83.1937642210211));
#23185=CARTESIAN_POINT('Ctrl Pts',(-97.4829368794924,-139.907067340337,
83.17557218315));
#23186=CARTESIAN_POINT('Ctrl Pts',(-97.4681484941753,-139.91212881033,83.1569890466364));
#23187=CARTESIAN_POINT('Ctrl Pts',(-97.4476130510072,-139.919157267269,
83.1311841372042));
#23188=CARTESIAN_POINT('Ctrl Pts',(-97.4277452420287,-139.925954449789,
83.1045520895884));
#23189=CARTESIAN_POINT('Ctrl Pts',(-97.4087167048375,-139.932462814289,
83.0770775195449));
#23190=CARTESIAN_POINT('Ctrl Pts',(-97.3896881676464,-139.938971178789,
83.0496029495014));
#23191=CARTESIAN_POINT('Ctrl Pts',(-97.3714983087636,-139.945190921619,
83.0212855162084));
#23192=CARTESIAN_POINT('Ctrl Pts',(-97.3543677310461,-139.951047779757,
82.9921212813803));
#23193=CARTESIAN_POINT('Ctrl Pts',(-97.3386981110691,-139.956405143811,
82.9654442781753));
#23194=CARTESIAN_POINT('Ctrl Pts',(-97.3240367075897,-139.961419891151,
82.9382531572));
#23195=CARTESIAN_POINT('Ctrl Pts',(-97.3105164866214,-139.966044132201,
82.910533567852));
#23196=CARTESIAN_POINT('Ctrl Pts',(-97.2987364265489,-139.970073196333,
82.8863817120154));
#23197=CARTESIAN_POINT('Ctrl Pts',(-97.2878230738592,-139.973805693467,
82.8618285577111));
#23198=CARTESIAN_POINT('Ctrl Pts',(-97.277894901901,-139.977199920877,82.8368687469214));
#23199=CARTESIAN_POINT('Ctrl Pts',(-97.2675449135807,-139.980738358185,
82.8108484733772));
#23200=CARTESIAN_POINT('Ctrl Pts',(-97.2582088704294,-139.983928680802,
82.7843403311583));
#23201=CARTESIAN_POINT('Ctrl Pts',(-97.2499984542927,-139.986731261435,
82.757268617013));
#23202=CARTESIAN_POINT('Ctrl Pts',(-97.2412356636815,-139.989722392072,
82.7283755915447));
#23203=CARTESIAN_POINT('Ctrl Pts',(-97.2338238173965,-139.992251733102,
82.6990112555058));
#23204=CARTESIAN_POINT('Ctrl Pts',(-97.2279126563665,-139.99426861304,82.6692964230559));
#23205=CARTESIAN_POINT('Ctrl Pts',(-97.2221710252593,-139.996227649603,
82.6404338010639));
#23206=CARTESIAN_POINT('Ctrl Pts',(-97.2178453353219,-139.997703166035,
82.6112405024812));
#23207=CARTESIAN_POINT('Ctrl Pts',(-97.2150271728466,-139.998664330779,
82.5818324954324));
#23208=CARTESIAN_POINT('Ctrl Pts',(-97.21242764044,-139.999550929378,82.5547059305124));
#23209=CARTESIAN_POINT('Ctrl Pts',(-97.2111104751974,-140.,82.5273967255209));
#23210=CARTESIAN_POINT('Ctrl Pts',(-97.2111104761178,-140.,82.5));
#23211=CARTESIAN_POINT('Origin',(-168.964466094067,0.,82.5));
#23212=CARTESIAN_POINT('Origin',(-168.964466094067,-127.5,82.5));
#23213=CARTESIAN_POINT('Origin',(-140.840826156048,-127.5,110.623639938019));
#23214=CARTESIAN_POINT('Origin',(-168.964466094067,-127.5,82.5));
#23215=CARTESIAN_POINT('Origin',(0.,-122.5,32.5));
#23216=CARTESIAN_POINT('Origin',(-147.5,-122.5,32.5));
#23217=CARTESIAN_POINT('Origin',(-121.449578014911,-122.5,115.));
#23218=CARTESIAN_POINT('Ctrl Pts',(-102.653719754201,-135.507246376812,
87.5));
#23219=CARTESIAN_POINT('Ctrl Pts',(-102.653719754201,-135.507246376812,
85.));
#23220=CARTESIAN_POINT('Ctrl Pts',(-104.163333279998,-137.5,85.));
#23221=CARTESIAN_POINT('Ctrl Pts',(-101.942824967883,-136.045785799024,
87.4999999986499));
#23222=CARTESIAN_POINT('Ctrl Pts',(-102.098115024429,-135.928145581712,
85.2088536164867));
#23223=CARTESIAN_POINT('Ctrl Pts',(-103.441984205064,-137.773229542126,
85.));
#23224=CARTESIAN_POINT('Ctrl Pts',(-101.239352594638,-136.569897864386,
87.412786288228));
#23225=CARTESIAN_POINT('Ctrl Pts',(-101.486609565828,-136.386099347641,
85.331905314613));
#23226=CARTESIAN_POINT('Ctrl Pts',(-102.728166603362,-138.039139357556,
84.9563931437868));
#23227=CARTESIAN_POINT('Ctrl Pts',(-100.196407749732,-137.334867215748,
87.1513844296707));
#23228=CARTESIAN_POINT('Ctrl Pts',(-100.54257036391,-137.08212804413,85.3647787687136));
#23229=CARTESIAN_POINT('Ctrl Pts',(-101.669884334297,-138.427248808045,
84.825692214999));
#23230=CARTESIAN_POINT('Ctrl Pts',(-99.8508244887539,-137.58630689324,87.0421034532917));
#23231=CARTESIAN_POINT('Ctrl Pts',(-100.230398916982,-137.310719986095,
85.3526237075885));
#23232=CARTESIAN_POINT('Ctrl Pts',(-101.319218966522,-138.554817467693,
84.7710517262891));
#23233=CARTESIAN_POINT('Ctrl Pts',(-99.1647702284533,-138.081596677989,
86.7728948774191));
#23234=CARTESIAN_POINT('Ctrl Pts',(-99.6048287382421,-137.765412086316,
85.2762415031115));
#23235=CARTESIAN_POINT('Ctrl Pts',(-100.623075672997,-138.806104197121,
84.6364474390664));
#23236=CARTESIAN_POINT('Ctrl Pts',(-98.8231223087188,-138.326258685221,
86.6120988871654));
#23237=CARTESIAN_POINT('Ctrl Pts',(-99.2895441365193,-137.992946799803,
85.2128933853019));
#23238=CARTESIAN_POINT('Ctrl Pts',(-100.276403519106,-138.930234185559,
84.5560494432021));
#23239=CARTESIAN_POINT('Ctrl Pts',(-98.1642932033775,-138.794578008566,
86.236965419431));
#23240=CARTESIAN_POINT('Ctrl Pts',(-98.6779850295722,-138.431144249613,
85.0309421888964));
#23241=CARTESIAN_POINT('Ctrl Pts',(-99.6078857505209,-139.167837372319,
84.3684827100962));
#23242=CARTESIAN_POINT('Ctrl Pts',(-97.8450871550092,-139.019702589725,
86.0223563343333));
#23243=CARTESIAN_POINT('Ctrl Pts',(-98.3787305056279,-138.644046161722,
84.9137267915435));
#23244=CARTESIAN_POINT('Ctrl Pts',(-99.283985495488,-139.28205498953,84.2611781664592));
#23245=CARTESIAN_POINT('Ctrl Pts',(-97.2348460956408,-139.447206832062,
85.5210364529044));
#23246=CARTESIAN_POINT('Ctrl Pts',(-97.8048933229574,-139.049632684085,
84.6126732163398));
#23247=CARTESIAN_POINT('Ctrl Pts',(-98.6647703029657,-139.498950525936,
84.0105182271597));
#23248=CARTESIAN_POINT('Ctrl Pts',(-96.9485250987458,-139.646264128654,
85.2381599055602));
#23249=CARTESIAN_POINT('Ctrl Pts',(-97.5330426499524,-139.240425205481,
84.4318673801205));
#23250=CARTESIAN_POINT('Ctrl Pts',(-98.3742387030706,-139.599942828535,
83.869079952008));
#23251=CARTESIAN_POINT('Ctrl Pts',(-96.5670588723941,-139.910067692477,
84.7527693623909));
#23252=CARTESIAN_POINT('Ctrl Pts',(-97.1694267365962,-139.49429609941,84.1046276840804));
#23253=CARTESIAN_POINT('Ctrl Pts',(-97.9871626793753,-139.7337843447,83.6263846815815));
#23254=CARTESIAN_POINT('Ctrl Pts',(-96.446921948779,-139.992887137954,84.5790592166605));
#23255=CARTESIAN_POINT('Ctrl Pts',(-97.0550355767484,-139.573924747954,
83.985796851679));
#23256=CARTESIAN_POINT('Ctrl Pts',(-97.8652590362145,-139.775803032622,
83.5395296080959));
#23257=CARTESIAN_POINT('Ctrl Pts',(-96.230792082191,-140.141542227306,84.2107293038302));
#23258=CARTESIAN_POINT('Ctrl Pts',(-96.8492338219199,-139.716869275045,
83.7297846724926));
#23259=CARTESIAN_POINT('Ctrl Pts',(-97.6459507893286,-139.851223630635,
83.3553646521495));
#23260=CARTESIAN_POINT('Ctrl Pts',(-96.1354852319174,-140.20691083986,84.0176816842604));
#23261=CARTESIAN_POINT('Ctrl Pts',(-96.7581590378938,-139.779958879001,
83.5936364082725));
#23262=CARTESIAN_POINT('Ctrl Pts',(-97.5492423676424,-139.884388586841,
83.2588408418563));
#23263=CARTESIAN_POINT('Ctrl Pts',(-95.9757708369295,-140.316288364145,
83.6101822300658));
#23264=CARTESIAN_POINT('Ctrl Pts',(-96.6056940387067,-139.885419084152,
83.3034331025056));
#23265=CARTESIAN_POINT('Ctrl Pts',(-97.3871792316287,-139.939881597544,
83.0550911153068));
#23266=CARTESIAN_POINT('Ctrl Pts',(-95.9112233305706,-140.360393155342,
83.3934903679299));
#23267=CARTESIAN_POINT('Ctrl Pts',(-96.5438567051695,-139.928100230385,
83.1474982708776));
#23268=CARTESIAN_POINT('Ctrl Pts',(-97.3216824971681,-139.962258291636,
82.9467451839126));
#23269=CARTESIAN_POINT('Ctrl Pts',(-95.8249655550993,-140.419296052404,
82.9539654903595));
#23270=CARTESIAN_POINT('Ctrl Pts',(-96.4613838167463,-139.984990149168,
82.8298756349127));
#23271=CARTESIAN_POINT('Ctrl Pts',(-97.2341562250557,-139.99214285053,82.7269827452321));
#23272=CARTESIAN_POINT('Ctrl Pts',(-95.802253798755,-140.434782611285,82.7294636530625));
#23273=CARTESIAN_POINT('Ctrl Pts',(-96.4395937226627,-140.0000000025,82.6666388430675));
#23274=CARTESIAN_POINT('Ctrl Pts',(-97.2111104722631,-140.,82.6147318264911));
#23275=CARTESIAN_POINT('Ctrl Pts',(-95.802253802551,-140.434782608696,82.5));
#23276=CARTESIAN_POINT('Ctrl Pts',(-96.4395937263074,-140.,82.5));
#23277=CARTESIAN_POINT('Ctrl Pts',(-97.2111104761179,-140.,82.5));
#23278=CARTESIAN_POINT('Origin',(-104.163333279998,-137.5,87.5));
#23279=CARTESIAN_POINT('Origin',(-168.964466094067,-127.5,82.5));
#23280=CARTESIAN_POINT('Origin',(-168.964466094067,-127.5,82.5));
#23281=CARTESIAN_POINT('Origin',(-147.5,-122.5,37.5));
#23282=CARTESIAN_POINT('Origin',(-152.5,-122.5,37.5));
#23283=CARTESIAN_POINT('Origin',(-147.5,-122.5,37.5));
#23284=CARTESIAN_POINT('Origin',(0.,0.,87.5));
#23285=CARTESIAN_POINT('Origin',(-116.189500386222,-127.5,87.5));
#23286=CARTESIAN_POINT('Origin',(0.,-127.5,82.5));
#23287=CARTESIAN_POINT('Ctrl Pts',(-121.449578014911,-125.,82.5));
#23288=CARTESIAN_POINT('Ctrl Pts',(-121.449578013665,-125.,82.5578430303778));
#23289=CARTESIAN_POINT('Ctrl Pts',(-121.445542821646,-125.002000739816,
82.6149744276206));
#23290=CARTESIAN_POINT('Ctrl Pts',(-121.437730668306,-125.005872173714,
82.6713216462766));
#23291=CARTESIAN_POINT('Ctrl Pts',(-121.431548654752,-125.008935766527,
82.7159110513069));
#23292=CARTESIAN_POINT('Ctrl Pts',(-121.423002583494,-125.013170255242,
82.760009542539));
#23293=CARTESIAN_POINT('Ctrl Pts',(-121.412240896123,-125.018501093781,
82.8035838902947));
#23294=CARTESIAN_POINT('Ctrl Pts',(-121.402625881463,-125.023263924083,
82.8425153308796));
#23295=CARTESIAN_POINT('Ctrl Pts',(-121.391240873519,-125.02890257476,82.8810286286794));
#23296=CARTESIAN_POINT('Ctrl Pts',(-121.378166904503,-125.035375090082,
82.9190974411551));
#23297=CARTESIAN_POINT('Ctrl Pts',(-121.359482649641,-125.044625083389,
82.9735022966162));
#23298=CARTESIAN_POINT('Ctrl Pts',(-121.337601423089,-125.055455126064,
83.0262941391223));
#23299=CARTESIAN_POINT('Ctrl Pts',(-121.312984159938,-125.067631742438,
83.0775690600153));
#23300=CARTESIAN_POINT('Ctrl Pts',(-121.309754155107,-125.069229423281,
83.0842967876761));
#23301=CARTESIAN_POINT('Ctrl Pts',(-121.306476982697,-125.070850319854,
83.0909983906631));
#23302=CARTESIAN_POINT('Ctrl Pts',(-121.303153626062,-125.072493934659,
83.0976740773907));
#23303=CARTESIAN_POINT('Ctrl Pts',(-121.28333698938,-125.082294543202,83.1374801147826));
#23304=CARTESIAN_POINT('Ctrl Pts',(-121.26193952168,-125.092872330006,83.17618707187));
#23305=CARTESIAN_POINT('Ctrl Pts',(-121.239293756531,-125.104060083144,
83.2137354525194));
#23306=CARTESIAN_POINT('Ctrl Pts',(-121.223112895711,-125.112053960817,
83.2405645358964));
#23307=CARTESIAN_POINT('Ctrl Pts',(-121.206293748505,-125.120359745354,
83.2668025986261));
#23308=CARTESIAN_POINT('Ctrl Pts',(-121.188944294236,-125.128923152136,
83.2924342403752));
#23309=CARTESIAN_POINT('Ctrl Pts',(-121.169248714547,-125.138644568041,
83.3215319880497));
#23310=CARTESIAN_POINT('Ctrl Pts',(-121.148816846868,-125.14872481678,83.3499289055538));
#23311=CARTESIAN_POINT('Ctrl Pts',(-121.127768696513,-125.159103720469,
83.3776130175156));
#23312=CARTESIAN_POINT('Ctrl Pts',(-121.095198113589,-125.175164368916,
83.4204523002623));
#23313=CARTESIAN_POINT('Ctrl Pts',(-121.06107241282,-125.191979398505,83.4617485539175));
#23314=CARTESIAN_POINT('Ctrl Pts',(-121.025604781292,-125.209440222843,
83.501677334517));
#23315=CARTESIAN_POINT('Ctrl Pts',(-120.994690465973,-125.224659435575,
83.536480078894));
#23316=CARTESIAN_POINT('Ctrl Pts',(-120.962755773204,-125.240369726302,
83.5702435568607));
#23317=CARTESIAN_POINT('Ctrl Pts',(-120.929914941896,-125.256512858459,
83.6030728931431));
#23318=CARTESIAN_POINT('Ctrl Pts',(-120.919024936224,-125.261865914206,
83.6139590870702));
#23319=CARTESIAN_POINT('Ctrl Pts',(-120.908034223584,-125.267267022157,
83.6247432148631));
#23320=CARTESIAN_POINT('Ctrl Pts',(-120.896946618515,-125.272714234811,
83.6354286063845));
#23321=CARTESIAN_POINT('Ctrl Pts',(-120.861818540488,-125.289972254912,
83.6692823795648));
#23322=CARTESIAN_POINT('Ctrl Pts',(-120.825696080648,-125.307703371905,
83.7021357945799));
#23323=CARTESIAN_POINT('Ctrl Pts',(-120.788855644393,-125.325770196084,
83.7339645608881));
#23324=CARTESIAN_POINT('Ctrl Pts',(-120.750104876469,-125.344773861135,
83.7674437826873));
#23325=CARTESIAN_POINT('Ctrl Pts',(-120.710559563375,-125.364149043196,
83.7997894992622));
#23326=CARTESIAN_POINT('Ctrl Pts',(-120.670490053905,-125.383761285265,
83.8309820047453));
#23327=CARTESIAN_POINT('Ctrl Pts',(-120.655933159393,-125.390886237448,
83.8423139630822));
#23328=CARTESIAN_POINT('Ctrl Pts',(-120.64130662474,-125.398042702867,83.8534937861157));
#23329=CARTESIAN_POINT('Ctrl Pts',(-120.62662193437,-125.405224965794,83.8645207217807));
#23330=CARTESIAN_POINT('Ctrl Pts',(-120.623763587428,-125.406622979559,
83.8666670937534));
#23331=CARTESIAN_POINT('Ctrl Pts',(-120.62090288229,-125.40802204969,83.8688077929118));
#23332=CARTESIAN_POINT('Ctrl Pts',(-120.618039908549,-125.409422131597,
83.8709428055742));
#23333=CARTESIAN_POINT('Ctrl Pts',(-120.561761358576,-125.436944067424,
83.9129115512495));
#23334=CARTESIAN_POINT('Ctrl Pts',(-120.504422162934,-125.464947521895,
83.9528770557974));
#23335=CARTESIAN_POINT('Ctrl Pts',(-120.446193115434,-125.493345150898,
83.9910922510509));
#23336=CARTESIAN_POINT('Ctrl Pts',(-120.399258153872,-125.516234785589,
84.0218952402349));
#23337=CARTESIAN_POINT('Ctrl Pts',(-120.351744177112,-125.539380959607,
84.0515603444803));
#23338=CARTESIAN_POINT('Ctrl Pts',(-120.303722804547,-125.562746846771,
84.0802057525297));
#23339=CARTESIAN_POINT('Ctrl Pts',(-120.237604852662,-125.594918034739,
84.1196460186027));
#23340=CARTESIAN_POINT('Ctrl Pts',(-120.170523556422,-125.627506495568,
84.1571520519609));
#23341=CARTESIAN_POINT('Ctrl Pts',(-120.102573990086,-125.660461610429,
84.1929593090857));
#23342=CARTESIAN_POINT('Ctrl Pts',(-120.054961757025,-125.683553245799,
84.2180494393613));
#23343=CARTESIAN_POINT('Ctrl Pts',(-120.006922336468,-125.706825340362,
84.24230479924));
#23344=CARTESIAN_POINT('Ctrl Pts',(-119.958477373249,-125.73026591296,84.2657976274668));
#23345=CARTESIAN_POINT('Ctrl Pts',(-119.957432170273,-125.730771644714,
84.2663044866393));
#23346=CARTESIAN_POINT('Ctrl Pts',(-119.956386759699,-125.731277463805,
84.2668109935507));
#23347=CARTESIAN_POINT('Ctrl Pts',(-119.955341143413,-125.731783369317,
84.2673171481934));
#23348=CARTESIAN_POINT('Ctrl Pts',(-119.89298150186,-125.761955131908,84.2975037687741));
#23349=CARTESIAN_POINT('Ctrl Pts',(-119.829839678401,-125.792457959603,
84.3264634103549));
#23350=CARTESIAN_POINT('Ctrl Pts',(-119.766290102992,-125.823110100769,
84.3541852883538));
#23351=CARTESIAN_POINT('Ctrl Pts',(-119.706671564982,-125.85186616769,84.3801923517616));
#23352=CARTESIAN_POINT('Ctrl Pts',(-119.646693089753,-125.880754168446,
84.4051101569439));
#23353=CARTESIAN_POINT('Ctrl Pts',(-119.586626434295,-125.909641987124,
84.4289275235297));
#23354=CARTESIAN_POINT('Ctrl Pts',(-119.501128626528,-125.950760393823,
84.4628287390102));
#23355=CARTESIAN_POINT('Ctrl Pts',(-119.415197450965,-125.99200199476,84.4946555586857));
#23356=CARTESIAN_POINT('Ctrl Pts',(-119.328730569191,-126.033415379519,
84.524664540591));
#23357=CARTESIAN_POINT('Ctrl Pts',(-119.297298692445,-126.048469702963,
84.5355732099124));
#23358=CARTESIAN_POINT('Ctrl Pts',(-119.265795758865,-126.063546844264,
84.5462412487785));
#23359=CARTESIAN_POINT('Ctrl Pts',(-119.2342159707,-126.078649522118,84.5566796096831));
#23360=CARTESIAN_POINT('Ctrl Pts',(-119.130353069599,-126.12832078426,84.5910103797512));
#23361=CARTESIAN_POINT('Ctrl Pts',(-119.025943929888,-126.178130418089,
84.6227652061914));
#23362=CARTESIAN_POINT('Ctrl Pts',(-118.920995425666,-126.22807113596,84.6522643594009));
#23363=CARTESIAN_POINT('Ctrl Pts',(-118.879152593277,-126.247982435342,
84.6640256334899));
#23364=CARTESIAN_POINT('Ctrl Pts',(-118.8372237143,-126.267914711427,84.6754278512293));
#23365=CARTESIAN_POINT('Ctrl Pts',(-118.795208048995,-126.287868028778,
84.686489443114));
#23366=CARTESIAN_POINT('Ctrl Pts',(-118.687953257466,-126.338803528124,
84.7147267380122));
#23367=CARTESIAN_POINT('Ctrl Pts',(-118.579924099525,-126.389974247274,
84.740767917434));
#23368=CARTESIAN_POINT('Ctrl Pts',(-118.471295931314,-126.441294374187,
84.7647575879331));
#23369=CARTESIAN_POINT('Ctrl Pts',(-118.355734714551,-126.495889940035,
84.7902783672878));
#23370=CARTESIAN_POINT('Ctrl Pts',(-118.239495199037,-126.550654804871,
84.8134776148503));
#23371=CARTESIAN_POINT('Ctrl Pts',(-118.122742883405,-126.605505676004,
84.8344961206034));
#23372=CARTESIAN_POINT('Ctrl Pts',(-118.065228912442,-126.632526051511,
84.8448501570355));
#23373=CARTESIAN_POINT('Ctrl Pts',(-118.007589863346,-126.659567573612,
84.8546744803528));
#23374=CARTESIAN_POINT('Ctrl Pts',(-117.949842319794,-126.686621640134,
84.8639830042663));
#23375=CARTESIAN_POINT('Ctrl Pts',(-117.876606796367,-126.720931648849,
84.8757880885903));
#23376=CARTESIAN_POINT('Ctrl Pts',(-117.803387560177,-126.755173054075,
84.8867590613587));
#23377=CARTESIAN_POINT('Ctrl Pts',(-117.730135337144,-126.789368961517,
84.8969279885251));
#23378=CARTESIAN_POINT('Ctrl Pts',(-117.43068222065,-126.929160910906,84.9384982891291));
#23379=CARTESIAN_POINT('Ctrl Pts',(-117.129946637153,-127.068588179685,
84.9667803785313));
#23380=CARTESIAN_POINT('Ctrl Pts',(-116.828007609149,-127.207574667086,
84.9830546228536));
#23381=CARTESIAN_POINT('Ctrl Pts',(-116.615757670973,-127.305276092282,
84.9944947052243));
#23382=CARTESIAN_POINT('Ctrl Pts',(-116.402913049513,-127.402759565778,
85.));
#23383=CARTESIAN_POINT('Ctrl Pts',(-116.189500386222,-127.5,85.));
#23384=CARTESIAN_POINT('Origin',(-152.5,-122.5,85.));
#23385=CARTESIAN_POINT('Origin',(-152.5,-122.5,44.5));
#23386=CARTESIAN_POINT('Origin',(-147.5,-79.9999999999999,37.5));
#23387=CARTESIAN_POINT('Ctrl Pts',(-147.5,-89.4427190999916,35.));
#23388=CARTESIAN_POINT('Ctrl Pts',(-147.692029124165,-88.8093685912677,
35.));
#23389=CARTESIAN_POINT('Ctrl Pts',(-147.881019325443,-88.1768396525257,
35.0215706395343));
#23390=CARTESIAN_POINT('Ctrl Pts',(-148.067032921848,-87.5451886198136,
35.0650289614011));
#23391=CARTESIAN_POINT('Ctrl Pts',(-148.113199638031,-87.3884191442644,
35.0758148827002));
#23392=CARTESIAN_POINT('Ctrl Pts',(-148.159182993743,-87.2317038217301,
35.0879492852221));
#23393=CARTESIAN_POINT('Ctrl Pts',(-148.204983936061,-87.075043664733,35.1014374973017));
#23394=CARTESIAN_POINT('Ctrl Pts',(-148.227650188964,-86.9975147197269,
35.1081126269109));
#23395=CARTESIAN_POINT('Ctrl Pts',(-148.250265804087,-86.9200215223737,
35.1151175424361));
#23396=CARTESIAN_POINT('Ctrl Pts',(-148.272833473781,-86.8425552539348,
35.122453276526));
#23397=CARTESIAN_POINT('Ctrl Pts',(-148.349179005414,-86.5804899398114,
35.1472697740457));
#23398=CARTESIAN_POINT('Ctrl Pts',(-148.424974341849,-86.3187382386178,
35.1759312643052));
#23399=CARTESIAN_POINT('Ctrl Pts',(-148.500300623518,-86.0570314559301,
35.2088246089155));
#23400=CARTESIAN_POINT('Ctrl Pts',(-148.548487711945,-85.8896146181409,
35.2298668596451));
#23401=CARTESIAN_POINT('Ctrl Pts',(-148.596482723485,-85.7222162995132,
35.2526418166148));
#23402=CARTESIAN_POINT('Ctrl Pts',(-148.644305530043,-85.5547679896948,
35.2772618566301));
#23403=CARTESIAN_POINT('Ctrl Pts',(-148.705029122316,-85.3421484547101,
35.3085234529103));
#23404=CARTESIAN_POINT('Ctrl Pts',(-148.765481316906,-85.1294146681304,
35.3427818320249));
#23405=CARTESIAN_POINT('Ctrl Pts',(-148.825445173605,-84.9173615305793,
35.3802763717601));
#23406=CARTESIAN_POINT('Ctrl Pts',(-148.844370664369,-84.8504343861759,
35.3921102097507));
#23407=CARTESIAN_POINT('Ctrl Pts',(-148.863247416388,-84.7835753431863,
35.4042666138849));
#23408=CARTESIAN_POINT('Ctrl Pts',(-148.882068323811,-84.7168103169457,
35.4167536897855));
#23409=CARTESIAN_POINT('Ctrl Pts',(-148.922791444531,-84.5723496827009,
35.4437721904293));
#23410=CARTESIAN_POINT('Ctrl Pts',(-148.963298334261,-84.4281714850036,
35.4723673050235));
#23411=CARTESIAN_POINT('Ctrl Pts',(-149.003534667861,-84.2844711674245,
35.5026558877997));
#23412=CARTESIAN_POINT('Ctrl Pts',(-149.04618468001,-84.132150621731,35.5347614080551));
#23413=CARTESIAN_POINT('Ctrl Pts',(-149.088661184858,-83.9798999176192,
35.5688472728226));
#23414=CARTESIAN_POINT('Ctrl Pts',(-149.130874866098,-83.8280577825359,
35.6051699481661));
#23415=CARTESIAN_POINT('Ctrl Pts',(-149.15342877087,-83.7469316415681,35.6245764092162));
#23416=CARTESIAN_POINT('Ctrl Pts',(-149.175907457633,-83.6659227742899,
35.6446218400823));
#23417=CARTESIAN_POINT('Ctrl Pts',(-149.198295785931,-83.5850879913789,
35.6653487918288));
#23418=CARTESIAN_POINT('Ctrl Pts',(-149.22791298944,-83.4781527979922,35.692768183748));
#23419=CARTESIAN_POINT('Ctrl Pts',(-149.257371929283,-83.3715229740751,
35.7213784233686));
#23420=CARTESIAN_POINT('Ctrl Pts',(-149.286670239395,-83.2652102229956,
35.7513256082022));
#23421=CARTESIAN_POINT('Ctrl Pts',(-149.305367124994,-83.1973661276528,
35.7704365769474));
#23422=CARTESIAN_POINT('Ctrl Pts',(-149.32399829751,-83.1296521692792,35.7900922410059));
#23423=CARTESIAN_POINT('Ctrl Pts',(-149.342561050911,-83.0620783213206,
35.8103347154936));
#23424=CARTESIAN_POINT('Ctrl Pts',(-149.371267458519,-82.95757860723,35.8416387311796));
#23425=CARTESIAN_POINT('Ctrl Pts',(-149.399774767598,-82.8535435891935,
35.8742597573608));
#23426=CARTESIAN_POINT('Ctrl Pts',(-149.428061694081,-82.7500633861383,
35.9084779858675));
#23427=CARTESIAN_POINT('Ctrl Pts',(-149.454923581065,-82.6517963113765,
35.9409723675908));
#23428=CARTESIAN_POINT('Ctrl Pts',(-149.48158676368,-82.5540293874095,35.9749069410037));
#23429=CARTESIAN_POINT('Ctrl Pts',(-149.508023085914,-82.4568752753999,
36.0105521857142));
#23430=CARTESIAN_POINT('Ctrl Pts',(-149.512553176896,-82.4402270834618,
36.0166603046949));
#23431=CARTESIAN_POINT('Ctrl Pts',(-149.517076580988,-82.4235969779229,
36.0228187343148));
#23432=CARTESIAN_POINT('Ctrl Pts',(-149.521593124104,-82.406985643267,36.0290289363984));
#23433=CARTESIAN_POINT('Ctrl Pts',(-149.546047412515,-82.3170455368254,
36.0626533409386));
#23434=CARTESIAN_POINT('Ctrl Pts',(-149.570311794236,-82.2276143985463,
36.0978073544095));
#23435=CARTESIAN_POINT('Ctrl Pts',(-149.594353719118,-82.1388178247615,
36.1347461416596));
#23436=CARTESIAN_POINT('Ctrl Pts',(-149.612438155897,-82.0720246693601,
36.1625316524285));
#23437=CARTESIAN_POINT('Ctrl Pts',(-149.63039654831,-82.0055912015912,36.1913275605255));
#23438=CARTESIAN_POINT('Ctrl Pts',(-149.648211128679,-81.9395854582945,
36.2212549329038));
#23439=CARTESIAN_POINT('Ctrl Pts',(-149.655934224025,-81.9109702095313,
36.2342292463902));
#23440=CARTESIAN_POINT('Ctrl Pts',(-149.663637104736,-81.8824099165123,
36.2474379019948));
#23441=CARTESIAN_POINT('Ctrl Pts',(-149.67131055004,-81.8539394834478,36.2608852437835));
#23442=CARTESIAN_POINT('Ctrl Pts',(-149.685698655415,-81.8005559543076,
36.2860997026084));
#23443=CARTESIAN_POINT('Ctrl Pts',(-149.69999936079,-81.7474243597968,36.3121788856582));
#23444=CARTESIAN_POINT('Ctrl Pts',(-149.714175605302,-81.6946906272139,
36.3392201558208));
#23445=CARTESIAN_POINT('Ctrl Pts',(-149.727286670739,-81.6459192182506,
36.3642295906055));
#23446=CARTESIAN_POINT('Ctrl Pts',(-149.740291333114,-81.5974878781538,
36.3900621046248));
#23447=CARTESIAN_POINT('Ctrl Pts',(-149.75314895044,-81.5495528039286,36.4168048599562));
#23448=CARTESIAN_POINT('Ctrl Pts',(-149.76292982072,-81.5130882918069,36.4371482419517));
#23449=CARTESIAN_POINT('Ctrl Pts',(-149.772625404106,-81.4769116545281,
36.458018554439));
#23450=CARTESIAN_POINT('Ctrl Pts',(-149.782212501331,-81.4411109947051,
36.4794579384388));
#23451=CARTESIAN_POINT('Ctrl Pts',(-149.792712453297,-81.4019015030656,
36.5029387164987));
#23452=CARTESIAN_POINT('Ctrl Pts',(-149.80309231573,-81.3631061432697,36.5271022623878));
#23453=CARTESIAN_POINT('Ctrl Pts',(-149.813325028167,-81.3248298095044,
36.5520580116842));
#23454=CARTESIAN_POINT('Ctrl Pts',(-149.822817814989,-81.2893212306205,
36.5752092151911));
#23455=CARTESIAN_POINT('Ctrl Pts',(-149.832167251568,-81.2543175533046,
36.5989995466176));
#23456=CARTESIAN_POINT('Ctrl Pts',(-149.841373631764,-81.2198208404941,
36.623594471715));
#23457=CARTESIAN_POINT('Ctrl Pts',(-149.850444720927,-81.1858310691555,
36.6478279656349));
#23458=CARTESIAN_POINT('Ctrl Pts',(-149.859377062136,-81.1523329411744,
36.6728423499023));
#23459=CARTESIAN_POINT('Ctrl Pts',(-149.868158592942,-81.1193744240715,
36.6988172833931));
#23460=CARTESIAN_POINT('Ctrl Pts',(-149.876313696672,-81.0887669899376,
36.7229393051294));
#23461=CARTESIAN_POINT('Ctrl Pts',(-149.884338741479,-81.0586248955665,
36.7478897210636));
#23462=CARTESIAN_POINT('Ctrl Pts',(-149.8922125854,-81.0290296766823,36.773832259155));
#23463=CARTESIAN_POINT('Ctrl Pts',(-149.892817407753,-81.0267563461321,
36.7758250122624));
#23464=CARTESIAN_POINT('Ctrl Pts',(-149.893421331922,-81.0244862651329,
36.7778236297172));
#23465=CARTESIAN_POINT('Ctrl Pts',(-149.894024345238,-81.0222194822742,
36.7798281910486));
#23466=CARTESIAN_POINT('Ctrl Pts',(-149.901678691384,-80.9934460867894,
36.805273079051));
#23467=CARTESIAN_POINT('Ctrl Pts',(-149.909127380051,-80.9654260581732,
36.8314799870868));
#23468=CARTESIAN_POINT('Ctrl Pts',(-149.916327644768,-80.9383234966228,
36.8585857768089));
#23469=CARTESIAN_POINT('Ctrl Pts',(-149.922896825408,-80.9135964026004,
36.8833158160623));
#23470=CARTESIAN_POINT('Ctrl Pts',(-149.929259164437,-80.889633198716,36.9087941212802));
#23471=CARTESIAN_POINT('Ctrl Pts',(-149.935369835439,-80.8666055523405,
36.935135681796));
#23472=CARTESIAN_POINT('Ctrl Pts',(-149.935956871689,-80.8643933463222,
36.9376662469157));
#23473=CARTESIAN_POINT('Ctrl Pts',(-149.936541575423,-80.86218981226,36.9402047878343));
#23474=CARTESIAN_POINT('Ctrl Pts',(-149.937123900464,-80.8599951269442,
36.9427514122746));
#23475=CARTESIAN_POINT('Ctrl Pts',(-149.949888621083,-80.8118870379003,
36.9985741010473));
#23476=CARTESIAN_POINT('Ctrl Pts',(-149.961572072671,-80.7677918263995,
37.0585526832355));
#23477=CARTESIAN_POINT('Ctrl Pts',(-149.971367310254,-80.7307169524392,
37.1227154597912));
#23478=CARTESIAN_POINT('Ctrl Pts',(-149.975158206732,-80.7163684480826,
37.1475473683212));
#23479=CARTESIAN_POINT('Ctrl Pts',(-149.978650998302,-80.7031305919437,
37.1730908787877));
#23480=CARTESIAN_POINT('Ctrl Pts',(-149.981796037926,-80.6911891223571,
37.1992286595141));
#23481=CARTESIAN_POINT('Ctrl Pts',(-149.985757876154,-80.6761463323226,
37.2321546862971));
#23482=CARTESIAN_POINT('Ctrl Pts',(-149.989179977686,-80.6631984113665,
37.2661215533609));
#23483=CARTESIAN_POINT('Ctrl Pts',(-149.991954976261,-80.6527310533642,
37.3008958029159));
#23484=CARTESIAN_POINT('Ctrl Pts',(-149.993127423005,-80.6483085574699,
37.3155880467323));
#23485=CARTESIAN_POINT('Ctrl Pts',(-149.994184300917,-80.6443291875706,
37.33042386883));
#23486=CARTESIAN_POINT('Ctrl Pts',(-149.995117265699,-80.6408234431072,
37.3453832597703));
#23487=CARTESIAN_POINT('Ctrl Pts',(-149.997168971269,-80.6331138750977,
37.3782808206269));
#23488=CARTESIAN_POINT('Ctrl Pts',(-149.998622294847,-80.6276965661502,
37.4117792041199));
#23489=CARTESIAN_POINT('Ctrl Pts',(-149.999384955835,-80.624860626989,37.4456825897666));
#23490=CARTESIAN_POINT('Ctrl Pts',(-149.999789923498,-80.6233547630872,
37.4636850509239));
#23491=CARTESIAN_POINT('Ctrl Pts',(-150.,-80.6225774829854,37.481801403423));
#23492=CARTESIAN_POINT('Ctrl Pts',(-150.,-80.6225774829854,37.5));
#23493=CARTESIAN_POINT('Origin',(0.,0.,32.5));
#23494=CARTESIAN_POINT('Origin',(-147.5,-89.4427190999916,32.5));
#23495=CARTESIAN_POINT('Ctrl Pts',(-119.689439203101,-120.724637681159,
82.5));
#23496=CARTESIAN_POINT('Ctrl Pts',(-115.377099114166,-125.,82.5));
#23497=CARTESIAN_POINT('Ctrl Pts',(-121.449578014911,-125.,82.5));
#23498=CARTESIAN_POINT('Ctrl Pts',(-119.689439200917,-120.724637683324,
82.7056798133782));
#23499=CARTESIAN_POINT('Ctrl Pts',(-115.377099118341,-124.999999995701,
82.3507082521197));
#23500=CARTESIAN_POINT('Ctrl Pts',(-121.449578012695,-125.,82.6028399066646));
#23501=CARTESIAN_POINT('Ctrl Pts',(-119.676882557983,-120.737090180421,
82.9079954286207));
#23502=CARTESIAN_POINT('Ctrl Pts',(-115.401361881511,-124.975048941511,
82.2053610116202));
#23503=CARTESIAN_POINT('Ctrl Pts',(-121.436836713265,-125.006317811859,
82.7039977143433));
#23504=CARTESIAN_POINT('Ctrl Pts',(-119.628410587298,-120.785117230515,
83.3063417968652));
#23505=CARTESIAN_POINT('Ctrl Pts',(-115.489012547634,-124.884856124345,
81.9514922386294));
#23506=CARTESIAN_POINT('Ctrl Pts',(-121.387651919446,-125.030684477513,
82.9031708983997));
#23507=CARTESIAN_POINT('Ctrl Pts',(-119.592485604525,-120.820701126369,
83.5023756354685));
#23508=CARTESIAN_POINT('Ctrl Pts',(-115.551419916513,-124.820623886438,
81.844093442978));
#23509=CARTESIAN_POINT('Ctrl Pts',(-121.351198628156,-125.048738071447,
83.0011878177447));
#23510=CARTESIAN_POINT('Ctrl Pts',(-119.497801818693,-120.91434900059,83.8883271564993));
#23511=CARTESIAN_POINT('Ctrl Pts',(-115.697825563992,-124.669744960185,
81.6876871655071));
#23512=CARTESIAN_POINT('Ctrl Pts',(-121.255122433638,-125.096250595907,
83.1941635782393));
#23513=CARTESIAN_POINT('Ctrl Pts',(-119.439376348876,-120.972080469663,
84.0761788301475));
#23514=CARTESIAN_POINT('Ctrl Pts',(-115.779889571829,-124.585091209873,
81.639444465222));
#23515=CARTESIAN_POINT('Ctrl Pts',(-121.195837765812,-125.125540825988,
83.2880894152805));
#23516=CARTESIAN_POINT('Ctrl Pts',(-119.305221428487,-121.104388919918,
84.4342801401529));
#23517=CARTESIAN_POINT('Ctrl Pts',(-115.940258775456,-124.419250986645,
81.6056236890861));
#23518=CARTESIAN_POINT('Ctrl Pts',(-121.059709978865,-125.192667908432,
83.4671400698696));
#23519=CARTESIAN_POINT('Ctrl Pts',(-119.229146767872,-121.179307379907,
84.6059387232763));
#23520=CARTESIAN_POINT('Ctrl Pts',(-116.018662098376,-124.337976550129,
81.6177805257506));
#23521=CARTESIAN_POINT('Ctrl Pts',(-120.982516573327,-125.230678008636,
83.5529693617978));
#23522=CARTESIAN_POINT('Ctrl Pts',(-119.060491893051,-121.345017393603,
84.9357796688685));
#23523=CARTESIAN_POINT('Ctrl Pts',(-116.159254888288,-124.191486350903,
81.6927658265867));
#23524=CARTESIAN_POINT('Ctrl Pts',(-120.811381479668,-125.314751472042,
83.7178898342746));
#23525=CARTESIAN_POINT('Ctrl Pts',(-118.96776206845,-121.435951457507,85.093861858456));
#23526=CARTESIAN_POINT('Ctrl Pts',(-116.221496701314,-124.12623198531,81.7541916577615));
#23527=CARTESIAN_POINT('Ctrl Pts',(-120.717287981259,-125.36088713601,83.7969309295804));
#23528=CARTESIAN_POINT('Ctrl Pts',(-118.772148188168,-121.627281202587,
85.3899146057789));
#23529=CARTESIAN_POINT('Ctrl Pts',(-116.320002770212,-124.021697634043,
81.9095222659674));
#23530=CARTESIAN_POINT('Ctrl Pts',(-120.518797426192,-125.45795884595,83.9449573025371));
#23531=CARTESIAN_POINT('Ctrl Pts',(-118.66868983755,-121.728242289117,85.5290754975167));
#23532=CARTESIAN_POINT('Ctrl Pts',(-116.35752640374,-123.981145420879,82.0023320413466));
#23533=CARTESIAN_POINT('Ctrl Pts',(-120.413817629313,-125.50918174931,84.0145377490307));
#23534=CARTESIAN_POINT('Ctrl Pts',(-118.45169839953,-121.939403249423,85.7917547211079));
#23535=CARTESIAN_POINT('Ctrl Pts',(-116.406873166747,-123.925571355125,
82.2074570860312));
#23536=CARTESIAN_POINT('Ctrl Pts',(-120.193635140666,-125.616314884214,
84.1458773602816));
#23537=CARTESIAN_POINT('Ctrl Pts',(-118.338158476483,-122.049610026221,
85.9152619328964));
#23538=CARTESIAN_POINT('Ctrl Pts',(-116.419520677459,-123.909734352817,
82.3190059601612));
#23539=CARTESIAN_POINT('Ctrl Pts',(-120.078425512936,-125.672228616066,
84.2076309666417));
#23540=CARTESIAN_POINT('Ctrl Pts',(-118.101739972007,-122.278395780866,
86.1479296435188));
#23541=CARTESIAN_POINT('Ctrl Pts',(-116.420156575106,-123.902371131663,
82.5520650696801));
#23542=CARTESIAN_POINT('Ctrl Pts',(-119.838530265679,-125.788303741941,
84.323964821566));
#23543=CARTESIAN_POINT('Ctrl Pts',(-117.978621353548,-122.397201959151,
86.2571677342239));
#23544=CARTESIAN_POINT('Ctrl Pts',(-116.408784821067,-123.910208556756,
82.6734238697007));
#23545=CARTESIAN_POINT('Ctrl Pts',(-119.713601079353,-125.848580405477,
84.3785838674499));
#23546=CARTESIAN_POINT('Ctrl Pts',(-117.603241895162,-122.758291253176,
86.5592543593046));
#23547=CARTESIAN_POINT('Ctrl Pts',(-116.343210235511,-123.964762276173,
83.0296153459409));
#23548=CARTESIAN_POINT('Ctrl Pts',(-119.332701334762,-126.031780121634,
84.5296271789764));
#23549=CARTESIAN_POINT('Ctrl Pts',(-117.342767505456,-123.007368772318,
86.7291564746629));
#23550=CARTESIAN_POINT('Ctrl Pts',(-116.259553389397,-124.040181684855,
83.2697315003776));
#23551=CARTESIAN_POINT('Ctrl Pts',(-119.068396439392,-126.158150332831,
84.6145782376957));
#23552=CARTESIAN_POINT('Ctrl Pts',(-116.804336290701,-123.518763278367,
87.016825817368));
#23553=CARTESIAN_POINT('Ctrl Pts',(-116.02736829311,-124.252946369571,83.719666170302));
#23554=CARTESIAN_POINT('Ctrl Pts',(-118.522047118472,-126.417607839943,
84.7584129083197));
#23555=CARTESIAN_POINT('Ctrl Pts',(-116.525023660543,-123.782353191698,
87.1348755768559));
#23556=CARTESIAN_POINT('Ctrl Pts',(-115.881406957195,-124.387808755614,
83.9325453429328));
#23557=CARTESIAN_POINT('Ctrl Pts',(-118.238626949676,-126.551340957402,
84.8174377888648));
#23558=CARTESIAN_POINT('Ctrl Pts',(-115.67127235659,-124.582362934986,87.4141780079963));
#23559=CARTESIAN_POINT('Ctrl Pts',(-115.387279747809,-124.844116246409,
84.4905439734664));
#23560=CARTESIAN_POINT('Ctrl Pts',(-117.372320479466,-126.95722825408,84.9570890031244));
#23561=CARTESIAN_POINT('Ctrl Pts',(-115.09272258053,-125.11712992375,87.4999999999441));
#23562=CARTESIAN_POINT('Ctrl Pts',(-114.975356365161,-125.224084605227,
84.7914664637573));
#23563=CARTESIAN_POINT('Ctrl Pts',(-116.78526355091,-127.228543433485,85.));
#23564=CARTESIAN_POINT('Ctrl Pts',(-114.505594583524,-125.652173913043,
87.5));
#23565=CARTESIAN_POINT('Ctrl Pts',(-114.505594583524,-125.652173913043,
85.));
#23566=CARTESIAN_POINT('Ctrl Pts',(-116.189500386222,-127.5,85.));
#23567=CARTESIAN_POINT('Origin',(-121.449578014911,-122.5,82.5));
#23568=CARTESIAN_POINT('Origin',(-147.5,-122.5,44.5));
#23569=CARTESIAN_POINT('Origin',(-147.5,-122.5,49.5));
#23570=CARTESIAN_POINT('Origin',(-147.5,-122.5,44.5));
#23571=CARTESIAN_POINT('Ctrl Pts',(-145.36231884058,-88.1464478086873,32.5));
#23572=CARTESIAN_POINT('Ctrl Pts',(-145.36231884058,-88.1464478086873,35.));
#23573=CARTESIAN_POINT('Ctrl Pts',(-147.5,-89.4427190999916,35.));
#23574=CARTESIAN_POINT('Ctrl Pts',(-145.88328041902,-87.2873300001825,32.5000000009303));
#23575=CARTESIAN_POINT('Ctrl Pts',(-145.793011707092,-87.4361921450511,
34.7836438007663));
#23576=CARTESIAN_POINT('Ctrl Pts',(-147.764311380887,-88.5709672327986,
35.));
#23577=CARTESIAN_POINT('Ctrl Pts',(-146.390924783419,-86.432995377738,32.5817470282981));
#23578=CARTESIAN_POINT('Ctrl Pts',(-146.25636627112,-86.6602829701382,34.6533815799931));
#23579=CARTESIAN_POINT('Ctrl Pts',(-148.021866250329,-87.7040688391623,
35.0408735143651));
#23580=CARTESIAN_POINT('Ctrl Pts',(-147.13295559207,-85.1594666843921,32.8264997589536));
#23581=CARTESIAN_POINT('Ctrl Pts',(-146.95625485105,-85.4644664729224,34.606035054135));
#23582=CARTESIAN_POINT('Ctrl Pts',(-148.398337763665,-86.4118117826985,
35.1632498793688));
#23583=CARTESIAN_POINT('Ctrl Pts',(-147.377049426154,-84.7363019818542,
32.9287776457782));
#23584=CARTESIAN_POINT('Ctrl Pts',(-147.185340564392,-85.0695699101127,
34.6128471107274));
#23585=CARTESIAN_POINT('Ctrl Pts',(-148.522179488132,-85.9824240698147,
35.2143888231312));
#23586=CARTESIAN_POINT('Ctrl Pts',(-147.858493843555,-83.8933928830767,
33.1802802395072));
#23587=CARTESIAN_POINT('Ctrl Pts',(-147.640340054158,-84.2776371924663,
34.6763398436954));
#23588=CARTESIAN_POINT('Ctrl Pts',(-148.766441729588,-85.1271192490123,
35.3401401195115));
#23589=CARTESIAN_POINT('Ctrl Pts',(-148.095887496716,-83.4735259621086,
33.329690382783));
#23590=CARTESIAN_POINT('Ctrl Pts',(-147.866955151253,-83.8795640251351,
34.7317798844392));
#23591=CARTESIAN_POINT('Ctrl Pts',(-148.886884097334,-84.7010778144719,
35.4148451917151));
#23592=CARTESIAN_POINT('Ctrl Pts',(-148.555727425865,-82.65238822296,33.6809331684156));
#23593=CARTESIAN_POINT('Ctrl Pts',(-148.307824862021,-83.0977615436487,
34.8965208417471));
#23594=CARTESIAN_POINT('Ctrl Pts',(-149.120185238387,-83.867864520377,35.5904665838843));
#23595=CARTESIAN_POINT('Ctrl Pts',(-148.780093861296,-82.2476812683581,
33.8839399244617));
#23596=CARTESIAN_POINT('Ctrl Pts',(-148.524727773055,-82.7095240936236,
35.0050364952365));
#23597=CARTESIAN_POINT('Ctrl Pts',(-149.234018208522,-83.457205992854,35.691969962678));
#23598=CARTESIAN_POINT('Ctrl Pts',(-149.207972890121,-81.4688789012013,
34.3573989375128));
#23599=CARTESIAN_POINT('Ctrl Pts',(-148.93931728545,-81.9607628458225,35.2860875789467));
#23600=CARTESIAN_POINT('Ctrl Pts',(-149.4511038933,-82.6669506497871,35.9286994683092));
#23601=CARTESIAN_POINT('Ctrl Pts',(-149.410469407752,-81.0966396786721,
34.6254381321728));
#23602=CARTESIAN_POINT('Ctrl Pts',(-149.13707735126,-81.6002642788733,35.4559386647908));
#23603=CARTESIAN_POINT('Ctrl Pts',(-149.553841095111,-82.2892373209608,
36.0627190669335));
#23604=CARTESIAN_POINT('Ctrl Pts',(-149.689478100498,-80.5797647052593,
35.1010485304976));
#23605=CARTESIAN_POINT('Ctrl Pts',(-149.410828634125,-81.0973762069276,
35.7764659917703));
#23606=CARTESIAN_POINT('Ctrl Pts',(-149.695396978193,-81.7647612450649,
36.3005242648253));
#23607=CARTESIAN_POINT('Ctrl Pts',(-149.778860900691,-80.4134491496535,
35.2734504935396));
#23608=CARTESIAN_POINT('Ctrl Pts',(-149.498351131341,-80.935915280146,35.8944893614103));
#23609=CARTESIAN_POINT('Ctrl Pts',(-149.74074560314,-81.5959998724055,36.3867252471529));
#23610=CARTESIAN_POINT('Ctrl Pts',(-149.942345818684,-80.1081950067706,
35.6444293836573));
#23611=CARTESIAN_POINT('Ctrl Pts',(-149.658443692203,-80.6395711160542,
36.1532547010742));
#23612=CARTESIAN_POINT('Ctrl Pts',(-149.823690158896,-81.2862566980837,
36.5722146914456));
#23613=CARTESIAN_POINT('Ctrl Pts',(-150.016754772459,-79.9686937648418,
35.8430315532085));
#23614=CARTESIAN_POINT('Ctrl Pts',(-149.731542660712,-80.5037270542566,
36.2939840338164));
#23615=CARTESIAN_POINT('Ctrl Pts',(-149.861441758745,-81.144703967216,36.6715157768338));
#23616=CARTESIAN_POINT('Ctrl Pts',(-150.145196691125,-79.7272764209246,
36.2762826327136));
#23617=CARTESIAN_POINT('Ctrl Pts',(-149.857607243134,-80.2688649285009,
36.6048325581329));
#23618=CARTESIAN_POINT('Ctrl Pts',(-149.926607145573,-80.8997363683411,
36.8881413161273));
#23619=CARTESIAN_POINT('Ctrl Pts',(-150.197080555724,-79.6294105444985,
36.5038809199123));
#23620=CARTESIAN_POINT('Ctrl Pts',(-149.908727602392,-80.1732994372084,
36.7701162187303));
#23621=CARTESIAN_POINT('Ctrl Pts',(-149.952930574586,-80.8004312877628,
37.0019404601773));
#23622=CARTESIAN_POINT('Ctrl Pts',(-150.269771338359,-79.4921496315481,
36.9870649844503));
#23623=CARTESIAN_POINT('Ctrl Pts',(-149.980179574577,-80.0395829024242,
37.1229099719677));
#23624=CARTESIAN_POINT('Ctrl Pts',(-149.989810459912,-80.6611518320492,
37.243532492004));
#23625=CARTESIAN_POINT('Ctrl Pts',(-150.289855071895,-79.4541343321333,
37.2465705504854));
#23626=CARTESIAN_POINT('Ctrl Pts',(-149.99999999943,-80.0024038110911,37.313811727788));
#23627=CARTESIAN_POINT('Ctrl Pts',(-150.,-80.6225774840775,37.3732852754135));
#23628=CARTESIAN_POINT('Ctrl Pts',(-150.289855072464,-79.4541343310581,
37.5));
#23629=CARTESIAN_POINT('Ctrl Pts',(-150.,-80.0024038100394,37.5));
#23630=CARTESIAN_POINT('Ctrl Pts',(-150.,-80.6225774829855,37.5));
#23631=CARTESIAN_POINT('Origin',(-152.5,-80.6225774829854,37.5));
#23632=CARTESIAN_POINT('Origin',(-121.449578014911,-122.5,115.));
#23633=CARTESIAN_POINT('Origin',(-115.217186218029,-122.5,49.5));
#23634=CARTESIAN_POINT('Origin',(-147.5,0.,44.5));
#23635=CARTESIAN_POINT('Ctrl Pts',(-150.,-80.6225774829854,44.5));
#23636=CARTESIAN_POINT('Ctrl Pts',(-150.,-80.6225774829854,44.5312343888304));
#23637=CARTESIAN_POINT('Ctrl Pts',(-149.999418286665,-80.6247797743348,
44.5621210164789));
#23638=CARTESIAN_POINT('Ctrl Pts',(-149.998293554945,-80.6290354954265,
44.5925723355625));
#23639=CARTESIAN_POINT('Ctrl Pts',(-149.997125538082,-80.6334549973542,
44.6241955694378));
#23640=CARTESIAN_POINT('Ctrl Pts',(-149.995371936956,-80.6400888791781,
44.655349356458));
#23641=CARTESIAN_POINT('Ctrl Pts',(-149.993090530187,-80.6487160556979,
44.6859412124329));
#23642=CARTESIAN_POINT('Ctrl Pts',(-149.992231155702,-80.6519657941861,
44.6974647429366));
#23643=CARTESIAN_POINT('Ctrl Pts',(-149.991297028852,-80.6554978429527,
44.7089085934095));
#23644=CARTESIAN_POINT('Ctrl Pts',(-149.990291719683,-80.6592985775913,
44.7202680068894));
#23645=CARTESIAN_POINT('Ctrl Pts',(-149.987499102739,-80.6698565196466,
44.7518229668389));
#23646=CARTESIAN_POINT('Ctrl Pts',(-149.984157100677,-80.6824881297728,
44.7827141728588));
#23647=CARTESIAN_POINT('Ctrl Pts',(-149.980355786964,-80.6968505802923,
44.8128256266941));
#23648=CARTESIAN_POINT('Ctrl Pts',(-149.977558137322,-80.7074209008703,
44.8349867279405));
#23649=CARTESIAN_POINT('Ctrl Pts',(-149.974509955706,-80.7189351701335,
44.8567449506927));
#23650=CARTESIAN_POINT('Ctrl Pts',(-149.971243495187,-80.7312708109915,
44.8780946805967));
#23651=CARTESIAN_POINT('Ctrl Pts',(-149.965898079908,-80.7514575307578,
44.9130325504344));
#23652=CARTESIAN_POINT('Ctrl Pts',(-149.960009186179,-80.773686648641,44.9465704967713));
#23653=CARTESIAN_POINT('Ctrl Pts',(-149.953740444404,-80.797335293561,44.9787015735967));
#23654=CARTESIAN_POINT('Ctrl Pts',(-149.948225014278,-80.8181420923231,
45.0069714745479));
#23655=CARTESIAN_POINT('Ctrl Pts',(-149.9424154207,-80.8400482470994,45.0341525202745));
#23656=CARTESIAN_POINT('Ctrl Pts',(-149.936415096464,-80.8626613647233,
45.0602466352771));
#23657=CARTESIAN_POINT('Ctrl Pts',(-149.930229230798,-80.8859737229195,
45.0871476299065));
#23658=CARTESIAN_POINT('Ctrl Pts',(-149.923781601043,-80.9102578633712,
45.1131530185116));
#23659=CARTESIAN_POINT('Ctrl Pts',(-149.917129634266,-80.9352949903539,
45.1383421170535));
#23660=CARTESIAN_POINT('Ctrl Pts',(-149.910169623638,-80.9614915538295,
45.1646976896917));
#23661=CARTESIAN_POINT('Ctrl Pts',(-149.902985851619,-80.9885126935503,
45.1901596664586));
#23662=CARTESIAN_POINT('Ctrl Pts',(-149.895629953764,-81.0161619977713,
45.2148125956205));
#23663=CARTESIAN_POINT('Ctrl Pts',(-149.894768894784,-81.0193985410376,
45.2176983923565));
#23664=CARTESIAN_POINT('Ctrl Pts',(-149.893905462669,-81.0226437475977,
45.2205730959881));
#23665=CARTESIAN_POINT('Ctrl Pts',(-149.893039728921,-81.0258973457795,
45.2234368363464));
#23666=CARTESIAN_POINT('Ctrl Pts',(-149.885294621979,-81.055004985282,45.2490566939069));
#23667=CARTESIAN_POINT('Ctrl Pts',(-149.877335285324,-81.0848961910411,
45.2738874208924));
#23668=CARTESIAN_POINT('Ctrl Pts',(-149.869211724912,-81.1153826082176,
45.2979942587922));
#23669=CARTESIAN_POINT('Ctrl Pts',(-149.860756318493,-81.1471143901477,
45.3230858567598));
#23670=CARTESIAN_POINT('Ctrl Pts',(-149.852122887,-81.179491428094,45.3473933229362));
#23671=CARTESIAN_POINT('Ctrl Pts',(-149.843353240441,-81.212356779593,45.3709861423032));
#23672=CARTESIAN_POINT('Ctrl Pts',(-149.834033859779,-81.2472823286657,
45.3960579012523));
#23673=CARTESIAN_POINT('Ctrl Pts',(-149.824560562659,-81.282759673792,45.420322766943));
#23674=CARTESIAN_POINT('Ctrl Pts',(-149.814968902639,-81.318656015993,45.4438574826091));
#23675=CARTESIAN_POINT('Ctrl Pts',(-149.814245534136,-81.3213631890219,
45.4456323862228));
#23676=CARTESIAN_POINT('Ctrl Pts',(-149.813521486337,-81.3240727682655,
45.4474031333746));
#23677=CARTESIAN_POINT('Ctrl Pts',(-149.81279677161,-81.3267847076918,45.4491697551619));
#23678=CARTESIAN_POINT('Ctrl Pts',(-149.802161746897,-81.3665818053887,
45.4750945303171));
#23679=CARTESIAN_POINT('Ctrl Pts',(-149.791378236576,-81.4068954418303,
45.5001449499175));
#23680=CARTESIAN_POINT('Ctrl Pts',(-149.780505488345,-81.4474999785173,
45.5243508763432));
#23681=CARTESIAN_POINT('Ctrl Pts',(-149.766212096436,-81.5008789903218,
45.5561721588362));
#23682=CARTESIAN_POINT('Ctrl Pts',(-149.75173104415,-81.5548874755347,45.5866585651915));
#23683=CARTESIAN_POINT('Ctrl Pts',(-149.7370901728,-81.6094178533078,45.6160154789332));
#23684=CARTESIAN_POINT('Ctrl Pts',(-149.721679195218,-81.6668165155371,
45.6469165591158));
#23685=CARTESIAN_POINT('Ctrl Pts',(-149.706091100881,-81.7247936014321,
45.6765660851853));
#23686=CARTESIAN_POINT('Ctrl Pts',(-149.690345642873,-81.7832715016962,
45.7051731327433));
#23687=CARTESIAN_POINT('Ctrl Pts',(-149.684002656688,-81.8068290579963,
45.7166973518138));
#23688=CARTESIAN_POINT('Ctrl Pts',(-149.67763399788,-81.8304683944407,45.7280520707485));
#23689=CARTESIAN_POINT('Ctrl Pts',(-149.671240444102,-81.854186356593,45.7392497349255));
#23690=CARTESIAN_POINT('Ctrl Pts',(-149.663115656512,-81.8843266214971,
45.7534794803999));
#23691=CARTESIAN_POINT('Ctrl Pts',(-149.654955183208,-81.9145791058626,
45.7674477491405));
#23692=CARTESIAN_POINT('Ctrl Pts',(-149.646761444289,-81.9449339838539,
45.7811773107384));
#23693=CARTESIAN_POINT('Ctrl Pts',(-149.629599044989,-82.0085145472401,
45.8099349048783));
#23694=CARTESIAN_POINT('Ctrl Pts',(-149.612256027528,-82.0726719053374,
45.8376821506386));
#23695=CARTESIAN_POINT('Ctrl Pts',(-149.594776281623,-82.1372383448953,
45.8645156723128));
#23696=CARTESIAN_POINT('Ctrl Pts',(-149.57592605508,-82.2068670465535,45.8934530473311));
#23697=CARTESIAN_POINT('Ctrl Pts',(-149.556916727547,-82.2769718987423,
45.9213279816653));
#23698=CARTESIAN_POINT('Ctrl Pts',(-149.537787182918,-82.3473991049663,
45.9482460618992));
#23699=CARTESIAN_POINT('Ctrl Pts',(-149.532245072383,-82.3678029028159,
45.9560446257929));
#23700=CARTESIAN_POINT('Ctrl Pts',(-149.526692780135,-82.3882340721267,
45.9637627732937));
#23701=CARTESIAN_POINT('Ctrl Pts',(-149.521131044556,-82.4086895813368,
45.9714028195526));
#23702=CARTESIAN_POINT('Ctrl Pts',(-149.513307047732,-82.4374654619684,
45.9821504893812));
#23703=CARTESIAN_POINT('Ctrl Pts',(-149.505462657808,-82.4662967316413,
45.9927459306726));
#23704=CARTESIAN_POINT('Ctrl Pts',(-149.497602582526,-82.4951656239004,
46.0031912460791));
#23705=CARTESIAN_POINT('Ctrl Pts',(-149.466886299739,-82.6079819808148,
46.0440103540796));
#23706=CARTESIAN_POINT('Ctrl Pts',(-149.435949796432,-82.721306238521,46.0825462658463));
#23707=CARTESIAN_POINT('Ctrl Pts',(-149.404819096531,-82.8350358342389,
46.1191658716245));
#23708=CARTESIAN_POINT('Ctrl Pts',(-149.382928718768,-82.9150078175565,
46.1449159192168));
#23709=CARTESIAN_POINT('Ctrl Pts',(-149.360942099001,-82.995181007926,46.169717455523));
#23710=CARTESIAN_POINT('Ctrl Pts',(-149.338865605393,-83.0755291035976,
46.193686300737));
#23711=CARTESIAN_POINT('Ctrl Pts',(-149.30257270251,-83.2076182697843,46.233090156576));
#23712=CARTESIAN_POINT('Ctrl Pts',(-149.266041574139,-83.3401623692395,
46.2702654172594));
#23713=CARTESIAN_POINT('Ctrl Pts',(-149.229255373738,-83.4732146574125,
46.3055170512346));
#23714=CARTESIAN_POINT('Ctrl Pts',(-149.222100057115,-83.4990947765572,
46.3123738779743));
#23715=CARTESIAN_POINT('Ctrl Pts',(-149.214935059986,-83.5249942184406,
46.3191578024711));
#23716=CARTESIAN_POINT('Ctrl Pts',(-149.207760216038,-83.5509135089673,
46.3258708967128));
#23717=CARTESIAN_POINT('Ctrl Pts',(-149.164019348336,-83.7089284102155,
46.366796743915));
#23718=CARTESIAN_POINT('Ctrl Pts',(-149.119950314816,-83.8675446159544,
46.4050588777709));
#23719=CARTESIAN_POINT('Ctrl Pts',(-149.075578120339,-84.0266555943282,
46.4410493230434));
#23720=CARTESIAN_POINT('Ctrl Pts',(-149.050851325548,-84.1153215834145,
46.4611053145304));
#23721=CARTESIAN_POINT('Ctrl Pts',(-149.026030206988,-84.2041418314762,
46.4804550867179));
#23722=CARTESIAN_POINT('Ctrl Pts',(-149.001117827171,-84.2931021083258,
46.4991611413161));
#23723=CARTESIAN_POINT('Ctrl Pts',(-148.961812515426,-84.4334584869728,
46.5286744721549));
#23724=CARTESIAN_POINT('Ctrl Pts',(-148.922228706232,-84.5743409203763,
46.5565824640166));
#23725=CARTESIAN_POINT('Ctrl Pts',(-148.882458149795,-84.7154243069172,
46.58297626425));
#23726=CARTESIAN_POINT('Ctrl Pts',(-148.823378480021,-84.9250054803839,
46.6221845917561));
#23727=CARTESIAN_POINT('Ctrl Pts',(-148.763691428381,-85.1357176965639,
46.658180607518));
#23728=CARTESIAN_POINT('Ctrl Pts',(-148.703725142332,-85.346373256235,46.6911268937745));
#23729=CARTESIAN_POINT('Ctrl Pts',(-148.683093735236,-85.4188493239555,
46.7024620670668));
#23730=CARTESIAN_POINT('Ctrl Pts',(-148.662429146923,-85.4913191022908,
46.7134360383522));
#23731=CARTESIAN_POINT('Ctrl Pts',(-148.64174438629,-85.5637353575988,46.7240548006858));
#23732=CARTESIAN_POINT('Ctrl Pts',(-148.565624143843,-85.8302283090543,
46.7631320120529));
#23733=CARTESIAN_POINT('Ctrl Pts',(-148.489028565031,-86.0967324995911,
46.7975654258511));
#23734=CARTESIAN_POINT('Ctrl Pts',(-148.411875341988,-86.3635238183437,
46.8277812265461));
#23735=CARTESIAN_POINT('Ctrl Pts',(-148.365096720961,-86.5252815453832,
46.846101310063));
#23736=CARTESIAN_POINT('Ctrl Pts',(-148.318112978006,-86.6871449972432,
46.8628698580675));
#23737=CARTESIAN_POINT('Ctrl Pts',(-148.270904619886,-86.8491769961467,
46.8781728422293));
#23738=CARTESIAN_POINT('Ctrl Pts',(-148.24918654488,-86.9237193705385,46.8852129379044));
#23739=CARTESIAN_POINT('Ctrl Pts',(-148.227421070419,-86.9982969676292,
46.8919477958447));
#23740=CARTESIAN_POINT('Ctrl Pts',(-148.205605817643,-87.0729174681581,
46.8983780579096));
#23741=CARTESIAN_POINT('Ctrl Pts',(-148.10190068443,-87.42764766667,46.9289461742125));
#23742=CARTESIAN_POINT('Ctrl Pts',(-147.997167488693,-87.7829762387816,
46.9525973445083));
#23743=CARTESIAN_POINT('Ctrl Pts',(-147.891499227195,-88.1385323929249,
46.969351029831));
#23744=CARTESIAN_POINT('Ctrl Pts',(-147.785745335364,-88.4943766789206,
46.9861182918287));
#23745=CARTESIAN_POINT('Ctrl Pts',(-147.679054863979,-88.8504488649393,
46.9959768816863));
#23746=CARTESIAN_POINT('Ctrl Pts',(-147.571529965735,-89.2063722196095,
46.9989975290796));
#23747=CARTESIAN_POINT('Ctrl Pts',(-147.547727111398,-89.285163196442,46.9996662116924));
#23748=CARTESIAN_POINT('Ctrl Pts',(-147.523883400528,-89.3639468619846,
47.));
#23749=CARTESIAN_POINT('Ctrl Pts',(-147.5,-89.4427190999916,47.));
#23750=CARTESIAN_POINT('Origin',(-152.5,-80.6225774829854,115.));
#23751=CARTESIAN_POINT('Origin',(-152.5,-80.6225774829854,44.5));
#23752=CARTESIAN_POINT('Ctrl Pts',(-150.289855072464,-79.4541343310581,
44.5));
#23753=CARTESIAN_POINT('Ctrl Pts',(-150.,-80.0024038100394,44.5));
#23754=CARTESIAN_POINT('Ctrl Pts',(-150.,-80.6225774829855,44.5));
#23755=CARTESIAN_POINT('Ctrl Pts',(-150.28985506853,-79.4541343384987,44.7594238560556));
#23756=CARTESIAN_POINT('Ctrl Pts',(-149.999999996126,-80.0024038172978,
44.6905851824362));
#23757=CARTESIAN_POINT('Ctrl Pts',(-150.,-80.6225774905387,44.629711927975));
#23758=CARTESIAN_POINT('Ctrl Pts',(-150.270119749701,-79.4914922605508,
45.0111695802387));
#23759=CARTESIAN_POINT('Ctrl Pts',(-149.980519833119,-80.0389466368966,
44.8758156770736));
#23760=CARTESIAN_POINT('Ctrl Pts',(-149.989987226484,-80.6604847938369,
44.7555847901951));
#23761=CARTESIAN_POINT('Ctrl Pts',(-150.196231486305,-79.6310132970258,
45.5012087006257));
#23762=CARTESIAN_POINT('Ctrl Pts',(-149.907890955038,-80.1748646486434,
45.2336047942099));
#23763=CARTESIAN_POINT('Ctrl Pts',(-149.952499797667,-80.8020576101747,
45.0006043502371));
#23764=CARTESIAN_POINT('Ctrl Pts',(-150.143050717941,-79.7313168859281,
45.7320003431406));
#23765=CARTESIAN_POINT('Ctrl Pts',(-149.855501091412,-80.272795283317,45.4011397919881));
#23766=CARTESIAN_POINT('Ctrl Pts',(-149.925518380098,-80.9038362519448,
45.1160001719023));
#23767=CARTESIAN_POINT('Ctrl Pts',(-150.01502846971,-79.971931353987,46.1617150079383));
#23768=CARTESIAN_POINT('Ctrl Pts',(-149.729850869406,-80.506872138187,45.7093793927994));
#23769=CARTESIAN_POINT('Ctrl Pts',(-149.860565913637,-81.1479891679691,
45.3308575036371));
#23770=CARTESIAN_POINT('Ctrl Pts',(-149.939105635844,-80.1142600764838,
46.3637363656926));
#23771=CARTESIAN_POINT('Ctrl Pts',(-149.655266820466,-80.6454659182033,
45.8524984192499));
#23772=CARTESIAN_POINT('Ctrl Pts',(-149.8220462428,-81.2924109599909,45.4318681833206));
#23773=CARTESIAN_POINT('Ctrl Pts',(-149.775363670977,-80.4199633406152,
46.7336380224264));
#23774=CARTESIAN_POINT('Ctrl Pts',(-149.494928348598,-80.9422362487695,
46.1103934277676));
#23775=CARTESIAN_POINT('Ctrl Pts',(-149.738971273161,-81.6026098603007,
45.616819010739));
#23776=CARTESIAN_POINT('Ctrl Pts',(-149.686995608736,-80.5843780010491,
46.903585266663));
#23777=CARTESIAN_POINT('Ctrl Pts',(-149.408398325687,-81.1018541496878,
46.2266925752405));
#23778=CARTESIAN_POINT('Ctrl Pts',(-149.694137478568,-81.7694423834459,
45.7017926336777));
#23779=CARTESIAN_POINT('Ctrl Pts',(-149.500255462679,-80.9302925286903,
47.2210941330543));
#23780=CARTESIAN_POINT('Ctrl Pts',(-149.226078269656,-81.4367533718067,
46.4395269094013));
#23781=CARTESIAN_POINT('Ctrl Pts',(-149.599394315017,-82.1204438893779,
45.8605470661809));
#23782=CARTESIAN_POINT('Ctrl Pts',(-149.401347886678,-81.1127763961003,
47.369210707149));
#23783=CARTESIAN_POINT('Ctrl Pts',(-149.129574349821,-81.6133256610688,
46.5363235480013));
#23784=CARTESIAN_POINT('Ctrl Pts',(-149.549213266548,-82.3056113431187,
45.9346053539496));
#23785=CARTESIAN_POINT('Ctrl Pts',(-149.197899201605,-81.4863922312653,
47.6435514113241));
#23786=CARTESIAN_POINT('Ctrl Pts',(-148.93165319989,-81.9738530462045,46.7107456147876));
#23787=CARTESIAN_POINT('Ctrl Pts',(-149.445992976772,-82.684721528767,46.071775705287));
#23788=CARTESIAN_POINT('Ctrl Pts',(-149.093462145135,-81.6773447374821,
47.7698090460946));
#23789=CARTESIAN_POINT('Ctrl Pts',(-148.830186520417,-82.1578926315274,
46.7883037911384));
#23790=CARTESIAN_POINT('Ctrl Pts',(-149.393006529828,-82.8784821601051,
46.1349045233201));
#23791=CARTESIAN_POINT('Ctrl Pts',(-148.773324875584,-82.2599185303359,
48.1224993059861));
#23792=CARTESIAN_POINT('Ctrl Pts',(-148.518202139789,-82.721231742148,46.9985052310704));
#23793=CARTESIAN_POINT('Ctrl Pts',(-149.230583943609,-83.4696232145796,
46.3112496524474));
#23794=CARTESIAN_POINT('Ctrl Pts',(-148.550873607932,-82.6611103319713,
48.3232112727545));
#23795=CARTESIAN_POINT('Ctrl Pts',(-148.30315471628,-83.1060920248234,47.1056075630378));
#23796=CARTESIAN_POINT('Ctrl Pts',(-149.117722639557,-83.8767148956951,
46.4116056366651));
#23797=CARTESIAN_POINT('Ctrl Pts',(-148.091214058598,-83.4818155626998,
48.6734332925097));
#23798=CARTESIAN_POINT('Ctrl Pts',(-147.862495369544,-83.8874214153556,
47.2694844772005));
#23799=CARTESIAN_POINT('Ctrl Pts',(-148.884513014786,-84.7094893209564,
46.586716645967));
#23800=CARTESIAN_POINT('Ctrl Pts',(-147.853104568995,-83.9028862659541,
48.8228865658125));
#23801=CARTESIAN_POINT('Ctrl Pts',(-147.635229789707,-84.286581928446,47.3247069198698));
#23802=CARTESIAN_POINT('Ctrl Pts',(-148.763707465283,-85.1367522404598,
46.6614432831528));
#23803=CARTESIAN_POINT('Ctrl Pts',(-147.37234266623,-84.7444834282146,49.073322172108));
#23804=CARTESIAN_POINT('Ctrl Pts',(-147.180928816256,-85.0771956930355,
47.3874171310308));
#23805=CARTESIAN_POINT('Ctrl Pts',(-148.519791499647,-85.9907258315643,
46.7866610858075));
#23806=CARTESIAN_POINT('Ctrl Pts',(-147.128665473946,-85.166872640511,49.1751382031672));
#23807=CARTESIAN_POINT('Ctrl Pts',(-146.952267516978,-85.4713149459694,
47.3939268980417));
#23808=CARTESIAN_POINT('Ctrl Pts',(-148.396161159612,-86.4193266499342,
46.837569101695));
#23809=CARTESIAN_POINT('Ctrl Pts',(-146.388097896077,-86.4377602232181,
49.41873440213));
#23810=CARTESIAN_POINT('Ctrl Pts',(-146.253862108763,-86.6644852388405,
47.3459550909554));
#23811=CARTESIAN_POINT('Ctrl Pts',(-148.020432020732,-87.7089037559046,
46.9593672008422));
#23812=CARTESIAN_POINT('Ctrl Pts',(-145.881711078451,-87.289917999924,49.4999999990937));
#23813=CARTESIAN_POINT('Ctrl Pts',(-145.791767290438,-87.4382443129923,
47.2157310733627));
#23814=CARTESIAN_POINT('Ctrl Pts',(-147.763515165397,-88.573593311031,47.));
#23815=CARTESIAN_POINT('Ctrl Pts',(-145.36231884058,-88.1464478086874,49.5));
#23816=CARTESIAN_POINT('Ctrl Pts',(-145.36231884058,-88.1464478086874,46.9999999999999));
#23817=CARTESIAN_POINT('Ctrl Pts',(-147.5,-89.4427190999917,47.));
#23818=CARTESIAN_POINT('Origin',(-147.5,-89.4427190999916,49.5));
#23819=CARTESIAN_POINT('Origin',(0.,0.,49.5));
#23820=CARTESIAN_POINT('Origin',(177.5,-137.5,-73.9644660940671));
#23821=CARTESIAN_POINT('Origin',(177.5,-137.5,-73.9644660940671));
#23822=CARTESIAN_POINT('Origin',(177.5,-137.5,-73.9644660940672));
#23823=CARTESIAN_POINT('Origin',(177.5,-137.5,-73.9644660940672));
#23824=CARTESIAN_POINT('Origin',(225.840826156048,-127.5,-25.623639938019));
#23825=CARTESIAN_POINT('Origin',(177.5,-127.5,-73.9644660940672));
#23826=CARTESIAN_POINT('Origin',(168.964466094067,-127.5,-82.5));
#23827=CARTESIAN_POINT('Origin',(177.5,-125.,-73.9644660940672));
#23828=CARTESIAN_POINT('Origin',(177.5,-127.5,-73.9644660940672));
#23829=CARTESIAN_POINT('Origin',(177.5,-137.5,85.));
#23830=CARTESIAN_POINT('Origin',(177.5,-137.5,73.9644660940673));
#23831=CARTESIAN_POINT('Origin',(258.232233047034,-137.5,6.76776695296642));
#23832=CARTESIAN_POINT('Origin',(168.964466094067,-137.5,-82.5));
#23833=CARTESIAN_POINT('Origin',(168.964466094067,0.,-82.5));
#23834=CARTESIAN_POINT('Origin',(168.964466094067,-127.5,-82.5));
#23835=CARTESIAN_POINT('Origin',(168.964466094067,-137.5,-82.5));
#23836=CARTESIAN_POINT('Origin',(168.964466094067,-127.5,-82.5));
#23837=CARTESIAN_POINT('Origin',(168.964466094067,-127.5,-82.5));
#23838=CARTESIAN_POINT('Origin',(177.5,-127.5,-73.9644660940671));
#23839=CARTESIAN_POINT('Origin',(177.5,-127.5,-73.9644660940672));
#23840=CARTESIAN_POINT('Origin',(177.5,-137.5,73.9644660940673));
#23841=CARTESIAN_POINT('Origin',(177.5,-137.5,73.9644660940673));
#23842=CARTESIAN_POINT('Origin',(177.5,-137.5,73.9644660940673));
#23843=CARTESIAN_POINT('Origin',(168.964466094067,-137.5,-82.5));
#23844=CARTESIAN_POINT('Origin',(168.964466094067,-137.5,-82.5));
#23845=CARTESIAN_POINT('Origin',(0.,-127.5,-82.5));
#23846=CARTESIAN_POINT('Ctrl Pts',(121.449578014911,-125.,-82.5));
#23847=CARTESIAN_POINT('Ctrl Pts',(121.449578013665,-125.,-82.5578430303792));
#23848=CARTESIAN_POINT('Ctrl Pts',(121.445542821646,-125.002000739817,-82.6149744276235));
#23849=CARTESIAN_POINT('Ctrl Pts',(121.437730668305,-125.005872173715,-82.6713216462809));
#23850=CARTESIAN_POINT('Ctrl Pts',(121.431548654752,-125.008935766528,-82.7159110513097));
#23851=CARTESIAN_POINT('Ctrl Pts',(121.423002583493,-125.013170255242,-82.7600095425404));
#23852=CARTESIAN_POINT('Ctrl Pts',(121.412240896123,-125.018501093781,-82.8035838902947));
#23853=CARTESIAN_POINT('Ctrl Pts',(121.402625881463,-125.023263924083,-82.8425153308796));
#23854=CARTESIAN_POINT('Ctrl Pts',(121.391240873519,-125.02890257476,-82.8810286286793));
#23855=CARTESIAN_POINT('Ctrl Pts',(121.378166904503,-125.035375090082,-82.9190974411551));
#23856=CARTESIAN_POINT('Ctrl Pts',(121.359482649641,-125.044625083389,-82.9735022966163));
#23857=CARTESIAN_POINT('Ctrl Pts',(121.337601423089,-125.055455126064,-83.0262941391226));
#23858=CARTESIAN_POINT('Ctrl Pts',(121.312984159938,-125.067631742438,-83.0775690600158));
#23859=CARTESIAN_POINT('Ctrl Pts',(121.309754155106,-125.069229423281,-83.0842967876764));
#23860=CARTESIAN_POINT('Ctrl Pts',(121.306476982697,-125.070850319854,-83.0909983906632));
#23861=CARTESIAN_POINT('Ctrl Pts',(121.303153626062,-125.072493934659,-83.0976740773907));
#23862=CARTESIAN_POINT('Ctrl Pts',(121.28333698938,-125.082294543202,-83.1374801147826));
#23863=CARTESIAN_POINT('Ctrl Pts',(121.26193952168,-125.092872330006,-83.1761870718699));
#23864=CARTESIAN_POINT('Ctrl Pts',(121.239293756531,-125.104060083144,-83.2137354525193));
#23865=CARTESIAN_POINT('Ctrl Pts',(121.223112895711,-125.112053960817,-83.2405645358963));
#23866=CARTESIAN_POINT('Ctrl Pts',(121.206293748506,-125.120359745354,-83.2668025986261));
#23867=CARTESIAN_POINT('Ctrl Pts',(121.188944294236,-125.128923152136,-83.2924342403753));
#23868=CARTESIAN_POINT('Ctrl Pts',(121.169248714547,-125.138644568041,-83.3215319880497));
#23869=CARTESIAN_POINT('Ctrl Pts',(121.148816846868,-125.14872481678,-83.3499289055538));
#23870=CARTESIAN_POINT('Ctrl Pts',(121.127768696513,-125.159103720469,-83.3776130175157));
#23871=CARTESIAN_POINT('Ctrl Pts',(121.095198113589,-125.175164368915,-83.4204523002619));
#23872=CARTESIAN_POINT('Ctrl Pts',(121.061072412821,-125.191979398504,-83.4617485539168));
#23873=CARTESIAN_POINT('Ctrl Pts',(121.025604781293,-125.209440222843,-83.5016773345161));
#23874=CARTESIAN_POINT('Ctrl Pts',(120.994690465974,-125.224659435574,-83.5364800788934));
#23875=CARTESIAN_POINT('Ctrl Pts',(120.962755773204,-125.240369726302,-83.5702435568605));
#23876=CARTESIAN_POINT('Ctrl Pts',(120.929914941896,-125.256512858459,-83.6030728931431));
#23877=CARTESIAN_POINT('Ctrl Pts',(120.919024936224,-125.261865914206,-83.6139590870702));
#23878=CARTESIAN_POINT('Ctrl Pts',(120.908034223584,-125.267267022157,-83.6247432148631));
#23879=CARTESIAN_POINT('Ctrl Pts',(120.896946618515,-125.272714234811,-83.6354286063845));
#23880=CARTESIAN_POINT('Ctrl Pts',(120.861818540488,-125.289972254912,-83.6692823795651));
#23881=CARTESIAN_POINT('Ctrl Pts',(120.825696080647,-125.307703371905,-83.7021357945807));
#23882=CARTESIAN_POINT('Ctrl Pts',(120.788855644392,-125.325770196085,-83.7339645608892));
#23883=CARTESIAN_POINT('Ctrl Pts',(120.750104876467,-125.344773861135,-83.7674437826887));
#23884=CARTESIAN_POINT('Ctrl Pts',(120.710559563373,-125.364149043197,-83.7997894992637));
#23885=CARTESIAN_POINT('Ctrl Pts',(120.670490053903,-125.383761285266,-83.8309820047469));
#23886=CARTESIAN_POINT('Ctrl Pts',(120.655933159391,-125.390886237448,-83.8423139630833));
#23887=CARTESIAN_POINT('Ctrl Pts',(120.641306624739,-125.398042702867,-83.8534937861162));
#23888=CARTESIAN_POINT('Ctrl Pts',(120.62662193437,-125.405224965794,-83.8645207217808));
#23889=CARTESIAN_POINT('Ctrl Pts',(120.623763587428,-125.406622979559,-83.8666670937534));
#23890=CARTESIAN_POINT('Ctrl Pts',(120.62090288229,-125.40802204969,-83.8688077929118));
#23891=CARTESIAN_POINT('Ctrl Pts',(120.618039908549,-125.409422131597,-83.8709428055742));
#23892=CARTESIAN_POINT('Ctrl Pts',(120.561761358575,-125.436944067424,-83.9129115512497));
#23893=CARTESIAN_POINT('Ctrl Pts',(120.504422162933,-125.464947521896,-83.9528770557978));
#23894=CARTESIAN_POINT('Ctrl Pts',(120.446193115433,-125.493345150898,-83.9910922510515));
#23895=CARTESIAN_POINT('Ctrl Pts',(120.399258153871,-125.516234785589,-84.0218952402353));
#23896=CARTESIAN_POINT('Ctrl Pts',(120.351744177111,-125.539380959607,-84.0515603444805));
#23897=CARTESIAN_POINT('Ctrl Pts',(120.303722804547,-125.562746846771,-84.0802057525297));
#23898=CARTESIAN_POINT('Ctrl Pts',(120.237604852662,-125.594918034739,-84.1196460186027));
#23899=CARTESIAN_POINT('Ctrl Pts',(120.170523556422,-125.627506495568,-84.157152051961));
#23900=CARTESIAN_POINT('Ctrl Pts',(120.102573990086,-125.660461610429,-84.1929593090859));
#23901=CARTESIAN_POINT('Ctrl Pts',(120.054961757024,-125.683553245799,-84.2180494393614));
#23902=CARTESIAN_POINT('Ctrl Pts',(120.006922336468,-125.706825340362,-84.24230479924));
#23903=CARTESIAN_POINT('Ctrl Pts',(119.958477373249,-125.73026591296,-84.2657976274669));
#23904=CARTESIAN_POINT('Ctrl Pts',(119.957432170273,-125.730771644714,-84.2663044866393));
#23905=CARTESIAN_POINT('Ctrl Pts',(119.956386759699,-125.731277463805,-84.2668109935507));
#23906=CARTESIAN_POINT('Ctrl Pts',(119.955341143413,-125.731783369317,-84.2673171481935));
#23907=CARTESIAN_POINT('Ctrl Pts',(119.89298150186,-125.761955131908,-84.2975037687741));
#23908=CARTESIAN_POINT('Ctrl Pts',(119.829839678401,-125.792457959603,-84.3264634103549));
#23909=CARTESIAN_POINT('Ctrl Pts',(119.766290102992,-125.823110100769,-84.3541852883539));
#23910=CARTESIAN_POINT('Ctrl Pts',(119.706671564982,-125.85186616769,-84.3801923517616));
#23911=CARTESIAN_POINT('Ctrl Pts',(119.646693089753,-125.880754168446,-84.4051101569439));
#23912=CARTESIAN_POINT('Ctrl Pts',(119.586626434295,-125.909641987124,-84.4289275235297));
#23913=CARTESIAN_POINT('Ctrl Pts',(119.501128626528,-125.950760393823,-84.4628287390101));
#23914=CARTESIAN_POINT('Ctrl Pts',(119.415197450966,-125.99200199476,-84.4946555586855));
#23915=CARTESIAN_POINT('Ctrl Pts',(119.328730569191,-126.033415379519,-84.5246645405908));
#23916=CARTESIAN_POINT('Ctrl Pts',(119.297298692445,-126.048469702963,-84.5355732099122));
#23917=CARTESIAN_POINT('Ctrl Pts',(119.265795758865,-126.063546844264,-84.5462412487785));
#23918=CARTESIAN_POINT('Ctrl Pts',(119.2342159707,-126.078649522118,-84.5566796096831));
#23919=CARTESIAN_POINT('Ctrl Pts',(119.1303530696,-126.12832078426,-84.5910103797511));
#23920=CARTESIAN_POINT('Ctrl Pts',(119.025943929888,-126.178130418089,-84.6227652061912));
#23921=CARTESIAN_POINT('Ctrl Pts',(118.920995425667,-126.22807113596,-84.6522643594006));
#23922=CARTESIAN_POINT('Ctrl Pts',(118.879152593278,-126.247982435342,-84.6640256334897));
#23923=CARTESIAN_POINT('Ctrl Pts',(118.8372237143,-126.267914711427,-84.6754278512292));
#23924=CARTESIAN_POINT('Ctrl Pts',(118.795208048995,-126.287868028778,-84.686489443114));
#23925=CARTESIAN_POINT('Ctrl Pts',(118.687953257482,-126.338803528117,-84.7147267380079));
#23926=CARTESIAN_POINT('Ctrl Pts',(118.579924099557,-126.389974247259,-84.7407679174261));
#23927=CARTESIAN_POINT('Ctrl Pts',(118.471295931363,-126.441294374164,-84.7647575879222));
#23928=CARTESIAN_POINT('Ctrl Pts',(118.355734714612,-126.495889940006,-84.7902783672747));
#23929=CARTESIAN_POINT('Ctrl Pts',(118.23949519911,-126.550654804836,-84.8134776148356));
#23930=CARTESIAN_POINT('Ctrl Pts',(118.122742883492,-126.605505675963,-84.8344961205875));
#23931=CARTESIAN_POINT('Ctrl Pts',(118.065228912499,-126.632526051483,-84.8448501570254));
#23932=CARTESIAN_POINT('Ctrl Pts',(118.007589863374,-126.659567573598,-84.854674480348));
#23933=CARTESIAN_POINT('Ctrl Pts',(117.949842319793,-126.686621640133,-84.8639830042662));
#23934=CARTESIAN_POINT('Ctrl Pts',(117.876606796367,-126.720931648848,-84.8757880885902));
#23935=CARTESIAN_POINT('Ctrl Pts',(117.803387560177,-126.755173054075,-84.8867590613586));
#23936=CARTESIAN_POINT('Ctrl Pts',(117.730135337143,-126.789368961517,-84.896927988525));
#23937=CARTESIAN_POINT('Ctrl Pts',(117.430682221293,-126.929160910605,-84.9384982890397));
#23938=CARTESIAN_POINT('Ctrl Pts',(117.129946638445,-127.068588179086,-84.9667803784096));
#23939=CARTESIAN_POINT('Ctrl Pts',(116.828007611095,-127.20757466619,-84.9830546227486));
#23940=CARTESIAN_POINT('Ctrl Pts',(116.615757672273,-127.305276091686,-84.9944947051906));
#23941=CARTESIAN_POINT('Ctrl Pts',(116.402913050166,-127.402759565481,-85.));
#23942=CARTESIAN_POINT('Ctrl Pts',(116.189500386222,-127.5,-85.));
#23943=CARTESIAN_POINT('Origin',(177.5,-127.5,85.));
#23944=CARTESIAN_POINT('Origin',(177.5,-127.5,73.9644660940673));
#23945=CARTESIAN_POINT('Origin',(177.5,-125.,73.9644660940673));
#23946=CARTESIAN_POINT('Origin',(177.5,-127.5,73.9644660940673));
#23947=CARTESIAN_POINT('Origin',(173.232233047034,-137.5,78.2322330470336));
#23948=CARTESIAN_POINT('Origin',(168.964466094067,-137.5,82.5));
#23949=CARTESIAN_POINT('Origin',(0.,-137.5,-82.5));
#23950=CARTESIAN_POINT('Ctrl Pts',(104.163333279998,-137.5,-85.));
#23951=CARTESIAN_POINT('Ctrl Pts',(103.738099080441,-137.661068405961,-85.));
#23952=CARTESIAN_POINT('Ctrl Pts',(103.313784132472,-137.820236149174,-84.9848502161634));
#23953=CARTESIAN_POINT('Ctrl Pts',(102.890445132596,-137.977529707376,-84.9541805579568));
#23954=CARTESIAN_POINT('Ctrl Pts',(102.674532847161,-138.057752913,-84.9385383515953));
#23955=CARTESIAN_POINT('Ctrl Pts',(102.458874713662,-138.137488523029,-84.9188583125581));
#23956=CARTESIAN_POINT('Ctrl Pts',(102.243480097268,-138.216739650426,-84.8950864427477));
#23957=CARTESIAN_POINT('Ctrl Pts',(102.169808729557,-138.243845894054,-84.8869557559584));
#23958=CARTESIAN_POINT('Ctrl Pts',(102.096197177396,-138.270885582569,-84.8783493800412));
#23959=CARTESIAN_POINT('Ctrl Pts',(102.022632569934,-138.297863659494,-84.8692643545073));
#23960=CARTESIAN_POINT('Ctrl Pts',(101.824799549342,-138.370414232822,-84.8448325236913));
#23961=CARTESIAN_POINT('Ctrl Pts',(101.627311999894,-138.442516995573,-84.8168822159707));
#23962=CARTESIAN_POINT('Ctrl Pts',(101.42999704102,-138.514238577898,-84.7850438375703));
#23963=CARTESIAN_POINT('Ctrl Pts',(101.276966125295,-138.569863450352,-84.7603510508216));
#23964=CARTESIAN_POINT('Ctrl Pts',(101.124039180306,-138.625258921571,-84.7333188027895));
#23965=CARTESIAN_POINT('Ctrl Pts',(100.971140292634,-138.680453268945,-84.7037536341508));
#23966=CARTESIAN_POINT('Ctrl Pts',(100.819413206494,-138.735224612453,-84.6744150499591));
#23967=CARTESIAN_POINT('Ctrl Pts',(100.667483749192,-138.789877248555,-84.6424995110724));
#23968=CARTESIAN_POINT('Ctrl Pts',(100.516166836934,-138.844125833747,-84.6079054671296));
#23969=CARTESIAN_POINT('Ctrl Pts',(100.456828089701,-138.865399351931,-84.5943394539282));
#23970=CARTESIAN_POINT('Ctrl Pts',(100.397584005817,-138.886610562357,-84.5803613497262));
#23971=CARTESIAN_POINT('Ctrl Pts',(100.338485741259,-138.907741516914,-84.565964289852));
#23972=CARTESIAN_POINT('Ctrl Pts',(100.220918177777,-138.949778535426,-84.5373233938226));
#23973=CARTESIAN_POINT('Ctrl Pts',(100.103632370179,-138.991604254091,-84.5069540658058));
#23974=CARTESIAN_POINT('Ctrl Pts',(99.9869935660692,-139.033088789031,-84.4747498712919));
#23975=CARTESIAN_POINT('Ctrl Pts',(99.9720326094956,-139.038409902621,-84.4706191228734));
#23976=CARTESIAN_POINT('Ctrl Pts',(99.9570823608136,-139.043725379489,-84.4664581642972));
#23977=CARTESIAN_POINT('Ctrl Pts',(99.9421436485644,-139.049034924161,-84.4622667514209));
#23978=CARTESIAN_POINT('Ctrl Pts',(99.8232112700053,-139.0913060896,-84.4288974291803));
#23979=CARTESIAN_POINT('Ctrl Pts',(99.7047475328351,-139.133296386698,-84.3935836754955));
#23980=CARTESIAN_POINT('Ctrl Pts',(99.5868591110941,-139.174972397689,-84.3559924242641));
#23981=CARTESIAN_POINT('Ctrl Pts',(99.5255437217676,-139.196648664126,-84.336440697551));
#23982=CARTESIAN_POINT('Ctrl Pts',(99.4643844621158,-139.218239730484,-84.3162722626081));
#23983=CARTESIAN_POINT('Ctrl Pts',(99.4033998553792,-139.239739634851,-84.2954359997591));
#23984=CARTESIAN_POINT('Ctrl Pts',(99.3132315996693,-139.271528129989,-84.2646287259707));
#23985=CARTESIAN_POINT('Ctrl Pts',(99.223535776852,-139.303085592255,-84.2323955368028));
#23986=CARTESIAN_POINT('Ctrl Pts',(99.1342049110009,-139.334451631701,-84.1984942631106));
#23987=CARTESIAN_POINT('Ctrl Pts',(99.0808040909447,-139.353201838725,-84.1782285263033));
#23988=CARTESIAN_POINT('Ctrl Pts',(99.0275342339471,-139.371883428182,-84.1573660209767));
#23989=CARTESIAN_POINT('Ctrl Pts',(98.9743778992268,-139.390502757733,-84.1358481968094));
#23990=CARTESIAN_POINT('Ctrl Pts',(98.8981671957289,-139.417197453882,-84.1049979034971));
#23991=CARTESIAN_POINT('Ctrl Pts',(98.8224769045325,-139.443662996202,-84.0729177573328));
#23992=CARTESIAN_POINT('Ctrl Pts',(98.7474387368693,-139.46985661819,-84.0394249607335));
#23993=CARTESIAN_POINT('Ctrl Pts',(98.6761330066818,-139.4947473558,-84.0075981132516));
#23994=CARTESIAN_POINT('Ctrl Pts',(98.6054159170073,-139.519392616372,-83.9744956741588));
#23995=CARTESIAN_POINT('Ctrl Pts',(98.5354408951835,-139.543741578814,-83.9399393538181));
#23996=CARTESIAN_POINT('Ctrl Pts',(98.5230520237326,-139.548052490877,-83.9338212591129));
#23997=CARTESIAN_POINT('Ctrl Pts',(98.5106865249416,-139.552354076384,-83.9276575341684));
#23998=CARTESIAN_POINT('Ctrl Pts',(98.4983453996891,-139.556646001529,-83.921447113738));
#23999=CARTESIAN_POINT('Ctrl Pts',(98.4332103940779,-139.579298276965,-83.8886692461367));
#24000=CARTESIAN_POINT('Ctrl Pts',(98.3686986921717,-139.601700795348,-83.8545667766362));
#24001=CARTESIAN_POINT('Ctrl Pts',(98.3049498142096,-139.623806785601,-83.8189431096019));
#24002=CARTESIAN_POINT('Ctrl Pts',(98.2461451146523,-139.644198299252,-83.7860823110428));
#24003=CARTESIAN_POINT('Ctrl Pts',(98.1879895705334,-139.664337465922,-83.7519270259336));
#24004=CARTESIAN_POINT('Ctrl Pts',(98.1306351301536,-139.684172991867,-83.7163018099732));
#24005=CARTESIAN_POINT('Ctrl Pts',(98.1258128865628,-139.685840722163,-83.7133065149586));
#24006=CARTESIAN_POINT('Ctrl Pts',(98.1209963324925,-139.687506296946,-83.710300816007));
#24007=CARTESIAN_POINT('Ctrl Pts',(98.1161855731307,-139.689169680641,-83.7072846016472));
#24008=CARTESIAN_POINT('Ctrl Pts',(98.1011329199801,-139.694374334612,-83.697847000393));
#24009=CARTESIAN_POINT('Ctrl Pts',(98.0861233722941,-139.699562258723,-83.6882946516978));
#24010=CARTESIAN_POINT('Ctrl Pts',(98.0711656112444,-139.704730507617,-83.6786258523484));
#24011=CARTESIAN_POINT('Ctrl Pts',(98.0285985107537,-139.719438415389,-83.6511101865903));
#24012=CARTESIAN_POINT('Ctrl Pts',(97.9864063827793,-139.734002420143,-83.6226254451987));
#24013=CARTESIAN_POINT('Ctrl Pts',(97.9447745948348,-139.748359981237,-83.5930927466016));
#24014=CARTESIAN_POINT('Ctrl Pts',(97.9055854441768,-139.761875149636,-83.5652928025733));
#24015=CARTESIAN_POINT('Ctrl Pts',(97.8668926229667,-139.775207447803,-83.5365641602674));
#24016=CARTESIAN_POINT('Ctrl Pts',(97.828893412403,-139.788290019043,-83.5068350472078));
#24017=CARTESIAN_POINT('Ctrl Pts',(97.804144005828,-139.796810876973,-83.4874720684692));
#24018=CARTESIAN_POINT('Ctrl Pts',(97.7796896932354,-139.805225503118,-83.4676845636184));
#24019=CARTESIAN_POINT('Ctrl Pts',(97.7555963200441,-139.813511537342,-83.4474515115311));
#24020=CARTESIAN_POINT('Ctrl Pts',(97.728363634325,-139.822877223255,-83.424582138104));
#24021=CARTESIAN_POINT('Ctrl Pts',(97.7016349752933,-139.832064017308,-83.4011923028985));
#24022=CARTESIAN_POINT('Ctrl Pts',(97.6754851218662,-139.841046916235,-83.3772268830841));
#24023=CARTESIAN_POINT('Ctrl Pts',(97.6463215006398,-139.851065093299,-83.3504994512098));
#24024=CARTESIAN_POINT('Ctrl Pts',(97.6179056267942,-139.860816746996,-83.3230936650656));
#24025=CARTESIAN_POINT('Ctrl Pts',(97.5902935806194,-139.87028550355,-83.2948558990642));
#24026=CARTESIAN_POINT('Ctrl Pts',(97.5639466259767,-139.879320433372,-83.2679118929831));
#24027=CARTESIAN_POINT('Ctrl Pts',(97.5383314014496,-139.88809782761,-83.2402104364255));
#24028=CARTESIAN_POINT('Ctrl Pts',(97.5135388526037,-139.896588714057,-83.2116040346635));
#24029=CARTESIAN_POINT('Ctrl Pts',(97.4980774724969,-139.901883886554,-83.1937642210211));
#24030=CARTESIAN_POINT('Ctrl Pts',(97.4829368794924,-139.907067340337,-83.17557218315));
#24031=CARTESIAN_POINT('Ctrl Pts',(97.4681484941753,-139.91212881033,-83.1569890466364));
#24032=CARTESIAN_POINT('Ctrl Pts',(97.4476130510072,-139.919157267269,-83.1311841372042));
#24033=CARTESIAN_POINT('Ctrl Pts',(97.4277452420287,-139.925954449789,-83.1045520895884));
#24034=CARTESIAN_POINT('Ctrl Pts',(97.4087167048375,-139.932462814289,-83.0770775195449));
#24035=CARTESIAN_POINT('Ctrl Pts',(97.3896881676464,-139.938971178789,-83.0496029495014));
#24036=CARTESIAN_POINT('Ctrl Pts',(97.3714983087636,-139.945190921619,-83.0212855162084));
#24037=CARTESIAN_POINT('Ctrl Pts',(97.3543677310461,-139.951047779757,-82.9921212813803));
#24038=CARTESIAN_POINT('Ctrl Pts',(97.3386981110691,-139.956405143811,-82.9654442781753));
#24039=CARTESIAN_POINT('Ctrl Pts',(97.3240367075897,-139.961419891151,-82.9382531572));
#24040=CARTESIAN_POINT('Ctrl Pts',(97.3105164866214,-139.966044132201,-82.910533567852));
#24041=CARTESIAN_POINT('Ctrl Pts',(97.2987364265489,-139.970073196333,-82.8863817120154));
#24042=CARTESIAN_POINT('Ctrl Pts',(97.2878230738592,-139.973805693467,-82.8618285577111));
#24043=CARTESIAN_POINT('Ctrl Pts',(97.277894901901,-139.977199920877,-82.8368687469214));
#24044=CARTESIAN_POINT('Ctrl Pts',(97.2675449135807,-139.980738358185,-82.8108484733772));
#24045=CARTESIAN_POINT('Ctrl Pts',(97.2582088704294,-139.983928680802,-82.7843403311583));
#24046=CARTESIAN_POINT('Ctrl Pts',(97.2499984542927,-139.986731261435,-82.757268617013));
#24047=CARTESIAN_POINT('Ctrl Pts',(97.2412356636815,-139.989722392072,-82.7283755915447));
#24048=CARTESIAN_POINT('Ctrl Pts',(97.2338238173965,-139.992251733102,-82.6990112555058));
#24049=CARTESIAN_POINT('Ctrl Pts',(97.2279126563665,-139.99426861304,-82.6692964230559));
#24050=CARTESIAN_POINT('Ctrl Pts',(97.2221710252593,-139.996227649603,-82.6404338010639));
#24051=CARTESIAN_POINT('Ctrl Pts',(97.2178453353219,-139.997703166035,-82.6112405024812));
#24052=CARTESIAN_POINT('Ctrl Pts',(97.2150271728466,-139.998664330779,-82.5818324954324));
#24053=CARTESIAN_POINT('Ctrl Pts',(97.21242764044,-139.999550929378,-82.5547059305124));
#24054=CARTESIAN_POINT('Ctrl Pts',(97.2111104751974,-140.,-82.5273967255209));
#24055=CARTESIAN_POINT('Ctrl Pts',(97.2111104761178,-140.,-82.5));
#24056=CARTESIAN_POINT('Origin',(0.,0.,-87.5));
#24057=CARTESIAN_POINT('Origin',(104.163333279998,-137.5,-87.5));
#24058=CARTESIAN_POINT('Origin',(116.189500386223,-127.5,-87.5));
#24059=CARTESIAN_POINT('Ctrl Pts',(119.689439203101,-120.724637681159,-82.5));
#24060=CARTESIAN_POINT('Ctrl Pts',(115.377099114166,-125.,-82.5));
#24061=CARTESIAN_POINT('Ctrl Pts',(121.449578014911,-125.,-82.5));
#24062=CARTESIAN_POINT('Ctrl Pts',(119.689439200917,-120.724637683324,-82.7056798133782));
#24063=CARTESIAN_POINT('Ctrl Pts',(115.377099118341,-124.999999995701,-82.3507082521197));
#24064=CARTESIAN_POINT('Ctrl Pts',(121.449578012695,-125.,-82.6028399066646));
#24065=CARTESIAN_POINT('Ctrl Pts',(119.676882557983,-120.737090180421,-82.9079954286207));
#24066=CARTESIAN_POINT('Ctrl Pts',(115.401361881511,-124.975048941511,-82.2053610116202));
#24067=CARTESIAN_POINT('Ctrl Pts',(121.436836713265,-125.006317811859,-82.7039977143433));
#24068=CARTESIAN_POINT('Ctrl Pts',(119.628410587298,-120.785117230515,-83.3063417968652));
#24069=CARTESIAN_POINT('Ctrl Pts',(115.489012547634,-124.884856124345,-81.9514922386294));
#24070=CARTESIAN_POINT('Ctrl Pts',(121.387651919446,-125.030684477513,-82.9031708983997));
#24071=CARTESIAN_POINT('Ctrl Pts',(119.592485604525,-120.820701126369,-83.5023756354685));
#24072=CARTESIAN_POINT('Ctrl Pts',(115.551419916513,-124.820623886438,-81.844093442978));
#24073=CARTESIAN_POINT('Ctrl Pts',(121.351198628156,-125.048738071447,-83.0011878177447));
#24074=CARTESIAN_POINT('Ctrl Pts',(119.497801818693,-120.91434900059,-83.8883271564993));
#24075=CARTESIAN_POINT('Ctrl Pts',(115.697825563992,-124.669744960185,-81.6876871655071));
#24076=CARTESIAN_POINT('Ctrl Pts',(121.255122433638,-125.096250595907,-83.1941635782393));
#24077=CARTESIAN_POINT('Ctrl Pts',(119.439376348876,-120.972080469663,-84.0761788301475));
#24078=CARTESIAN_POINT('Ctrl Pts',(115.779889571829,-124.585091209873,-81.639444465222));
#24079=CARTESIAN_POINT('Ctrl Pts',(121.195837765812,-125.125540825988,-83.2880894152805));
#24080=CARTESIAN_POINT('Ctrl Pts',(119.305221428487,-121.104388919918,-84.4342801401529));
#24081=CARTESIAN_POINT('Ctrl Pts',(115.940258775456,-124.419250986645,-81.6056236890861));
#24082=CARTESIAN_POINT('Ctrl Pts',(121.059709978865,-125.192667908432,-83.4671400698696));
#24083=CARTESIAN_POINT('Ctrl Pts',(119.229146767872,-121.179307379907,-84.6059387232763));
#24084=CARTESIAN_POINT('Ctrl Pts',(116.018662098376,-124.337976550129,-81.6177805257506));
#24085=CARTESIAN_POINT('Ctrl Pts',(120.982516573327,-125.230678008636,-83.5529693617978));
#24086=CARTESIAN_POINT('Ctrl Pts',(119.060491893051,-121.345017393603,-84.9357796688685));
#24087=CARTESIAN_POINT('Ctrl Pts',(116.159254888288,-124.191486350903,-81.6927658265867));
#24088=CARTESIAN_POINT('Ctrl Pts',(120.811381479668,-125.314751472042,-83.7178898342746));
#24089=CARTESIAN_POINT('Ctrl Pts',(118.96776206845,-121.435951457507,-85.093861858456));
#24090=CARTESIAN_POINT('Ctrl Pts',(116.221496701314,-124.12623198531,-81.7541916577615));
#24091=CARTESIAN_POINT('Ctrl Pts',(120.717287981259,-125.36088713601,-83.7969309295804));
#24092=CARTESIAN_POINT('Ctrl Pts',(118.772148188168,-121.627281202587,-85.3899146057789));
#24093=CARTESIAN_POINT('Ctrl Pts',(116.320002770212,-124.021697634043,-81.9095222659674));
#24094=CARTESIAN_POINT('Ctrl Pts',(120.518797426192,-125.45795884595,-83.9449573025371));
#24095=CARTESIAN_POINT('Ctrl Pts',(118.66868983755,-121.728242289117,-85.5290754975167));
#24096=CARTESIAN_POINT('Ctrl Pts',(116.35752640374,-123.981145420879,-82.0023320413466));
#24097=CARTESIAN_POINT('Ctrl Pts',(120.413817629313,-125.50918174931,-84.0145377490307));
#24098=CARTESIAN_POINT('Ctrl Pts',(118.45169839953,-121.939403249423,-85.7917547211079));
#24099=CARTESIAN_POINT('Ctrl Pts',(116.406873166747,-123.925571355125,-82.2074570860312));
#24100=CARTESIAN_POINT('Ctrl Pts',(120.193635140666,-125.616314884214,-84.1458773602816));
#24101=CARTESIAN_POINT('Ctrl Pts',(118.338158476483,-122.049610026221,-85.9152619328964));
#24102=CARTESIAN_POINT('Ctrl Pts',(116.419520677459,-123.909734352817,-82.3190059601612));
#24103=CARTESIAN_POINT('Ctrl Pts',(120.078425512936,-125.672228616066,-84.2076309666417));
#24104=CARTESIAN_POINT('Ctrl Pts',(118.101739972007,-122.278395780866,-86.1479296435188));
#24105=CARTESIAN_POINT('Ctrl Pts',(116.420156575106,-123.902371131663,-82.5520650696801));
#24106=CARTESIAN_POINT('Ctrl Pts',(119.838530265679,-125.788303741941,-84.323964821566));
#24107=CARTESIAN_POINT('Ctrl Pts',(117.978621353548,-122.397201959151,-86.2571677342239));
#24108=CARTESIAN_POINT('Ctrl Pts',(116.408784821067,-123.910208556756,-82.6734238697007));
#24109=CARTESIAN_POINT('Ctrl Pts',(119.713601079353,-125.848580405477,-84.3785838674499));
#24110=CARTESIAN_POINT('Ctrl Pts',(117.603241895162,-122.758291253176,-86.5592543593046));
#24111=CARTESIAN_POINT('Ctrl Pts',(116.343210235511,-123.964762276173,-83.0296153459409));
#24112=CARTESIAN_POINT('Ctrl Pts',(119.332701334762,-126.031780121634,-84.5296271789764));
#24113=CARTESIAN_POINT('Ctrl Pts',(117.342767505456,-123.007368772318,-86.7291564746629));
#24114=CARTESIAN_POINT('Ctrl Pts',(116.259553389397,-124.040181684855,-83.2697315003776));
#24115=CARTESIAN_POINT('Ctrl Pts',(119.068396439392,-126.158150332831,-84.6145782376957));
#24116=CARTESIAN_POINT('Ctrl Pts',(116.804336290701,-123.518763278367,-87.016825817368));
#24117=CARTESIAN_POINT('Ctrl Pts',(116.02736829311,-124.252946369571,-83.719666170302));
#24118=CARTESIAN_POINT('Ctrl Pts',(118.522047118472,-126.417607839943,-84.7584129083197));
#24119=CARTESIAN_POINT('Ctrl Pts',(116.525023660541,-123.782353191699,-87.1348755768559));
#24120=CARTESIAN_POINT('Ctrl Pts',(115.881406957192,-124.387808755614,-83.9325453429328));
#24121=CARTESIAN_POINT('Ctrl Pts',(118.238626949673,-126.551340957402,-84.8174377888648));
#24122=CARTESIAN_POINT('Ctrl Pts',(115.671272356593,-124.582362934983,-87.4141780079963));
#24123=CARTESIAN_POINT('Ctrl Pts',(115.387279747815,-124.844116246409,-84.4905439734664));
#24124=CARTESIAN_POINT('Ctrl Pts',(117.372320479471,-126.95722825408,-84.9570890031244));
#24125=CARTESIAN_POINT('Ctrl Pts',(115.092722580527,-125.117129923752,-87.4999999999441));
#24126=CARTESIAN_POINT('Ctrl Pts',(114.975356365159,-125.224084605229,-84.7914664637583));
#24127=CARTESIAN_POINT('Ctrl Pts',(116.785263550907,-127.228543433487,-85.));
#24128=CARTESIAN_POINT('Ctrl Pts',(114.505594583524,-125.652173913043,-87.5));
#24129=CARTESIAN_POINT('Ctrl Pts',(114.505594583524,-125.652173913043,-85.));
#24130=CARTESIAN_POINT('Ctrl Pts',(116.189500386222,-127.5,-85.));
#24131=CARTESIAN_POINT('Origin',(177.5,-127.5,73.9644660940673));
#24132=CARTESIAN_POINT('Origin',(177.5,-127.5,73.9644660940673));
#24133=CARTESIAN_POINT('Origin',(168.964466094067,-137.5,82.5));
#24134=CARTESIAN_POINT('Origin',(168.964466094067,-137.5,82.5));
#24135=CARTESIAN_POINT('Origin',(168.964466094067,-137.5,82.5));
#24136=CARTESIAN_POINT('Ctrl Pts',(102.653719754201,-135.507246376812,-87.5));
#24137=CARTESIAN_POINT('Ctrl Pts',(102.653719754201,-135.507246376812,-85.));
#24138=CARTESIAN_POINT('Ctrl Pts',(104.163333279998,-137.5,-85.));
#24139=CARTESIAN_POINT('Ctrl Pts',(101.942824967883,-136.045785799024,-87.4999999986499));
#24140=CARTESIAN_POINT('Ctrl Pts',(102.098115024429,-135.928145581712,-85.2088536164867));
#24141=CARTESIAN_POINT('Ctrl Pts',(103.441984205064,-137.773229542126,-85.));
#24142=CARTESIAN_POINT('Ctrl Pts',(101.239352594638,-136.569897864386,-87.412786288228));
#24143=CARTESIAN_POINT('Ctrl Pts',(101.486609565828,-136.386099347641,-85.331905314613));
#24144=CARTESIAN_POINT('Ctrl Pts',(102.728166603362,-138.039139357556,-84.9563931437868));
#24145=CARTESIAN_POINT('Ctrl Pts',(100.196407749732,-137.334867215748,-87.1513844296707));
#24146=CARTESIAN_POINT('Ctrl Pts',(100.54257036391,-137.08212804413,-85.3647787687136));
#24147=CARTESIAN_POINT('Ctrl Pts',(101.669884334297,-138.427248808045,-84.825692214999));
#24148=CARTESIAN_POINT('Ctrl Pts',(99.8508244887539,-137.58630689324,-87.0421034532917));
#24149=CARTESIAN_POINT('Ctrl Pts',(100.230398916982,-137.310719986095,-85.3526237075885));
#24150=CARTESIAN_POINT('Ctrl Pts',(101.319218966522,-138.554817467693,-84.7710517262891));
#24151=CARTESIAN_POINT('Ctrl Pts',(99.1647702284533,-138.081596677989,-86.7728948774191));
#24152=CARTESIAN_POINT('Ctrl Pts',(99.6048287382421,-137.765412086316,-85.2762415031115));
#24153=CARTESIAN_POINT('Ctrl Pts',(100.623075672997,-138.806104197121,-84.6364474390664));
#24154=CARTESIAN_POINT('Ctrl Pts',(98.8231223087188,-138.326258685221,-86.6120988871654));
#24155=CARTESIAN_POINT('Ctrl Pts',(99.2895441365193,-137.992946799803,-85.2128933853019));
#24156=CARTESIAN_POINT('Ctrl Pts',(100.276403519106,-138.930234185559,-84.5560494432021));
#24157=CARTESIAN_POINT('Ctrl Pts',(98.1642932033775,-138.794578008566,-86.236965419431));
#24158=CARTESIAN_POINT('Ctrl Pts',(98.6779850295722,-138.431144249613,-85.0309421888964));
#24159=CARTESIAN_POINT('Ctrl Pts',(99.6078857505209,-139.167837372319,-84.3684827100962));
#24160=CARTESIAN_POINT('Ctrl Pts',(97.8450871550092,-139.019702589725,-86.0223563343333));
#24161=CARTESIAN_POINT('Ctrl Pts',(98.3787305056279,-138.644046161722,-84.9137267915435));
#24162=CARTESIAN_POINT('Ctrl Pts',(99.283985495488,-139.28205498953,-84.2611781664592));
#24163=CARTESIAN_POINT('Ctrl Pts',(97.2348460956408,-139.447206832062,-85.5210364529044));
#24164=CARTESIAN_POINT('Ctrl Pts',(97.8048933229574,-139.049632684085,-84.6126732163398));
#24165=CARTESIAN_POINT('Ctrl Pts',(98.6647703029657,-139.498950525936,-84.0105182271597));
#24166=CARTESIAN_POINT('Ctrl Pts',(96.9485250987458,-139.646264128654,-85.2381599055602));
#24167=CARTESIAN_POINT('Ctrl Pts',(97.5330426499524,-139.240425205481,-84.4318673801205));
#24168=CARTESIAN_POINT('Ctrl Pts',(98.3742387030706,-139.599942828535,-83.869079952008));
#24169=CARTESIAN_POINT('Ctrl Pts',(96.5670588723941,-139.910067692477,-84.7527693623909));
#24170=CARTESIAN_POINT('Ctrl Pts',(97.1694267365962,-139.49429609941,-84.1046276840804));
#24171=CARTESIAN_POINT('Ctrl Pts',(97.9871626793753,-139.7337843447,-83.6263846815815));
#24172=CARTESIAN_POINT('Ctrl Pts',(96.446921948779,-139.992887137954,-84.5790592166605));
#24173=CARTESIAN_POINT('Ctrl Pts',(97.0550355767484,-139.573924747954,-83.985796851679));
#24174=CARTESIAN_POINT('Ctrl Pts',(97.8652590362145,-139.775803032622,-83.5395296080959));
#24175=CARTESIAN_POINT('Ctrl Pts',(96.230792082191,-140.141542227306,-84.2107293038302));
#24176=CARTESIAN_POINT('Ctrl Pts',(96.8492338219199,-139.716869275045,-83.7297846724926));
#24177=CARTESIAN_POINT('Ctrl Pts',(97.6459507893286,-139.851223630635,-83.3553646521495));
#24178=CARTESIAN_POINT('Ctrl Pts',(96.1354852319174,-140.20691083986,-84.0176816842604));
#24179=CARTESIAN_POINT('Ctrl Pts',(96.7581590378938,-139.779958879001,-83.5936364082725));
#24180=CARTESIAN_POINT('Ctrl Pts',(97.5492423676424,-139.884388586841,-83.2588408418563));
#24181=CARTESIAN_POINT('Ctrl Pts',(95.9757708369295,-140.316288364145,-83.6101822300658));
#24182=CARTESIAN_POINT('Ctrl Pts',(96.6056940387067,-139.885419084152,-83.3034331025056));
#24183=CARTESIAN_POINT('Ctrl Pts',(97.3871792316287,-139.939881597544,-83.0550911153068));
#24184=CARTESIAN_POINT('Ctrl Pts',(95.9112233305706,-140.360393155342,-83.3934903679299));
#24185=CARTESIAN_POINT('Ctrl Pts',(96.5438567051695,-139.928100230385,-83.1474982708776));
#24186=CARTESIAN_POINT('Ctrl Pts',(97.3216824971681,-139.962258291636,-82.9467451839126));
#24187=CARTESIAN_POINT('Ctrl Pts',(95.8249655550993,-140.419296052404,-82.9539654903595));
#24188=CARTESIAN_POINT('Ctrl Pts',(96.4613838167463,-139.984990149168,-82.8298756349127));
#24189=CARTESIAN_POINT('Ctrl Pts',(97.2341562250557,-139.99214285053,-82.7269827452321));
#24190=CARTESIAN_POINT('Ctrl Pts',(95.802253798755,-140.434782611285,-82.7294636530625));
#24191=CARTESIAN_POINT('Ctrl Pts',(96.4395937226627,-140.0000000025,-82.6666388430675));
#24192=CARTESIAN_POINT('Ctrl Pts',(97.2111104722631,-140.,-82.6147318264911));
#24193=CARTESIAN_POINT('Ctrl Pts',(95.802253802551,-140.434782608696,-82.5));
#24194=CARTESIAN_POINT('Ctrl Pts',(96.4395937263074,-140.,-82.5));
#24195=CARTESIAN_POINT('Ctrl Pts',(97.2111104761179,-140.,-82.5));
#24196=CARTESIAN_POINT('Origin',(97.2111104761179,-142.5,-82.5));
#24197=CARTESIAN_POINT('Origin',(140.840826156048,-127.5,110.623639938019));
#24198=CARTESIAN_POINT('Origin',(168.964466094067,-127.5,82.5));
#24199=CARTESIAN_POINT('Origin',(168.964466094067,0.,82.5));
#24200=CARTESIAN_POINT('Origin',(168.964466094067,-127.5,82.5));
#24201=CARTESIAN_POINT('Origin',(180.,-137.5,82.5));
#24202=CARTESIAN_POINT('Ctrl Pts',(97.2111104761179,-140.,82.5));
#24203=CARTESIAN_POINT('Ctrl Pts',(97.2111104761179,-140.,82.6755496768536));
#24204=CARTESIAN_POINT('Ctrl Pts',(97.2669993053863,-139.980948398877,82.8433669193193));
#24205=CARTESIAN_POINT('Ctrl Pts',(97.4416750152787,-139.921239210978,83.1407858319269));
#24206=CARTESIAN_POINT('Ctrl Pts',(97.5528693408584,-139.883166869044,83.2647663586162));
#24207=CARTESIAN_POINT('Ctrl Pts',(97.7975572341499,-139.799120034918,83.4891405228876));
#24208=CARTESIAN_POINT('Ctrl Pts',(97.9325262666959,-139.752638285023,83.5889920461804));
#24209=CARTESIAN_POINT('Ctrl Pts',(98.2091898573102,-139.657040028271,83.7678569462812));
#24210=CARTESIAN_POINT('Ctrl Pts',(98.3521285688953,-139.607498613007,83.8477491623104));
#24211=CARTESIAN_POINT('Ctrl Pts',(98.7901601853575,-139.455163852716,84.0681986935237));
#24212=CARTESIAN_POINT('Ctrl Pts',(99.0953089605357,-139.348355708036,84.1900813067333));
#24213=CARTESIAN_POINT('Ctrl Pts',(99.7103269532128,-139.131535702876,84.4002328533732));
#24214=CARTESIAN_POINT('Ctrl Pts',(100.021642419245,-139.021028910904,84.4887015138217));
#24215=CARTESIAN_POINT('Ctrl Pts',(100.963515042103,-138.68428076857,84.7184070178217));
#24216=CARTESIAN_POINT('Ctrl Pts',(101.60311676071,-138.452377890846,84.8244784333066));
#24217=CARTESIAN_POINT('Ctrl Pts',(102.880937057798,-137.982203598024,84.9652998446299));
#24218=CARTESIAN_POINT('Ctrl Pts',(103.521414707761,-137.743143193377,85.));
#24219=CARTESIAN_POINT('Ctrl Pts',(104.163333279998,-137.5,85.));
#24220=CARTESIAN_POINT('Origin',(97.2111104761179,-142.5,115.));
#24221=CARTESIAN_POINT('Origin',(97.2111104761179,-142.5,82.5));
#24222=CARTESIAN_POINT('Origin',(121.449578014911,-122.5,-49.5));
#24223=CARTESIAN_POINT('Origin',(121.449578014911,-122.5,-49.5));
#24224=CARTESIAN_POINT('Origin',(121.449578014911,-122.5,-49.5));
#24225=CARTESIAN_POINT('Origin',(168.964466094067,-127.5,82.5));
#24226=CARTESIAN_POINT('Origin',(168.964466094067,-127.5,82.5));
#24227=CARTESIAN_POINT('Ctrl Pts',(95.8063843937655,-140.431966711357,82.3302220946682));
#24228=CARTESIAN_POINT('Ctrl Pts',(96.4436693342528,-139.997193891514,82.3767164474287));
#24229=CARTESIAN_POINT('Ctrl Pts',(97.2155465823485,-139.998571769581,82.4151232270192));
#24230=CARTESIAN_POINT('Ctrl Pts',(95.7923535903208,-140.44153068871,82.6189757789366));
#24231=CARTESIAN_POINT('Ctrl Pts',(96.4301984592196,-140.006470158917,82.5862803340826));
#24232=CARTESIAN_POINT('Ctrl Pts',(97.2013093103815,-140.003422681504,82.5594793863882));
#24233=CARTESIAN_POINT('Ctrl Pts',(95.8143433314503,-140.426549686738,82.8999538047621));
#24234=CARTESIAN_POINT('Ctrl Pts',(96.451370555694,-139.991898168234,82.7909496905922));
#24235=CARTESIAN_POINT('Ctrl Pts',(97.2236226187951,-139.995824235922,82.69994805132));
#24236=CARTESIAN_POINT('Ctrl Pts',(95.9113524568369,-140.360304954438,83.3940569629634));
#24237=CARTESIAN_POINT('Ctrl Pts',(96.5440906351144,-139.927939556875,83.1478648493756));
#24238=CARTESIAN_POINT('Ctrl Pts',(97.3220593832045,-139.962224365005,82.9469649889257));
#24239=CARTESIAN_POINT('Ctrl Pts',(95.9760732771133,-140.316081550096,83.6111084029453));
#24240=CARTESIAN_POINT('Ctrl Pts',(96.6060933643896,-139.88514399948,83.3040436736954));
#24241=CARTESIAN_POINT('Ctrl Pts',(97.3877326179702,-139.939793891199,83.0554758102092));
#24242=CARTESIAN_POINT('Ctrl Pts',(96.1359171968624,-140.206614708383,84.0186285797908));
#24243=CARTESIAN_POINT('Ctrl Pts',(96.7586808353661,-139.779598324237,83.5942322269066));
#24244=CARTESIAN_POINT('Ctrl Pts',(97.549928900367,-139.884271165605,83.2592091881112));
#24245=CARTESIAN_POINT('Ctrl Pts',(96.2312574439685,-140.141222656174,84.2116073129497));
#24246=CARTESIAN_POINT('Ctrl Pts',(96.8497861981093,-139.716486932324,83.7303149679427));
#24247=CARTESIAN_POINT('Ctrl Pts',(97.6466721866358,-139.851103576304,83.3556865024526));
#24248=CARTESIAN_POINT('Ctrl Pts',(96.4473504048935,-139.992591935039,84.5797041056106));
#24249=CARTESIAN_POINT('Ctrl Pts',(97.0555509298913,-139.573566933705,83.9861341719472));
#24250=CARTESIAN_POINT('Ctrl Pts',(97.8659453704935,-139.775715999607,83.5397134594335));
#24251=CARTESIAN_POINT('Ctrl Pts',(96.5679243919307,-139.909470610042,84.7539893762804));
#24252=CARTESIAN_POINT('Ctrl Pts',(97.170358683852,-139.493647616232,84.1053449301989));
#24253=CARTESIAN_POINT('Ctrl Pts',(97.9882938037511,-139.733555567922,83.6268467456624));
#24254=CARTESIAN_POINT('Ctrl Pts',(96.9500803569823,-139.645185630464,85.2398999355275));
#24255=CARTESIAN_POINT('Ctrl Pts',(97.5346293969998,-139.239315047688,84.4328697043282));
#24256=CARTESIAN_POINT('Ctrl Pts',(98.3760735528311,-139.599505523373,83.8697781593213));
#24257=CARTESIAN_POINT('Ctrl Pts',(97.2354525040957,-139.44678671983,85.5216876072768));
#24258=CARTESIAN_POINT('Ctrl Pts',(97.8055901602141,-139.049145300856,84.6129417193528));
#24259=CARTESIAN_POINT('Ctrl Pts',(98.6656453772965,-139.498873185454,84.0106618938605));
#24260=CARTESIAN_POINT('Ctrl Pts',(97.84736130348,-139.018104706215,86.0240708677892));
#24261=CARTESIAN_POINT('Ctrl Pts',(98.3809815624723,-138.642451119717,84.9145219274169));
#24262=CARTESIAN_POINT('Ctrl Pts',(99.2865604725242,-139.281432946434,84.2618427002277));
#24263=CARTESIAN_POINT('Ctrl Pts',(98.166043362077,-138.793333891558,86.2379611602865));
#24264=CARTESIAN_POINT('Ctrl Pts',(98.6796642081939,-138.429941914644,85.0311843476465));
#24265=CARTESIAN_POINT('Ctrl Pts',(99.6099329912234,-139.167421255509,84.3687873468945));
#24266=CARTESIAN_POINT('Ctrl Pts',(98.8213488187872,-138.327519386904,86.6110898616138));
#24267=CARTESIAN_POINT('Ctrl Pts',(99.2879449246068,-137.99409288667,85.2121201908167));
#24268=CARTESIAN_POINT('Ctrl Pts',(100.27488438625,-138.931140045816,84.5553582822027));
#24269=CARTESIAN_POINT('Ctrl Pts',(99.1580967027271,-138.086393592505,86.7699896797119));
#24270=CARTESIAN_POINT('Ctrl Pts',(99.598826751245,-137.769758011627,85.2749349361932));
#24271=CARTESIAN_POINT('Ctrl Pts',(100.616589177685,-138.808829045632,84.6348154491461));
#24272=CARTESIAN_POINT('Ctrl Pts',(99.8465457819706,-137.589416498873,87.0407064600204));
#24273=CARTESIAN_POINT('Ctrl Pts',(100.226641408901,-137.313468734571,85.3520865086701));
#24274=CARTESIAN_POINT('Ctrl Pts',(101.3151733035,-138.556733152654,84.7701949757436));
#24275=CARTESIAN_POINT('Ctrl Pts',(100.196958385717,-137.33447257932,87.1516264431956));
#24276=CARTESIAN_POINT('Ctrl Pts',(100.543205603977,-137.081667395925,85.3644982653917));
#24277=CARTESIAN_POINT('Ctrl Pts',(101.670744758202,-138.427408643403,84.8256690051307));
#24278=CARTESIAN_POINT('Ctrl Pts',(101.288218386673,-136.534036534848,87.4248120559258));
#24279=CARTESIAN_POINT('Ctrl Pts',(101.533114418443,-136.351795325559,85.3295920701954));
#24280=CARTESIAN_POINT('Ctrl Pts',(102.778066848937,-138.021368555809,84.9623127946856));
#24281=CARTESIAN_POINT('Ctrl Pts',(102.034252820327,-135.97755865104,87.5102062320107));
#24282=CARTESIAN_POINT('Ctrl Pts',(102.179857181174,-135.866853574868,85.1905835680137));
#24283=CARTESIAN_POINT('Ctrl Pts',(103.535087152153,-137.739070348775,85.0050578474458));
#24284=CARTESIAN_POINT('Ctrl Pts',(102.78362116352,-135.408741267552,87.4990307673126));
#24285=CARTESIAN_POINT('Ctrl Pts',(102.759250409394,-135.427238236656,84.9584361067191));
#24286=CARTESIAN_POINT('Ctrl Pts',(104.295502567804,-137.450494181459,84.9995248789653));
#24287=CARTESIAN_POINT('Origin',(104.163333279998,-137.5,87.5));
#24288=CARTESIAN_POINT('Origin',(0.,0.,-49.5));
#24289=CARTESIAN_POINT('Origin',(147.5,-89.4427190999916,-49.5));
#24290=CARTESIAN_POINT('Origin',(147.5,0.,-44.5));
#24291=CARTESIAN_POINT('Origin',(147.5,-122.5,-44.5));
#24292=CARTESIAN_POINT('Ctrl Pts',(150.,-80.6225774829854,-44.5));
#24293=CARTESIAN_POINT('Ctrl Pts',(150.,-80.6225774829854,-44.5312343888304));
#24294=CARTESIAN_POINT('Ctrl Pts',(149.999418286665,-80.6247797743348,-44.5621210164789));
#24295=CARTESIAN_POINT('Ctrl Pts',(149.998293554945,-80.6290354954265,-44.5925723355625));
#24296=CARTESIAN_POINT('Ctrl Pts',(149.997125538082,-80.6334549973542,-44.6241955694378));
#24297=CARTESIAN_POINT('Ctrl Pts',(149.995371936956,-80.6400888791781,-44.655349356458));
#24298=CARTESIAN_POINT('Ctrl Pts',(149.993090530187,-80.6487160556979,-44.6859412124329));
#24299=CARTESIAN_POINT('Ctrl Pts',(149.992231155702,-80.6519657941861,-44.6974647429366));
#24300=CARTESIAN_POINT('Ctrl Pts',(149.991297028852,-80.6554978429527,-44.7089085934095));
#24301=CARTESIAN_POINT('Ctrl Pts',(149.990291719683,-80.6592985775913,-44.7202680068894));
#24302=CARTESIAN_POINT('Ctrl Pts',(149.987499102739,-80.6698565196466,-44.7518229668389));
#24303=CARTESIAN_POINT('Ctrl Pts',(149.984157100677,-80.6824881297728,-44.7827141728588));
#24304=CARTESIAN_POINT('Ctrl Pts',(149.980355786964,-80.6968505802923,-44.8128256266941));
#24305=CARTESIAN_POINT('Ctrl Pts',(149.977558137322,-80.7074209008703,-44.8349867279405));
#24306=CARTESIAN_POINT('Ctrl Pts',(149.974509955706,-80.7189351701335,-44.8567449506927));
#24307=CARTESIAN_POINT('Ctrl Pts',(149.971243495187,-80.7312708109915,-44.8780946805967));
#24308=CARTESIAN_POINT('Ctrl Pts',(149.965898079908,-80.7514575307578,-44.9130325504344));
#24309=CARTESIAN_POINT('Ctrl Pts',(149.960009186179,-80.773686648641,-44.9465704967713));
#24310=CARTESIAN_POINT('Ctrl Pts',(149.953740444404,-80.797335293561,-44.9787015735967));
#24311=CARTESIAN_POINT('Ctrl Pts',(149.948225014278,-80.8181420923231,-45.0069714745479));
#24312=CARTESIAN_POINT('Ctrl Pts',(149.9424154207,-80.8400482470994,-45.0341525202745));
#24313=CARTESIAN_POINT('Ctrl Pts',(149.936415096464,-80.8626613647233,-45.0602466352771));
#24314=CARTESIAN_POINT('Ctrl Pts',(149.930229230798,-80.8859737229195,-45.0871476299065));
#24315=CARTESIAN_POINT('Ctrl Pts',(149.923781601043,-80.9102578633712,-45.1131530185116));
#24316=CARTESIAN_POINT('Ctrl Pts',(149.917129634266,-80.9352949903539,-45.1383421170535));
#24317=CARTESIAN_POINT('Ctrl Pts',(149.910169623638,-80.9614915538295,-45.1646976896917));
#24318=CARTESIAN_POINT('Ctrl Pts',(149.902985851619,-80.9885126935503,-45.1901596664586));
#24319=CARTESIAN_POINT('Ctrl Pts',(149.895629953764,-81.0161619977713,-45.2148125956205));
#24320=CARTESIAN_POINT('Ctrl Pts',(149.894768894784,-81.0193985410376,-45.2176983923565));
#24321=CARTESIAN_POINT('Ctrl Pts',(149.893905462669,-81.0226437475977,-45.2205730959881));
#24322=CARTESIAN_POINT('Ctrl Pts',(149.893039728921,-81.0258973457795,-45.2234368363464));
#24323=CARTESIAN_POINT('Ctrl Pts',(149.885294621979,-81.055004985282,-45.2490566939069));
#24324=CARTESIAN_POINT('Ctrl Pts',(149.877335285324,-81.0848961910411,-45.2738874208924));
#24325=CARTESIAN_POINT('Ctrl Pts',(149.869211724912,-81.1153826082176,-45.2979942587922));
#24326=CARTESIAN_POINT('Ctrl Pts',(149.860756318493,-81.1471143901477,-45.3230858567598));
#24327=CARTESIAN_POINT('Ctrl Pts',(149.852122887,-81.179491428094,-45.3473933229362));
#24328=CARTESIAN_POINT('Ctrl Pts',(149.843353240441,-81.212356779593,-45.3709861423032));
#24329=CARTESIAN_POINT('Ctrl Pts',(149.834033859779,-81.2472823286657,-45.3960579012523));
#24330=CARTESIAN_POINT('Ctrl Pts',(149.824560562659,-81.282759673792,-45.420322766943));
#24331=CARTESIAN_POINT('Ctrl Pts',(149.814968902639,-81.318656015993,-45.4438574826091));
#24332=CARTESIAN_POINT('Ctrl Pts',(149.814245534136,-81.3213631890219,-45.4456323862228));
#24333=CARTESIAN_POINT('Ctrl Pts',(149.813521486337,-81.3240727682655,-45.4474031333746));
#24334=CARTESIAN_POINT('Ctrl Pts',(149.81279677161,-81.3267847076918,-45.4491697551619));
#24335=CARTESIAN_POINT('Ctrl Pts',(149.802161746897,-81.3665818053887,-45.4750945303171));
#24336=CARTESIAN_POINT('Ctrl Pts',(149.791378236576,-81.4068954418303,-45.5001449499175));
#24337=CARTESIAN_POINT('Ctrl Pts',(149.780505488345,-81.4474999785173,-45.5243508763432));
#24338=CARTESIAN_POINT('Ctrl Pts',(149.766212096436,-81.5008789903218,-45.5561721588362));
#24339=CARTESIAN_POINT('Ctrl Pts',(149.75173104415,-81.5548874755347,-45.5866585651915));
#24340=CARTESIAN_POINT('Ctrl Pts',(149.7370901728,-81.6094178533078,-45.6160154789332));
#24341=CARTESIAN_POINT('Ctrl Pts',(149.721679195218,-81.6668165155371,-45.6469165591158));
#24342=CARTESIAN_POINT('Ctrl Pts',(149.706091100881,-81.7247936014321,-45.6765660851853));
#24343=CARTESIAN_POINT('Ctrl Pts',(149.690345642873,-81.7832715016962,-45.7051731327433));
#24344=CARTESIAN_POINT('Ctrl Pts',(149.684002656688,-81.8068290579963,-45.7166973518138));
#24345=CARTESIAN_POINT('Ctrl Pts',(149.67763399788,-81.8304683944407,-45.7280520707485));
#24346=CARTESIAN_POINT('Ctrl Pts',(149.671240444102,-81.854186356593,-45.7392497349255));
#24347=CARTESIAN_POINT('Ctrl Pts',(149.663115656512,-81.8843266214971,-45.7534794803999));
#24348=CARTESIAN_POINT('Ctrl Pts',(149.654955183208,-81.9145791058626,-45.7674477491405));
#24349=CARTESIAN_POINT('Ctrl Pts',(149.646761444289,-81.9449339838539,-45.7811773107384));
#24350=CARTESIAN_POINT('Ctrl Pts',(149.629599044989,-82.0085145472401,-45.8099349048783));
#24351=CARTESIAN_POINT('Ctrl Pts',(149.612256027528,-82.0726719053374,-45.8376821506386));
#24352=CARTESIAN_POINT('Ctrl Pts',(149.594776281623,-82.1372383448953,-45.8645156723128));
#24353=CARTESIAN_POINT('Ctrl Pts',(149.57592605508,-82.2068670465535,-45.8934530473311));
#24354=CARTESIAN_POINT('Ctrl Pts',(149.556916727547,-82.2769718987423,-45.9213279816653));
#24355=CARTESIAN_POINT('Ctrl Pts',(149.537787182918,-82.3473991049663,-45.9482460618992));
#24356=CARTESIAN_POINT('Ctrl Pts',(149.532245072383,-82.3678029028159,-45.9560446257929));
#24357=CARTESIAN_POINT('Ctrl Pts',(149.526692780135,-82.3882340721267,-45.9637627732937));
#24358=CARTESIAN_POINT('Ctrl Pts',(149.521131044556,-82.4086895813368,-45.9714028195526));
#24359=CARTESIAN_POINT('Ctrl Pts',(149.513307047732,-82.4374654619684,-45.9821504893812));
#24360=CARTESIAN_POINT('Ctrl Pts',(149.505462657808,-82.4662967316413,-45.9927459306726));
#24361=CARTESIAN_POINT('Ctrl Pts',(149.497602582526,-82.4951656239004,-46.0031912460791));
#24362=CARTESIAN_POINT('Ctrl Pts',(149.466886299739,-82.6079819808148,-46.0440103540796));
#24363=CARTESIAN_POINT('Ctrl Pts',(149.435949796432,-82.721306238521,-46.0825462658463));
#24364=CARTESIAN_POINT('Ctrl Pts',(149.404819096531,-82.8350358342389,-46.1191658716245));
#24365=CARTESIAN_POINT('Ctrl Pts',(149.382928718768,-82.9150078175565,-46.1449159192168));
#24366=CARTESIAN_POINT('Ctrl Pts',(149.360942099001,-82.995181007926,-46.169717455523));
#24367=CARTESIAN_POINT('Ctrl Pts',(149.338865605393,-83.0755291035976,-46.193686300737));
#24368=CARTESIAN_POINT('Ctrl Pts',(149.30257270251,-83.2076182697843,-46.233090156576));
#24369=CARTESIAN_POINT('Ctrl Pts',(149.266041574139,-83.3401623692395,-46.2702654172594));
#24370=CARTESIAN_POINT('Ctrl Pts',(149.229255373738,-83.4732146574125,-46.3055170512346));
#24371=CARTESIAN_POINT('Ctrl Pts',(149.222100057115,-83.4990947765572,-46.3123738779743));
#24372=CARTESIAN_POINT('Ctrl Pts',(149.214935059986,-83.5249942184406,-46.3191578024711));
#24373=CARTESIAN_POINT('Ctrl Pts',(149.207760216038,-83.5509135089673,-46.3258708967128));
#24374=CARTESIAN_POINT('Ctrl Pts',(149.164019348336,-83.7089284102155,-46.366796743915));
#24375=CARTESIAN_POINT('Ctrl Pts',(149.119950314816,-83.8675446159544,-46.4050588777709));
#24376=CARTESIAN_POINT('Ctrl Pts',(149.075578120339,-84.0266555943282,-46.4410493230434));
#24377=CARTESIAN_POINT('Ctrl Pts',(149.050851325548,-84.1153215834145,-46.4611053145304));
#24378=CARTESIAN_POINT('Ctrl Pts',(149.026030206988,-84.2041418314762,-46.4804550867179));
#24379=CARTESIAN_POINT('Ctrl Pts',(149.001117827171,-84.2931021083258,-46.4991611413161));
#24380=CARTESIAN_POINT('Ctrl Pts',(148.961812515426,-84.4334584869728,-46.5286744721549));
#24381=CARTESIAN_POINT('Ctrl Pts',(148.922228706232,-84.5743409203763,-46.5565824640166));
#24382=CARTESIAN_POINT('Ctrl Pts',(148.882458149795,-84.7154243069172,-46.58297626425));
#24383=CARTESIAN_POINT('Ctrl Pts',(148.823378480021,-84.9250054803839,-46.6221845917561));
#24384=CARTESIAN_POINT('Ctrl Pts',(148.763691428381,-85.1357176965639,-46.658180607518));
#24385=CARTESIAN_POINT('Ctrl Pts',(148.703725142332,-85.346373256235,-46.6911268937745));
#24386=CARTESIAN_POINT('Ctrl Pts',(148.683093735236,-85.4188493239555,-46.7024620670668));
#24387=CARTESIAN_POINT('Ctrl Pts',(148.662429146923,-85.4913191022908,-46.7134360383522));
#24388=CARTESIAN_POINT('Ctrl Pts',(148.64174438629,-85.5637353575988,-46.7240548006858));
#24389=CARTESIAN_POINT('Ctrl Pts',(148.565624143843,-85.8302283090543,-46.7631320120529));
#24390=CARTESIAN_POINT('Ctrl Pts',(148.489028565031,-86.0967324995911,-46.7975654258511));
#24391=CARTESIAN_POINT('Ctrl Pts',(148.411875341988,-86.3635238183437,-46.8277812265461));
#24392=CARTESIAN_POINT('Ctrl Pts',(148.365096720961,-86.5252815453832,-46.846101310063));
#24393=CARTESIAN_POINT('Ctrl Pts',(148.318112978006,-86.6871449972432,-46.8628698580675));
#24394=CARTESIAN_POINT('Ctrl Pts',(148.270904619886,-86.8491769961467,-46.8781728422293));
#24395=CARTESIAN_POINT('Ctrl Pts',(148.24918654488,-86.9237193705385,-46.8852129379044));
#24396=CARTESIAN_POINT('Ctrl Pts',(148.227421070419,-86.9982969676292,-46.8919477958447));
#24397=CARTESIAN_POINT('Ctrl Pts',(148.205605817643,-87.0729174681581,-46.8983780579096));
#24398=CARTESIAN_POINT('Ctrl Pts',(148.10190068443,-87.42764766667,-46.9289461742125));
#24399=CARTESIAN_POINT('Ctrl Pts',(147.997167488693,-87.7829762387816,-46.9525973445083));
#24400=CARTESIAN_POINT('Ctrl Pts',(147.891499227195,-88.1385323929249,-46.969351029831));
#24401=CARTESIAN_POINT('Ctrl Pts',(147.785745335364,-88.4943766789206,-46.9861182918287));
#24402=CARTESIAN_POINT('Ctrl Pts',(147.679054863979,-88.8504488649393,-46.9959768816863));
#24403=CARTESIAN_POINT('Ctrl Pts',(147.571529965735,-89.2063722196095,-46.9989975290796));
#24404=CARTESIAN_POINT('Ctrl Pts',(147.547727111398,-89.285163196442,-46.9996662116924));
#24405=CARTESIAN_POINT('Ctrl Pts',(147.523883400528,-89.3639468619846,-47.));
#24406=CARTESIAN_POINT('Ctrl Pts',(147.5,-89.4427190999916,-47.));
#24407=CARTESIAN_POINT('Origin',(115.217186218029,-122.5,-49.5));
#24408=CARTESIAN_POINT('Origin',(147.5,-122.5,-49.5));
#24409=CARTESIAN_POINT('Origin',(115.217186218029,-127.5,82.5));
#24410=CARTESIAN_POINT('Ctrl Pts',(116.189500386223,-127.5,85.));
#24411=CARTESIAN_POINT('Ctrl Pts',(116.448008540164,-127.382212026451,85.));
#24412=CARTESIAN_POINT('Ctrl Pts',(116.70545859626,-127.26417086413,84.9919054816509));
#24413=CARTESIAN_POINT('Ctrl Pts',(116.961798715612,-127.145925914751,84.9750282599701));
#24414=CARTESIAN_POINT('Ctrl Pts',(117.203993376622,-127.034206003318,84.9590823635802));
#24415=CARTESIAN_POINT('Ctrl Pts',(117.44519709308,-126.922304463616,84.9352961059057));
#24416=CARTESIAN_POINT('Ctrl Pts',(117.685352827265,-126.810270254864,84.9030396161985));
#24417=CARTESIAN_POINT('Ctrl Pts',(117.699379201419,-126.803726860281,84.9011556653736));
#24418=CARTESIAN_POINT('Ctrl Pts',(117.713401997064,-126.797183014578,84.8992428067277));
#24419=CARTESIAN_POINT('Ctrl Pts',(117.727421201483,-126.790638727994,84.897300909382));
#24420=CARTESIAN_POINT('Ctrl Pts',(117.801716706967,-126.755956939695,84.8870097230499));
#24421=CARTESIAN_POINT('Ctrl Pts',(117.875811770813,-126.721306222531,84.8759163529931));
#24422=CARTESIAN_POINT('Ctrl Pts',(117.949766484243,-126.686659174451,84.8639959183815));
#24423=CARTESIAN_POINT('Ctrl Pts',(118.06803595945,-126.631251100998,84.8449325824511));
#24424=CARTESIAN_POINT('Ctrl Pts',(118.186129688142,-126.575765453057,84.8236742085113));
#24425=CARTESIAN_POINT('Ctrl Pts',(118.304009972734,-126.520223268699,84.8000156545051));
#24426=CARTESIAN_POINT('Ctrl Pts',(118.414673338094,-126.468081512665,84.7778055350189));
#24427=CARTESIAN_POINT('Ctrl Pts',(118.525149041361,-126.41588969173,84.7534800370994));
#24428=CARTESIAN_POINT('Ctrl Pts',(118.635381578924,-126.363674712089,84.7268318520061));
#24429=CARTESIAN_POINT('Ctrl Pts',(118.688420413194,-126.338551262036,84.714009969248));
#24430=CARTESIAN_POINT('Ctrl Pts',(118.741402540217,-126.313422617291,84.7006497952873));
#24431=CARTESIAN_POINT('Ctrl Pts',(118.794319125548,-126.288292874885,84.6867249125825));
#24432=CARTESIAN_POINT('Ctrl Pts',(118.899018286902,-126.238571923722,84.6591735592211));
#24433=CARTESIAN_POINT('Ctrl Pts',(119.002876811871,-126.189124992078,84.6295858023581));
#24434=CARTESIAN_POINT('Ctrl Pts',(119.105920148838,-126.139946013067,84.5977086876102));
#24435=CARTESIAN_POINT('Ctrl Pts',(119.148229575818,-126.119753204074,84.5846199960125));
#24436=CARTESIAN_POINT('Ctrl Pts',(119.190401214644,-126.099605728966,84.5711448947681));
#24437=CARTESIAN_POINT('Ctrl Pts',(119.232435280194,-126.079503870074,84.5572639252337));
#24438=CARTESIAN_POINT('Ctrl Pts',(119.332253758341,-126.031767898399,84.5243007265521));
#24439=CARTESIAN_POINT('Ctrl Pts',(119.431308801167,-125.984284516995,84.4890488616751));
#24440=CARTESIAN_POINT('Ctrl Pts',(119.529560384222,-125.937075343632,84.4512249355722));
#24441=CARTESIAN_POINT('Ctrl Pts',(119.549179492571,-125.927648504302,84.4436721646005));
#24442=CARTESIAN_POINT('Ctrl Pts',(119.56876646678,-125.918232645463,84.4360167122299));
#24443=CARTESIAN_POINT('Ctrl Pts',(119.588320838716,-125.908828011419,84.4282561299977));
#24444=CARTESIAN_POINT('Ctrl Pts',(119.676176605169,-125.866573965376,84.3933886383497));
#24445=CARTESIAN_POINT('Ctrl Pts',(119.763367640996,-125.82454975495,84.3563903280491));
#24446=CARTESIAN_POINT('Ctrl Pts',(119.849778269297,-125.782813941846,84.3169432875038));
#24447=CARTESIAN_POINT('Ctrl Pts',(119.88415418401,-125.766210582052,84.3012504482301));
#24448=CARTESIAN_POINT('Ctrl Pts',(119.918406261816,-125.749653027032,84.2851696439165));
#24449=CARTESIAN_POINT('Ctrl Pts',(119.952525858354,-125.73314564101,84.2686790921243));
#24450=CARTESIAN_POINT('Ctrl Pts',(119.95435634409,-125.732260034563,84.2677943888189));
#24451=CARTESIAN_POINT('Ctrl Pts',(119.956186462171,-125.731374563089,84.2669084964009));
#24452=CARTESIAN_POINT('Ctrl Pts',(119.958016213969,-125.730489226021,84.2660214100548));
#24453=CARTESIAN_POINT('Ctrl Pts',(120.016911873286,-125.701992185948,84.2374680645808));
#24454=CARTESIAN_POINT('Ctrl Pts',(120.075514267379,-125.673592123274,84.2076160589798));
#24455=CARTESIAN_POINT('Ctrl Pts',(120.133520234546,-125.645440552611,84.1764738678677));
#24456=CARTESIAN_POINT('Ctrl Pts',(120.185326529706,-125.620297819024,84.1486601510473));
#24457=CARTESIAN_POINT('Ctrl Pts',(120.236657062466,-125.595353295122,84.1198170381164));
#24458=CARTESIAN_POINT('Ctrl Pts',(120.287252932459,-125.570735521273,84.0899486390561));
#24459=CARTESIAN_POINT('Ctrl Pts',(120.29330775259,-125.567789506258,84.0863742804385));
#24460=CARTESIAN_POINT('Ctrl Pts',(120.299351995964,-125.564848197438,84.0827852387161));
#24461=CARTESIAN_POINT('Ctrl Pts',(120.305385171907,-125.561911837745,84.0791815213283));
#24462=CARTESIAN_POINT('Ctrl Pts',(120.36056980737,-125.535053357114,84.046218811097));
#24463=CARTESIAN_POINT('Ctrl Pts',(120.414989618081,-125.508531012063,84.0119891408571));
#24464=CARTESIAN_POINT('Ctrl Pts',(120.468555276,-125.482393019785,83.9762964268862));
#24465=CARTESIAN_POINT('Ctrl Pts',(120.521845432222,-125.456389461797,83.9407872895508));
#24466=CARTESIAN_POINT('Ctrl Pts',(120.574290544872,-125.430766130924,83.9038303719441));
#24467=CARTESIAN_POINT('Ctrl Pts',(120.625763505242,-125.405589684656,83.8652058122217));
#24468=CARTESIAN_POINT('Ctrl Pts',(120.669724343261,-125.38408756649,83.8322182396925));
#24469=CARTESIAN_POINT('Ctrl Pts',(120.712919977829,-125.362939699079,83.798058607416));
#24470=CARTESIAN_POINT('Ctrl Pts',(120.755308589242,-125.342167431342,83.7625256624148));
#24471=CARTESIAN_POINT('Ctrl Pts',(120.796119057626,-125.322168522496,83.7283156215514));
#24472=CARTESIAN_POINT('Ctrl Pts',(120.836181594618,-125.302517695486,83.6928327066558));
#24473=CARTESIAN_POINT('Ctrl Pts',(120.87542145341,-125.283252598435,83.6558720771839));
#24474=CARTESIAN_POINT('Ctrl Pts',(120.882694505626,-125.279681839999,83.649021476893));
#24475=CARTESIAN_POINT('Ctrl Pts',(120.889939185317,-125.276124387987,83.6421200366677));
#24476=CARTESIAN_POINT('Ctrl Pts',(120.897154862446,-125.27258055919,83.6351663481078));
#24477=CARTESIAN_POINT('Ctrl Pts',(120.930420737947,-125.256242720701,83.603108298149));
#24478=CARTESIAN_POINT('Ctrl Pts',(120.962969894054,-125.240243618606,83.5699873690875));
#24479=CARTESIAN_POINT('Ctrl Pts',(120.994602600081,-125.224682872253,83.5357995420131));
#24480=CARTESIAN_POINT('Ctrl Pts',(121.024642658856,-125.209905580212,83.5033330077298));
#24481=CARTESIAN_POINT('Ctrl Pts',(121.053856347428,-125.195523551178,83.4699041218694));
#24482=CARTESIAN_POINT('Ctrl Pts',(121.082031519346,-125.181642679555,83.4355171688528));
#24483=CARTESIAN_POINT('Ctrl Pts',(121.097985602281,-125.173782689287,83.416045688717));
#24484=CARTESIAN_POINT('Ctrl Pts',(121.113605937311,-125.166083770035,83.3962671745771));
#24485=CARTESIAN_POINT('Ctrl Pts',(121.1288474274,-125.158568448299,83.3761839355069));
#24486=CARTESIAN_POINT('Ctrl Pts',(121.149706220237,-125.148283329307,83.3486989507179));
#24487=CARTESIAN_POINT('Ctrl Pts',(121.169911626188,-125.138314491271,83.3205937206656));
#24488=CARTESIAN_POINT('Ctrl Pts',(121.189383694812,-125.128702127376,83.2918112814197));
#24489=CARTESIAN_POINT('Ctrl Pts',(121.219288926705,-125.113939444639,83.2476071685062));
#24490=CARTESIAN_POINT('Ctrl Pts',(121.247502565816,-125.100002690991,83.201750806387));
#24491=CARTESIAN_POINT('Ctrl Pts',(121.273533474621,-125.08713705486,83.154295706818));
#24492=CARTESIAN_POINT('Ctrl Pts',(121.283706281684,-125.082109199894,83.1357503853428));
#24493=CARTESIAN_POINT('Ctrl Pts',(121.293546196337,-125.07724471837,83.1169610515117));
#24494=CARTESIAN_POINT('Ctrl Pts',(121.303025858184,-125.072557339689,83.0979315436973));
#24495=CARTESIAN_POINT('Ctrl Pts',(121.323095906417,-125.062633365845,83.0576428555715));
#24496=CARTESIAN_POINT('Ctrl Pts',(121.341528989802,-125.053514201567,83.0161861527192));
#24497=CARTESIAN_POINT('Ctrl Pts',(121.357996565716,-125.045363893225,82.9739496378786));
#24498=CARTESIAN_POINT('Ctrl Pts',(121.365145493259,-125.041825669743,82.9556138618141));
#24499=CARTESIAN_POINT('Ctrl Pts',(121.371924242049,-125.038469923387,82.9371317587732));
#24500=CARTESIAN_POINT('Ctrl Pts',(121.378307256224,-125.035309443556,82.9185377169621));
#24501=CARTESIAN_POINT('Ctrl Pts',(121.391447468896,-125.028803210607,82.8802596155576));
#24502=CARTESIAN_POINT('Ctrl Pts',(121.402999576331,-125.02308111907,82.8412451545452));
#24503=CARTESIAN_POINT('Ctrl Pts',(121.41267276749,-125.018288884737,82.8018442319798));
#24504=CARTESIAN_POINT('Ctrl Pts',(121.422709757883,-125.013316419171,82.7609614793595));
#24505=CARTESIAN_POINT('Ctrl Pts',(121.430817047113,-125.009299023442,82.7195176678589));
#24506=CARTESIAN_POINT('Ctrl Pts',(121.43683910078,-125.006314500199,82.6776303050308));
#24507=CARTESIAN_POINT('Ctrl Pts',(121.442766130939,-125.003377070502,82.6364038934916));
#24508=CARTESIAN_POINT('Ctrl Pts',(121.446673152333,-125.001440207745,82.5947478151296));
#24509=CARTESIAN_POINT('Ctrl Pts',(121.448457146603,-125.000555735143,82.5527767557765));
#24510=CARTESIAN_POINT('Ctrl Pts',(121.449202695032,-125.000186105503,82.5352366448472));
#24511=CARTESIAN_POINT('Ctrl Pts',(121.449578014743,-125.,82.5176415554239));
#24512=CARTESIAN_POINT('Ctrl Pts',(121.449578014911,-125.,82.5));
#24513=CARTESIAN_POINT('Origin',(0.,0.,87.5));
#24514=CARTESIAN_POINT('Origin',(116.189500386222,-127.5,87.5));
#24515=CARTESIAN_POINT('Ctrl Pts',(150.289855072464,-79.4541343310581,-44.5));
#24516=CARTESIAN_POINT('Ctrl Pts',(150.,-80.0024038100394,-44.5));
#24517=CARTESIAN_POINT('Ctrl Pts',(150.,-80.6225774829855,-44.5));
#24518=CARTESIAN_POINT('Ctrl Pts',(150.28985506853,-79.4541343384987,-44.7594238560556));
#24519=CARTESIAN_POINT('Ctrl Pts',(149.999999996126,-80.0024038172978,-44.6905851824362));
#24520=CARTESIAN_POINT('Ctrl Pts',(150.,-80.6225774905387,-44.629711927975));
#24521=CARTESIAN_POINT('Ctrl Pts',(150.270119749701,-79.4914922605508,-45.0111695802387));
#24522=CARTESIAN_POINT('Ctrl Pts',(149.980519833119,-80.0389466368966,-44.8758156770736));
#24523=CARTESIAN_POINT('Ctrl Pts',(149.989987226484,-80.6604847938369,-44.7555847901951));
#24524=CARTESIAN_POINT('Ctrl Pts',(150.196231486305,-79.6310132970258,-45.5012087006257));
#24525=CARTESIAN_POINT('Ctrl Pts',(149.907890955038,-80.1748646486434,-45.2336047942099));
#24526=CARTESIAN_POINT('Ctrl Pts',(149.952499797667,-80.8020576101747,-45.0006043502371));
#24527=CARTESIAN_POINT('Ctrl Pts',(150.143050717941,-79.7313168859281,-45.7320003431406));
#24528=CARTESIAN_POINT('Ctrl Pts',(149.855501091412,-80.272795283317,-45.4011397919881));
#24529=CARTESIAN_POINT('Ctrl Pts',(149.925518380098,-80.9038362519448,-45.1160001719023));
#24530=CARTESIAN_POINT('Ctrl Pts',(150.01502846971,-79.971931353987,-46.1617150079383));
#24531=CARTESIAN_POINT('Ctrl Pts',(149.729850869406,-80.506872138187,-45.7093793927994));
#24532=CARTESIAN_POINT('Ctrl Pts',(149.860565913637,-81.1479891679691,-45.3308575036371));
#24533=CARTESIAN_POINT('Ctrl Pts',(149.939105635844,-80.1142600764838,-46.3637363656926));
#24534=CARTESIAN_POINT('Ctrl Pts',(149.655266820466,-80.6454659182033,-45.8524984192499));
#24535=CARTESIAN_POINT('Ctrl Pts',(149.8220462428,-81.2924109599909,-45.4318681833206));
#24536=CARTESIAN_POINT('Ctrl Pts',(149.775363670977,-80.4199633406152,-46.7336380224264));
#24537=CARTESIAN_POINT('Ctrl Pts',(149.494928348598,-80.9422362487695,-46.1103934277676));
#24538=CARTESIAN_POINT('Ctrl Pts',(149.738971273161,-81.6026098603007,-45.616819010739));
#24539=CARTESIAN_POINT('Ctrl Pts',(149.686995608736,-80.5843780010491,-46.903585266663));
#24540=CARTESIAN_POINT('Ctrl Pts',(149.408398325687,-81.1018541496878,-46.2266925752405));
#24541=CARTESIAN_POINT('Ctrl Pts',(149.694137478568,-81.7694423834459,-45.7017926336777));
#24542=CARTESIAN_POINT('Ctrl Pts',(149.500255462679,-80.9302925286903,-47.2210941330543));
#24543=CARTESIAN_POINT('Ctrl Pts',(149.226078269656,-81.4367533718067,-46.4395269094013));
#24544=CARTESIAN_POINT('Ctrl Pts',(149.599394315017,-82.1204438893779,-45.8605470661809));
#24545=CARTESIAN_POINT('Ctrl Pts',(149.401347886678,-81.1127763961003,-47.369210707149));
#24546=CARTESIAN_POINT('Ctrl Pts',(149.129574349821,-81.6133256610688,-46.5363235480013));
#24547=CARTESIAN_POINT('Ctrl Pts',(149.549213266548,-82.3056113431187,-45.9346053539496));
#24548=CARTESIAN_POINT('Ctrl Pts',(149.197899201605,-81.4863922312653,-47.6435514113241));
#24549=CARTESIAN_POINT('Ctrl Pts',(148.93165319989,-81.9738530462045,-46.7107456147876));
#24550=CARTESIAN_POINT('Ctrl Pts',(149.445992976772,-82.684721528767,-46.071775705287));
#24551=CARTESIAN_POINT('Ctrl Pts',(149.093462145135,-81.6773447374821,-47.7698090460946));
#24552=CARTESIAN_POINT('Ctrl Pts',(148.830186520417,-82.1578926315274,-46.7883037911384));
#24553=CARTESIAN_POINT('Ctrl Pts',(149.393006529828,-82.8784821601051,-46.1349045233201));
#24554=CARTESIAN_POINT('Ctrl Pts',(148.773324875584,-82.2599185303359,-48.1224993059861));
#24555=CARTESIAN_POINT('Ctrl Pts',(148.518202139789,-82.721231742148,-46.9985052310704));
#24556=CARTESIAN_POINT('Ctrl Pts',(149.230583943609,-83.4696232145796,-46.3112496524474));
#24557=CARTESIAN_POINT('Ctrl Pts',(148.550873607932,-82.6611103319713,-48.3232112727545));
#24558=CARTESIAN_POINT('Ctrl Pts',(148.30315471628,-83.1060920248234,-47.1056075630378));
#24559=CARTESIAN_POINT('Ctrl Pts',(149.117722639557,-83.8767148956951,-46.4116056366651));
#24560=CARTESIAN_POINT('Ctrl Pts',(148.091214058598,-83.4818155626998,-48.6734332925097));
#24561=CARTESIAN_POINT('Ctrl Pts',(147.862495369544,-83.8874214153556,-47.2694844772005));
#24562=CARTESIAN_POINT('Ctrl Pts',(148.884513014786,-84.7094893209564,-46.586716645967));
#24563=CARTESIAN_POINT('Ctrl Pts',(147.853104568995,-83.9028862659541,-48.8228865658125));
#24564=CARTESIAN_POINT('Ctrl Pts',(147.635229789707,-84.286581928446,-47.3247069198698));
#24565=CARTESIAN_POINT('Ctrl Pts',(148.763707465283,-85.1367522404598,-46.6614432831528));
#24566=CARTESIAN_POINT('Ctrl Pts',(147.37234266623,-84.7444834282146,-49.073322172108));
#24567=CARTESIAN_POINT('Ctrl Pts',(147.180928816256,-85.0771956930355,-47.3874171310308));
#24568=CARTESIAN_POINT('Ctrl Pts',(148.519791499647,-85.9907258315643,-46.7866610858075));
#24569=CARTESIAN_POINT('Ctrl Pts',(147.128665473946,-85.166872640511,-49.1751382031672));
#24570=CARTESIAN_POINT('Ctrl Pts',(146.952267516978,-85.4713149459694,-47.3939268980417));
#24571=CARTESIAN_POINT('Ctrl Pts',(148.396161159612,-86.4193266499342,-46.837569101695));
#24572=CARTESIAN_POINT('Ctrl Pts',(146.388097896077,-86.4377602232181,-49.41873440213));
#24573=CARTESIAN_POINT('Ctrl Pts',(146.253862108763,-86.6644852388405,-47.3459550909554));
#24574=CARTESIAN_POINT('Ctrl Pts',(148.020432020732,-87.7089037559046,-46.9593672008422));
#24575=CARTESIAN_POINT('Ctrl Pts',(145.881711078451,-87.289917999924,-49.4999999990937));
#24576=CARTESIAN_POINT('Ctrl Pts',(145.791767290438,-87.4382443129923,-47.2157310733627));
#24577=CARTESIAN_POINT('Ctrl Pts',(147.763515165397,-88.573593311031,-47.));
#24578=CARTESIAN_POINT('Ctrl Pts',(145.36231884058,-88.1464478086874,-49.5));
#24579=CARTESIAN_POINT('Ctrl Pts',(145.36231884058,-88.1464478086874,-46.9999999999999));
#24580=CARTESIAN_POINT('Ctrl Pts',(147.5,-89.4427190999917,-47.));
#24581=CARTESIAN_POINT('Origin',(152.5,-80.6225774829854,-44.5));
#24582=CARTESIAN_POINT('Origin',(147.5,-122.5,-44.5));
#24583=CARTESIAN_POINT('Origin',(152.5,-122.5,-44.5));
#24584=CARTESIAN_POINT('Ctrl Pts',(114.505594583524,-125.652173913043,87.5));
#24585=CARTESIAN_POINT('Ctrl Pts',(114.505594583524,-125.652173913043,85.));
#24586=CARTESIAN_POINT('Ctrl Pts',(116.189500386223,-127.5,85.));
#24587=CARTESIAN_POINT('Ctrl Pts',(115.098666513066,-125.111713276286,87.4999999993277));
#24588=CARTESIAN_POINT('Ctrl Pts',(114.980468455817,-125.219426007098,84.789197137563));
#24589=CARTESIAN_POINT('Ctrl Pts',(116.791295074219,-127.225795199451,85.));
#24590=CARTESIAN_POINT('Ctrl Pts',(115.677248330338,-124.576762485165,87.412213589489));
#24591=CARTESIAN_POINT('Ctrl Pts',(115.390477170759,-124.841163526176,84.4869181320052));
#24592=CARTESIAN_POINT('Ctrl Pts',(117.378384335167,-126.95438684931,84.9561067940497));
#24593=CARTESIAN_POINT('Ctrl Pts',(116.521921487207,-123.785260415245,87.135895140949));
#24594=CARTESIAN_POINT('Ctrl Pts',(115.879476439134,-124.389591527255,83.9347335464724));
#24595=CARTESIAN_POINT('Ctrl Pts',(118.235479156151,-126.55281594586,84.8179475708219));
#24596=CARTESIAN_POINT('Ctrl Pts',(116.800657852356,-123.522253316268,87.0187226097786));
#24597=CARTESIAN_POINT('Ctrl Pts',(116.025791458688,-124.254393807365,83.7225655755012));
#24598=CARTESIAN_POINT('Ctrl Pts',(118.51831458544,-126.419378520877,84.7593613046283));
#24599=CARTESIAN_POINT('Ctrl Pts',(117.344689694216,-123.005546784036,86.728197778466));
#24600=CARTESIAN_POINT('Ctrl Pts',(116.260513692635,-124.039299071365,83.2680355386732));
#24601=CARTESIAN_POINT('Ctrl Pts',(119.07034689564,-126.157225941778,84.614098889494));
#24602=CARTESIAN_POINT('Ctrl Pts',(117.605972114118,-122.755671483612,86.5572347078813));
#24603=CARTESIAN_POINT('Ctrl Pts',(116.343854196171,-123.964200078231,83.0270891162914));
#24604=CARTESIAN_POINT('Ctrl Pts',(119.335471703983,-126.03045097373,84.5286173533875));
#24605=CARTESIAN_POINT('Ctrl Pts',(117.979759695143,-122.396103662867,86.2561620132639));
#24606=CARTESIAN_POINT('Ctrl Pts',(116.408893575195,-123.910132089279,82.6723188019316));
#24607=CARTESIAN_POINT('Ctrl Pts',(119.714756161272,-125.848023181682,84.3780810069086));
#24608=CARTESIAN_POINT('Ctrl Pts',(118.101314578112,-122.278806587615,86.1483179654515));
#24609=CARTESIAN_POINT('Ctrl Pts',(116.420127652017,-123.902387828605,82.5524859464439));
#24610=CARTESIAN_POINT('Ctrl Pts',(119.838098616002,-125.788512166127,84.3241589823631));
#24611=CARTESIAN_POINT('Ctrl Pts',(118.337674566632,-122.050079163152,85.9157683721022));
#24612=CARTESIAN_POINT('Ctrl Pts',(116.419552940987,-123.909688381786,82.3194835992922));
#24613=CARTESIAN_POINT('Ctrl Pts',(120.077934486753,-125.672466633894,84.2078841864137));
#24614=CARTESIAN_POINT('Ctrl Pts',(118.452813811185,-121.938320691333,85.7905474845089));
#24615=CARTESIAN_POINT('Ctrl Pts',(116.406751222331,-123.925725220725,82.2063383456538));
#24616=CARTESIAN_POINT('Ctrl Pts',(120.194766955428,-125.615765645109,84.1452737420412));
#24617=CARTESIAN_POINT('Ctrl Pts',(118.779955786451,-121.619960181736,85.394093024668));
#24618=CARTESIAN_POINT('Ctrl Pts',(116.330634260051,-124.011396018777,81.8918489994272));
#24619=CARTESIAN_POINT('Ctrl Pts',(120.526719842212,-125.454244503486,83.9470465127606));
#24620=CARTESIAN_POINT('Ctrl Pts',(118.976188771633,-121.427849190967,85.1007432598139));
#24621=CARTESIAN_POINT('Ctrl Pts',(116.22633468612,-124.12159432885,81.7284336163675));
#24622=CARTESIAN_POINT('Ctrl Pts',(120.725838606435,-125.356776429138,83.8003716291908));
#24623=CARTESIAN_POINT('Ctrl Pts',(119.229508592988,-121.178951530852,84.6051856591982));
#24624=CARTESIAN_POINT('Ctrl Pts',(116.018327623081,-124.338324238802,81.6176595477783));
#24625=CARTESIAN_POINT('Ctrl Pts',(120.982883719393,-125.230497467175,83.5525928299572));
#24626=CARTESIAN_POINT('Ctrl Pts',(119.306430749593,-121.103197399825,84.4313845009826));
#24627=CARTESIAN_POINT('Ctrl Pts',(115.938944698972,-124.420612015483,81.6055951047046));
#24628=CARTESIAN_POINT('Ctrl Pts',(121.060937084102,-125.192063387035,83.4656922503483));
#24629=CARTESIAN_POINT('Ctrl Pts',(119.440303841193,-120.971164568222,84.0733653040093));
#24630=CARTESIAN_POINT('Ctrl Pts',(115.778652442948,-124.586368326784,81.6400246699492));
#24631=CARTESIAN_POINT('Ctrl Pts',(121.196778897725,-125.125076140871,83.2866826521477));
#24632=CARTESIAN_POINT('Ctrl Pts',(119.497839395062,-120.914311737672,83.8880856770355));
#24633=CARTESIAN_POINT('Ctrl Pts',(115.697759348993,-124.669813047928,81.687827278078));
#24634=CARTESIAN_POINT('Ctrl Pts',(121.255160562605,-125.096231691082,83.1940428383536));
#24635=CARTESIAN_POINT('Ctrl Pts',(119.592195409222,-120.820988244119,83.5036466079772));
#24636=CARTESIAN_POINT('Ctrl Pts',(115.551887637631,-124.820142027722,81.8435231238131));
#24637=CARTESIAN_POINT('Ctrl Pts',(121.350904165271,-125.048883740856,83.0018233041528));
#24638=CARTESIAN_POINT('Ctrl Pts',(119.628897626029,-120.784634828299,83.3034927483087));
#24639=CARTESIAN_POINT('Ctrl Pts',(115.488159523431,-124.885734117079,81.9531151909441));
#24640=CARTESIAN_POINT('Ctrl Pts',(121.388146120508,-125.030439729044,82.9017463741549));
#24641=CARTESIAN_POINT('Ctrl Pts',(119.677240002648,-120.736735847766,82.9038841796106));
#24642=CARTESIAN_POINT('Ctrl Pts',(115.400689666877,-124.975740417798,82.2081803578444));
#24643=CARTESIAN_POINT('Ctrl Pts',(121.437199414473,-125.006138040429,82.7019420898048));
#24644=CARTESIAN_POINT('Ctrl Pts',(119.689439202153,-120.724637682099,82.7026620014997));
#24645=CARTESIAN_POINT('Ctrl Pts',(115.37709911597,-124.99999999812,82.3529550603214));
#24646=CARTESIAN_POINT('Ctrl Pts',(121.449578013946,-125.,82.6013310007504));
#24647=CARTESIAN_POINT('Ctrl Pts',(119.689439203101,-120.724637681159,82.5));
#24648=CARTESIAN_POINT('Ctrl Pts',(115.377099114166,-125.,82.5));
#24649=CARTESIAN_POINT('Ctrl Pts',(121.449578014911,-125.,82.5));
#24650=CARTESIAN_POINT('Origin',(152.5,-80.6225774829854,115.));
#24651=CARTESIAN_POINT('Origin',(152.5,-80.6225774829854,-37.5));
#24652=CARTESIAN_POINT('Origin',(147.5,-79.9999999999999,-37.5));
#24653=CARTESIAN_POINT('Origin',(147.5,-122.5,-37.5));
#24654=CARTESIAN_POINT('Ctrl Pts',(147.5,-89.4427190999916,-35.));
#24655=CARTESIAN_POINT('Ctrl Pts',(147.692029124325,-88.8093685907339,-35.));
#24656=CARTESIAN_POINT('Ctrl Pts',(147.88101932576,-88.1768396514604,-35.0215706395705));
#24657=CARTESIAN_POINT('Ctrl Pts',(148.067032922317,-87.5451886182185,-35.0650289615107));
#24658=CARTESIAN_POINT('Ctrl Pts',(148.113199638342,-87.3884191432013,-35.0758148827823));
#24659=CARTESIAN_POINT('Ctrl Pts',(148.159182993898,-87.2317038211986,-35.0879492852677));
#24660=CARTESIAN_POINT('Ctrl Pts',(148.204983936061,-87.0750436647327,-35.1014374973016));
#24661=CARTESIAN_POINT('Ctrl Pts',(148.227650188963,-86.9975147197266,-35.1081126269108));
#24662=CARTESIAN_POINT('Ctrl Pts',(148.250265804086,-86.9200215223735,-35.115117542436));
#24663=CARTESIAN_POINT('Ctrl Pts',(148.272833473781,-86.8425552539345,-35.1224532765259));
#24664=CARTESIAN_POINT('Ctrl Pts',(148.349179005424,-86.5804899397761,-35.1472697740491));
#24665=CARTESIAN_POINT('Ctrl Pts',(148.42497434187,-86.3187382385474,-35.1759312643129));
#24666=CARTESIAN_POINT('Ctrl Pts',(148.500300623548,-86.0570314558247,-35.2088246089286));
#24667=CARTESIAN_POINT('Ctrl Pts',(148.548487711965,-85.8896146180706,-35.2298668596546));
#24668=CARTESIAN_POINT('Ctrl Pts',(148.596482723494,-85.722216299478,-35.2526418166199));
#24669=CARTESIAN_POINT('Ctrl Pts',(148.644305530043,-85.5547679896948,-35.27726185663));
#24670=CARTESIAN_POINT('Ctrl Pts',(148.705029122345,-85.3421484546081,-35.3085234529253));
#24671=CARTESIAN_POINT('Ctrl Pts',(148.765481316966,-85.1294146679281,-35.3427818320588));
#24672=CARTESIAN_POINT('Ctrl Pts',(148.825445173693,-84.9173615302769,-35.3802763718155));
#24673=CARTESIAN_POINT('Ctrl Pts',(148.844370664429,-84.8504343859753,-35.3921102097894));
#24674=CARTESIAN_POINT('Ctrl Pts',(148.863247416419,-84.7835753430873,-35.4042666139058));
#24675=CARTESIAN_POINT('Ctrl Pts',(148.882068323814,-84.716810316948,-35.4167536897875));
#24676=CARTESIAN_POINT('Ctrl Pts',(148.922791444534,-84.5723496827033,-35.4437721904313));
#24677=CARTESIAN_POINT('Ctrl Pts',(148.963298334263,-84.4281714850057,-35.472367305025));
#24678=CARTESIAN_POINT('Ctrl Pts',(149.003534667861,-84.2844711674245,-35.5026558877997));
#24679=CARTESIAN_POINT('Ctrl Pts',(149.04618468002,-84.1321506216861,-35.5347614080625));
#24680=CARTESIAN_POINT('Ctrl Pts',(149.088661184879,-83.9798999175319,-35.5688472728399));
#24681=CARTESIAN_POINT('Ctrl Pts',(149.130874866131,-83.8280577824072,-35.6051699481951));
#24682=CARTESIAN_POINT('Ctrl Pts',(149.153428770922,-83.7469316413739,-35.6245764092618));
#24683=CARTESIAN_POINT('Ctrl Pts',(149.175907457703,-83.6659227740306,-35.6446218401457));
#24684=CARTESIAN_POINT('Ctrl Pts',(149.198295786019,-83.5850879910549,-35.6653487919112));
#24685=CARTESIAN_POINT('Ctrl Pts',(149.227912989617,-83.4781527973521,-35.6927681839146));
#24686=CARTESIAN_POINT('Ctrl Pts',(149.257371929547,-83.3715229731208,-35.7213784236265));
#24687=CARTESIAN_POINT('Ctrl Pts',(149.286670239745,-83.2652102217286,-35.7513256085597));
#24688=CARTESIAN_POINT('Ctrl Pts',(149.305367125227,-83.1973661268101,-35.7704365771927));
#24689=CARTESIAN_POINT('Ctrl Pts',(149.323998297626,-83.1296521688589,-35.7900922411323));
#24690=CARTESIAN_POINT('Ctrl Pts',(149.342561050911,-83.0620783213206,-35.8103347154936));
#24691=CARTESIAN_POINT('Ctrl Pts',(149.371267458519,-82.957578607228,-35.8416387311794));
#24692=CARTESIAN_POINT('Ctrl Pts',(149.399774767598,-82.85354358919,-35.8742597573607));
#24693=CARTESIAN_POINT('Ctrl Pts',(149.428061694082,-82.7500633861336,-35.9084779858677));
#24694=CARTESIAN_POINT('Ctrl Pts',(149.454923581066,-82.6517963113699,-35.9409723675915));
#24695=CARTESIAN_POINT('Ctrl Pts',(149.481586763681,-82.5540293874012,-35.9749069410053));
#24696=CARTESIAN_POINT('Ctrl Pts',(149.508023085916,-82.4568752753899,-36.0105521857167));
#24697=CARTESIAN_POINT('Ctrl Pts',(149.512553176897,-82.4402270834549,-36.0166603046963));
#24698=CARTESIAN_POINT('Ctrl Pts',(149.517076580988,-82.423596977919,-36.0228187343151));
#24699=CARTESIAN_POINT('Ctrl Pts',(149.521593124103,-82.4069856432661,-36.0290289363977));
#24700=CARTESIAN_POINT('Ctrl Pts',(149.546047412518,-82.3170455368108,-36.0626533409432));
#24701=CARTESIAN_POINT('Ctrl Pts',(149.570311794243,-82.2276143985182,-36.0978073544201));
#24702=CARTESIAN_POINT('Ctrl Pts',(149.594353719129,-82.1388178247201,-36.1347461416766));
#24703=CARTESIAN_POINT('Ctrl Pts',(149.612438155904,-82.0720246693327,-36.1625316524403));
#24704=CARTESIAN_POINT('Ctrl Pts',(149.630396548314,-82.0055912015778,-36.1913275605318));
#24705=CARTESIAN_POINT('Ctrl Pts',(149.648211128679,-81.9395854582948,-36.221254932904));
#24706=CARTESIAN_POINT('Ctrl Pts',(149.655934224025,-81.9109702095317,-36.2342292463905));
#24707=CARTESIAN_POINT('Ctrl Pts',(149.663637104736,-81.8824099165127,-36.2474379019951));
#24708=CARTESIAN_POINT('Ctrl Pts',(149.67131055004,-81.8539394834481,-36.2608852437837));
#24709=CARTESIAN_POINT('Ctrl Pts',(149.685698655412,-81.800555954318,-36.2860997026037));
#24710=CARTESIAN_POINT('Ctrl Pts',(149.699999360784,-81.7474243598168,-36.3121788856479));
#24711=CARTESIAN_POINT('Ctrl Pts',(149.714175605293,-81.6946906272435,-36.3392201558046));
#24712=CARTESIAN_POINT('Ctrl Pts',(149.727286670728,-81.6459192182899,-36.3642295905834));
#24713=CARTESIAN_POINT('Ctrl Pts',(149.7402913331,-81.5974878782028,-36.3900621045965));
#24714=CARTESIAN_POINT('Ctrl Pts',(149.753148950424,-81.5495528039874,-36.4168048599215));
#24715=CARTESIAN_POINT('Ctrl Pts',(149.762929820709,-81.5130882918453,-36.4371482419277));
#24716=CARTESIAN_POINT('Ctrl Pts',(149.7726254041,-81.4769116545467,-36.4580185544263));
#24717=CARTESIAN_POINT('Ctrl Pts',(149.782212501331,-81.4411109947047,-36.4794579384386));
#24718=CARTESIAN_POINT('Ctrl Pts',(149.792712453297,-81.4019015030661,-36.502938716499));
#24719=CARTESIAN_POINT('Ctrl Pts',(149.80309231573,-81.3631061432707,-36.5271022623885));
#24720=CARTESIAN_POINT('Ctrl Pts',(149.813325028167,-81.3248298095057,-36.5520580116851));
#24721=CARTESIAN_POINT('Ctrl Pts',(149.822817814989,-81.2893212306252,-36.57520921519));
#24722=CARTESIAN_POINT('Ctrl Pts',(149.832167251567,-81.2543175533125,-36.5989995466143));
#24723=CARTESIAN_POINT('Ctrl Pts',(149.841373631762,-81.2198208405048,-36.6235944717091));
#24724=CARTESIAN_POINT('Ctrl Pts',(149.850444720925,-81.1858310691643,-36.6478279656298));
#24725=CARTESIAN_POINT('Ctrl Pts',(149.859377062135,-81.1523329411813,-36.6728423498981));
#24726=CARTESIAN_POINT('Ctrl Pts',(149.868158592941,-81.1193744240766,-36.6988172833898));
#24727=CARTESIAN_POINT('Ctrl Pts',(149.876313696669,-81.0887669899474,-36.7229393051219));
#24728=CARTESIAN_POINT('Ctrl Pts',(149.884338741475,-81.0586248955809,-36.7478897210516));
#24729=CARTESIAN_POINT('Ctrl Pts',(149.892212585395,-81.0290296767013,-36.7738322591383));
#24730=CARTESIAN_POINT('Ctrl Pts',(149.89281740775,-81.0267563461447,-36.7758250122512));
#24731=CARTESIAN_POINT('Ctrl Pts',(149.89342133192,-81.0244862651392,-36.7778236297116));
#24732=CARTESIAN_POINT('Ctrl Pts',(149.894024345238,-81.0222194822742,-36.7798281910486));
#24733=CARTESIAN_POINT('Ctrl Pts',(149.901678691384,-80.9934460867893,-36.805273079051));
#24734=CARTESIAN_POINT('Ctrl Pts',(149.909127380051,-80.9654260581732,-36.8314799870868));
#24735=CARTESIAN_POINT('Ctrl Pts',(149.916327644768,-80.9383234966228,-36.8585857768089));
#24736=CARTESIAN_POINT('Ctrl Pts',(149.922896825409,-80.9135964026002,-36.8833158160625));
#24737=CARTESIAN_POINT('Ctrl Pts',(149.929259164437,-80.8896331987156,-36.9087941212806));
#24738=CARTESIAN_POINT('Ctrl Pts',(149.935369835439,-80.8666055523399,-36.9351356817967));
#24739=CARTESIAN_POINT('Ctrl Pts',(149.935956871689,-80.8643933463218,-36.9376662469162));
#24740=CARTESIAN_POINT('Ctrl Pts',(149.936541575424,-80.8621898122598,-36.9402047878345));
#24741=CARTESIAN_POINT('Ctrl Pts',(149.937123900464,-80.8599951269442,-36.9427514122747));
#24742=CARTESIAN_POINT('Ctrl Pts',(149.949888621083,-80.8118870379003,-36.9985741010473));
#24743=CARTESIAN_POINT('Ctrl Pts',(149.961572072671,-80.7677918263995,-37.0585526832355));
#24744=CARTESIAN_POINT('Ctrl Pts',(149.971367310254,-80.7307169524392,-37.1227154597912));
#24745=CARTESIAN_POINT('Ctrl Pts',(149.975158206732,-80.7163684480826,-37.1475473683212));
#24746=CARTESIAN_POINT('Ctrl Pts',(149.978650998302,-80.7031305919437,-37.1730908787877));
#24747=CARTESIAN_POINT('Ctrl Pts',(149.981796037926,-80.6911891223571,-37.1992286595142));
#24748=CARTESIAN_POINT('Ctrl Pts',(149.985757876154,-80.6761463323226,-37.2321546862971));
#24749=CARTESIAN_POINT('Ctrl Pts',(149.989179977686,-80.6631984113666,-37.2661215533609));
#24750=CARTESIAN_POINT('Ctrl Pts',(149.991954976261,-80.6527310533642,-37.3008958029158));
#24751=CARTESIAN_POINT('Ctrl Pts',(149.993127423005,-80.6483085574699,-37.3155880467322));
#24752=CARTESIAN_POINT('Ctrl Pts',(149.994184300917,-80.6443291875707,-37.33042386883));
#24753=CARTESIAN_POINT('Ctrl Pts',(149.995117265699,-80.6408234431072,-37.3453832597703));
#24754=CARTESIAN_POINT('Ctrl Pts',(149.997168971269,-80.633113875098,-37.3782808206258));
#24755=CARTESIAN_POINT('Ctrl Pts',(149.998622294846,-80.6276965661506,-37.4117792041177));
#24756=CARTESIAN_POINT('Ctrl Pts',(149.999384955835,-80.6248606269893,-37.4456825897633));
#24757=CARTESIAN_POINT('Ctrl Pts',(149.999789923498,-80.6233547630873,-37.4636850509217));
#24758=CARTESIAN_POINT('Ctrl Pts',(150.,-80.6225774829854,-37.4818014034218));
#24759=CARTESIAN_POINT('Ctrl Pts',(150.,-80.6225774829854,-37.5));
#24760=CARTESIAN_POINT('Origin',(152.5,-122.5,85.));
#24761=CARTESIAN_POINT('Origin',(152.5,-122.5,-37.5));
#24762=CARTESIAN_POINT('Origin',(0.,-122.5,49.5));
#24763=CARTESIAN_POINT('Origin',(121.449578014911,-122.5,49.5));
#24764=CARTESIAN_POINT('Origin',(147.5,-122.5,49.5));
#24765=CARTESIAN_POINT('Ctrl Pts',(145.36231884058,-88.1464478086873,-32.5));
#24766=CARTESIAN_POINT('Ctrl Pts',(145.36231884058,-88.1464478086873,-35.));
#24767=CARTESIAN_POINT('Ctrl Pts',(147.5,-89.4427190999916,-35.));
#24768=CARTESIAN_POINT('Ctrl Pts',(145.883280419022,-87.287330000178,-32.5000000009303));
#24769=CARTESIAN_POINT('Ctrl Pts',(145.793011707107,-87.4361921450692,-34.7836438007554));
#24770=CARTESIAN_POINT('Ctrl Pts',(147.764311380885,-88.5709672327977,-35.));
#24771=CARTESIAN_POINT('Ctrl Pts',(146.390924783416,-86.4329953777441,-32.5817470282946));
#24772=CARTESIAN_POINT('Ctrl Pts',(146.256366271119,-86.6602829701324,-34.6533815799968));
#24773=CARTESIAN_POINT('Ctrl Pts',(148.021866250328,-87.7040688391623,-35.0408735143647));
#24774=CARTESIAN_POINT('Ctrl Pts',(147.132955592072,-85.159466684389,-32.8264997589554));
#24775=CARTESIAN_POINT('Ctrl Pts',(146.95625485105,-85.4644664729262,-34.6060350541333));
#24776=CARTESIAN_POINT('Ctrl Pts',(148.398337763665,-86.4118117826985,-35.163249879369));
#24777=CARTESIAN_POINT('Ctrl Pts',(147.377049426154,-84.7363019818542,-32.9287776457782));
#24778=CARTESIAN_POINT('Ctrl Pts',(147.185340564392,-85.0695699101127,-34.6128471107274));
#24779=CARTESIAN_POINT('Ctrl Pts',(148.522179488132,-85.9824240698147,-35.2143888231312));
#24780=CARTESIAN_POINT('Ctrl Pts',(147.858493843555,-83.8933928830767,-33.1802802395072));
#24781=CARTESIAN_POINT('Ctrl Pts',(147.640340054158,-84.2776371924664,-34.6763398436954));
#24782=CARTESIAN_POINT('Ctrl Pts',(148.766441729588,-85.1271192490123,-35.3401401195115));
#24783=CARTESIAN_POINT('Ctrl Pts',(148.095887496715,-83.473525962111,-33.3296903827866));
#24784=CARTESIAN_POINT('Ctrl Pts',(147.866955151253,-83.8795640251386,-34.7317798844392));
#24785=CARTESIAN_POINT('Ctrl Pts',(148.886884097339,-84.701077814479,-35.4148451917191));
#24786=CARTESIAN_POINT('Ctrl Pts',(148.555727425866,-82.6523882229576,-33.6809331684121));
#24787=CARTESIAN_POINT('Ctrl Pts',(148.307824862021,-83.0977615436452,-34.8965208417471));
#24788=CARTESIAN_POINT('Ctrl Pts',(149.120185238382,-83.86786452037,-35.5904665838802));
#24789=CARTESIAN_POINT('Ctrl Pts',(148.780093861297,-82.2476812683578,-33.8839399244688));
#24790=CARTESIAN_POINT('Ctrl Pts',(148.52472777307,-82.7095240936269,-35.0050364952419));
#24791=CARTESIAN_POINT('Ctrl Pts',(149.234018208523,-83.4572059928576,-35.69196996268));
#24792=CARTESIAN_POINT('Ctrl Pts',(149.207972890121,-81.4688789012016,-34.3573989375057));
#24793=CARTESIAN_POINT('Ctrl Pts',(148.939317285436,-81.9607628458189,-35.2860875789416));
#24794=CARTESIAN_POINT('Ctrl Pts',(149.451103893298,-82.6669506497836,-35.9286994683073));
#24795=CARTESIAN_POINT('Ctrl Pts',(149.410469407752,-81.0966396786722,-34.6254381321728));
#24796=CARTESIAN_POINT('Ctrl Pts',(149.13707735126,-81.6002642788733,-35.4559386647908));
#24797=CARTESIAN_POINT('Ctrl Pts',(149.553841095111,-82.2892373209608,-36.0627190669335));
#24798=CARTESIAN_POINT('Ctrl Pts',(149.689478100498,-80.5797647052594,-35.1010485304976));
#24799=CARTESIAN_POINT('Ctrl Pts',(149.410828634125,-81.0973762069276,-35.7764659917703));
#24800=CARTESIAN_POINT('Ctrl Pts',(149.695396978193,-81.7647612450649,-36.3005242648253));
#24801=CARTESIAN_POINT('Ctrl Pts',(149.778860900692,-80.4134491496523,-35.2734504935361));
#24802=CARTESIAN_POINT('Ctrl Pts',(149.498351131334,-80.9359152801443,-35.8944893614086));
#24803=CARTESIAN_POINT('Ctrl Pts',(149.740745603139,-81.595999872402,-36.3867252471501));
#24804=CARTESIAN_POINT('Ctrl Pts',(149.942345818683,-80.1081950067719,-35.6444293836609));
#24805=CARTESIAN_POINT('Ctrl Pts',(149.65844369221,-80.6395711160561,-36.153254701076));
#24806=CARTESIAN_POINT('Ctrl Pts',(149.823690158897,-81.2862566980873,-36.5722146914484));
#24807=CARTESIAN_POINT('Ctrl Pts',(150.016754772459,-79.9686937648418,-35.8430315532085));
#24808=CARTESIAN_POINT('Ctrl Pts',(149.731542660712,-80.5037270542566,-36.2939840338164));
#24809=CARTESIAN_POINT('Ctrl Pts',(149.861441758745,-81.144703967216,-36.6715157768338));
#24810=CARTESIAN_POINT('Ctrl Pts',(150.145196691125,-79.7272764209246,-36.2762826327136));
#24811=CARTESIAN_POINT('Ctrl Pts',(149.857607243134,-80.2688649285009,-36.6048325581329));
#24812=CARTESIAN_POINT('Ctrl Pts',(149.926607145573,-80.8997363683411,-36.8881413161273));
#24813=CARTESIAN_POINT('Ctrl Pts',(150.197080555724,-79.6294105444985,-36.5038809199123));
#24814=CARTESIAN_POINT('Ctrl Pts',(149.908727602392,-80.1732994372084,-36.7701162187303));
#24815=CARTESIAN_POINT('Ctrl Pts',(149.952930574586,-80.8004312877628,-37.0019404601773));
#24816=CARTESIAN_POINT('Ctrl Pts',(150.269771338359,-79.4921496315481,-36.9870649844503));
#24817=CARTESIAN_POINT('Ctrl Pts',(149.980179574577,-80.0395829024242,-37.1229099719677));
#24818=CARTESIAN_POINT('Ctrl Pts',(149.989810459912,-80.6611518320492,-37.243532492004));
#24819=CARTESIAN_POINT('Ctrl Pts',(150.289855071895,-79.4541343321333,-37.2465705504854));
#24820=CARTESIAN_POINT('Ctrl Pts',(149.99999999943,-80.0024038110911,-37.313811727788));
#24821=CARTESIAN_POINT('Ctrl Pts',(150.,-80.6225774840775,-37.3732852754135));
#24822=CARTESIAN_POINT('Ctrl Pts',(150.289855072464,-79.4541343310581,-37.5));
#24823=CARTESIAN_POINT('Ctrl Pts',(150.,-80.0024038100394,-37.5));
#24824=CARTESIAN_POINT('Ctrl Pts',(150.,-80.6225774829855,-37.5));
#24825=CARTESIAN_POINT('Origin',(147.5,-89.4427190999916,-32.5));
#24826=CARTESIAN_POINT('Origin',(147.5,-122.5,-37.5));
#24827=CARTESIAN_POINT('Origin',(147.5,-122.5,-32.5));
#24828=CARTESIAN_POINT('Origin',(147.5,-122.5,44.5));
#24829=CARTESIAN_POINT('Origin',(152.5,-122.5,44.5));
#24830=CARTESIAN_POINT('Origin',(147.5,-122.5,44.5));
#24831=CARTESIAN_POINT('Origin',(121.449578014911,-122.5,49.5));
#24832=CARTESIAN_POINT('Origin',(121.449578014911,-122.5,49.5));
#24833=CARTESIAN_POINT('Origin',(0.,0.,-32.5));
#24834=CARTESIAN_POINT('Origin',(121.449578014911,-122.5,-32.5));
#24835=CARTESIAN_POINT('Origin',(0.,-122.5,-32.5));
#24836=CARTESIAN_POINT('Origin',(121.449578014911,-122.5,-32.5));
#24837=CARTESIAN_POINT('Origin',(152.5,-122.5,47.));
#24838=CARTESIAN_POINT('Origin',(152.5,-122.5,37.5));
#24839=CARTESIAN_POINT('Origin',(147.5,-79.9999999999999,44.5));
#24840=CARTESIAN_POINT('Ctrl Pts',(147.5,-89.4427190999916,47.));
#24841=CARTESIAN_POINT('Ctrl Pts',(147.692029124167,-88.8093685912607,47.));
#24842=CARTESIAN_POINT('Ctrl Pts',(147.881019325447,-88.1768396525117,46.9784293604652));
#24843=CARTESIAN_POINT('Ctrl Pts',(148.067032921855,-87.5451886197927,46.9349710385975));
#24844=CARTESIAN_POINT('Ctrl Pts',(148.113199638035,-87.3884191442505,46.9241851172987));
#24845=CARTESIAN_POINT('Ctrl Pts',(148.159182993745,-87.2317038217232,46.9120507147773));
#24846=CARTESIAN_POINT('Ctrl Pts',(148.204983936061,-87.075043664733,46.8985625026983));
#24847=CARTESIAN_POINT('Ctrl Pts',(148.227650188964,-86.9975147197269,46.8918873730891));
#24848=CARTESIAN_POINT('Ctrl Pts',(148.250265804087,-86.9200215223737,46.8848824575639));
#24849=CARTESIAN_POINT('Ctrl Pts',(148.272833473781,-86.8425552539348,46.877546723474));
#24850=CARTESIAN_POINT('Ctrl Pts',(148.349179005414,-86.5804899398113,46.8527302259542));
#24851=CARTESIAN_POINT('Ctrl Pts',(148.42497434185,-86.3187382386177,46.8240687356948));
#24852=CARTESIAN_POINT('Ctrl Pts',(148.500300623518,-86.0570314559301,46.7911753910845));
#24853=CARTESIAN_POINT('Ctrl Pts',(148.548487711945,-85.8896146181409,46.7701331403549));
#24854=CARTESIAN_POINT('Ctrl Pts',(148.596482723484,-85.7222162995132,46.7473581833852));
#24855=CARTESIAN_POINT('Ctrl Pts',(148.644305530043,-85.5547679896948,46.7227381433699));
#24856=CARTESIAN_POINT('Ctrl Pts',(148.705029122316,-85.3421484547092,46.6914765470896));
#24857=CARTESIAN_POINT('Ctrl Pts',(148.765481316907,-85.1294146681287,46.6572181679748));
#24858=CARTESIAN_POINT('Ctrl Pts',(148.825445173605,-84.9173615305767,46.6197236282395));
#24859=CARTESIAN_POINT('Ctrl Pts',(148.844370664369,-84.8504343861742,46.6078897902489));
#24860=CARTESIAN_POINT('Ctrl Pts',(148.863247416388,-84.7835753431854,46.5957333861149));
#24861=CARTESIAN_POINT('Ctrl Pts',(148.882068323811,-84.7168103169457,46.5832463102145));
#24862=CARTESIAN_POINT('Ctrl Pts',(148.922791444531,-84.5723496827009,46.5562278095707));
#24863=CARTESIAN_POINT('Ctrl Pts',(148.963298334261,-84.4281714850036,46.5276326949765));
#24864=CARTESIAN_POINT('Ctrl Pts',(149.003534667861,-84.2844711674245,46.4973441122003));
#24865=CARTESIAN_POINT('Ctrl Pts',(149.04618468001,-84.1321506217299,46.4652385919447));
#24866=CARTESIAN_POINT('Ctrl Pts',(149.088661184858,-83.9798999176171,46.431152727177));
#24867=CARTESIAN_POINT('Ctrl Pts',(149.130874866099,-83.8280577825329,46.3948300518332));
#24868=CARTESIAN_POINT('Ctrl Pts',(149.153428770871,-83.7469316415657,46.3754235907832));
#24869=CARTESIAN_POINT('Ctrl Pts',(149.175907457634,-83.6659227742882,46.3553781599173));
#24870=CARTESIAN_POINT('Ctrl Pts',(149.198295785931,-83.5850879913779,46.3346512081709));
#24871=CARTESIAN_POINT('Ctrl Pts',(149.227912989408,-83.4781527981097,46.3072318162821));
#24872=CARTESIAN_POINT('Ctrl Pts',(149.257371929218,-83.3715229743104,46.2786215766946));
#24873=CARTESIAN_POINT('Ctrl Pts',(149.286670239298,-83.265210223348,46.2486743918971));
#24874=CARTESIAN_POINT('Ctrl Pts',(149.30536712493,-83.1973661278873,46.2295634231207));
#24875=CARTESIAN_POINT('Ctrl Pts',(149.323998297478,-83.1296521693962,46.2099077590292));
#24876=CARTESIAN_POINT('Ctrl Pts',(149.342561050911,-83.0620783213206,46.1896652845064));
#24877=CARTESIAN_POINT('Ctrl Pts',(149.371267458519,-82.95757860723,46.1583612688204));
#24878=CARTESIAN_POINT('Ctrl Pts',(149.399774767598,-82.8535435891935,46.1257402426392));
#24879=CARTESIAN_POINT('Ctrl Pts',(149.428061694081,-82.7500633861384,46.0915220141326));
#24880=CARTESIAN_POINT('Ctrl Pts',(149.454923581065,-82.6517963113774,46.0590276324095));
#24881=CARTESIAN_POINT('Ctrl Pts',(149.48158676368,-82.5540293874111,46.0250930589968));
#24882=CARTESIAN_POINT('Ctrl Pts',(149.508023085913,-82.4568752754022,45.9894478142867));
#24883=CARTESIAN_POINT('Ctrl Pts',(149.512553176896,-82.4402270834634,45.9833396953057));
#24884=CARTESIAN_POINT('Ctrl Pts',(149.517076580988,-82.4235969779237,45.9771812656855));
#24885=CARTESIAN_POINT('Ctrl Pts',(149.521593124104,-82.406985643267,45.9709710636017));
#24886=CARTESIAN_POINT('Ctrl Pts',(149.546047412515,-82.3170455368253,45.9373466590614));
#24887=CARTESIAN_POINT('Ctrl Pts',(149.570311794236,-82.2276143985462,45.9021926455905));
#24888=CARTESIAN_POINT('Ctrl Pts',(149.594353719118,-82.1388178247614,45.8652538583403));
#24889=CARTESIAN_POINT('Ctrl Pts',(149.612438155897,-82.07202466936,45.8374683475715));
#24890=CARTESIAN_POINT('Ctrl Pts',(149.63039654831,-82.0055912015912,45.8086724394745));
#24891=CARTESIAN_POINT('Ctrl Pts',(149.648211128679,-81.9395854582945,45.7787450670962));
#24892=CARTESIAN_POINT('Ctrl Pts',(149.655934224025,-81.9109702095313,45.7657707536098));
#24893=CARTESIAN_POINT('Ctrl Pts',(149.663637104736,-81.8824099165123,45.7525620980052));
#24894=CARTESIAN_POINT('Ctrl Pts',(149.67131055004,-81.8539394834478,45.7391147562166));
#24895=CARTESIAN_POINT('Ctrl Pts',(149.685698655415,-81.8005559543078,45.7139002973917));
#24896=CARTESIAN_POINT('Ctrl Pts',(149.699999360789,-81.7474243597972,45.6878211143421));
#24897=CARTESIAN_POINT('Ctrl Pts',(149.714175605301,-81.6946906272146,45.6607798441796));
#24898=CARTESIAN_POINT('Ctrl Pts',(149.727286670739,-81.6459192182512,45.6357704093948));
#24899=CARTESIAN_POINT('Ctrl Pts',(149.740291333114,-81.5974878781543,45.6099378953754));
#24900=CARTESIAN_POINT('Ctrl Pts',(149.75314895044,-81.549552803929,45.583195140044));
#24901=CARTESIAN_POINT('Ctrl Pts',(149.76292982072,-81.5130882918071,45.5628517580484));
#24902=CARTESIAN_POINT('Ctrl Pts',(149.772625404106,-81.4769116545282,45.5419814455611));
#24903=CARTESIAN_POINT('Ctrl Pts',(149.782212501331,-81.4411109947051,45.5205420615612));
#24904=CARTESIAN_POINT('Ctrl Pts',(149.792712453297,-81.4019015030656,45.4970612835013));
#24905=CARTESIAN_POINT('Ctrl Pts',(149.80309231573,-81.3631061432697,45.4728977376122));
#24906=CARTESIAN_POINT('Ctrl Pts',(149.813325028167,-81.3248298095044,45.4479419883158));
#24907=CARTESIAN_POINT('Ctrl Pts',(149.822817814989,-81.2893212306204,45.4247907848088));
#24908=CARTESIAN_POINT('Ctrl Pts',(149.832167251568,-81.2543175533045,45.4010004533823));
#24909=CARTESIAN_POINT('Ctrl Pts',(149.841373631764,-81.2198208404939,45.3764055282848));
#24910=CARTESIAN_POINT('Ctrl Pts',(149.850444720927,-81.1858310691553,45.352172034365));
#24911=CARTESIAN_POINT('Ctrl Pts',(149.859377062136,-81.1523329411743,45.3271576500975));
#24912=CARTESIAN_POINT('Ctrl Pts',(149.868158592942,-81.1193744240714,45.3011827166068));
#24913=CARTESIAN_POINT('Ctrl Pts',(149.876313696672,-81.0887669899374,45.2770606948705));
#24914=CARTESIAN_POINT('Ctrl Pts',(149.884338741479,-81.0586248955663,45.2521102789363));
#24915=CARTESIAN_POINT('Ctrl Pts',(149.8922125854,-81.0290296766821,45.2261677408448));
#24916=CARTESIAN_POINT('Ctrl Pts',(149.892817407753,-81.0267563461319,45.2241749877375));
#24917=CARTESIAN_POINT('Ctrl Pts',(149.893421331922,-81.0244862651328,45.2221763702828));
#24918=CARTESIAN_POINT('Ctrl Pts',(149.894024345238,-81.0222194822742,45.2201718089514));
#24919=CARTESIAN_POINT('Ctrl Pts',(149.901678691384,-80.9934460867894,45.194726920949));
#24920=CARTESIAN_POINT('Ctrl Pts',(149.909127380051,-80.9654260581732,45.1685200129132));
#24921=CARTESIAN_POINT('Ctrl Pts',(149.916327644768,-80.9383234966228,45.1414142231911));
#24922=CARTESIAN_POINT('Ctrl Pts',(149.922896825408,-80.9135964026004,45.1166841839377));
#24923=CARTESIAN_POINT('Ctrl Pts',(149.929259164437,-80.8896331987158,45.0912058787197));
#24924=CARTESIAN_POINT('Ctrl Pts',(149.935369835439,-80.8666055523403,45.0648643182037));
#24925=CARTESIAN_POINT('Ctrl Pts',(149.935956871689,-80.864393346322,45.0623337530841));
#24926=CARTESIAN_POINT('Ctrl Pts',(149.936541575424,-80.8621898122599,45.0597952121657));
#24927=CARTESIAN_POINT('Ctrl Pts',(149.937123900464,-80.8599951269442,45.0572485877254));
#24928=CARTESIAN_POINT('Ctrl Pts',(149.949888621083,-80.8118870379003,45.0014258989527));
#24929=CARTESIAN_POINT('Ctrl Pts',(149.961572072671,-80.7677918263995,44.9414473167645));
#24930=CARTESIAN_POINT('Ctrl Pts',(149.971367310254,-80.7307169524392,44.8772845402088));
#24931=CARTESIAN_POINT('Ctrl Pts',(149.975158206732,-80.7163684480826,44.8524526316788));
#24932=CARTESIAN_POINT('Ctrl Pts',(149.978650998302,-80.7031305919437,44.8269091212123));
#24933=CARTESIAN_POINT('Ctrl Pts',(149.981796037926,-80.6911891223571,44.8007713404859));
#24934=CARTESIAN_POINT('Ctrl Pts',(149.985757876155,-80.6761463323222,44.767845313702));
#24935=CARTESIAN_POINT('Ctrl Pts',(149.989179977686,-80.6631984113658,44.7338784466372));
#24936=CARTESIAN_POINT('Ctrl Pts',(149.991954976262,-80.6527310533633,44.6991041970813));
#24937=CARTESIAN_POINT('Ctrl Pts',(149.993127423005,-80.6483085574693,44.6844119532658));
#24938=CARTESIAN_POINT('Ctrl Pts',(149.994184300917,-80.6443291875704,44.669576131169));
#24939=CARTESIAN_POINT('Ctrl Pts',(149.995117265699,-80.6408234431072,44.6546167402297));
#24940=CARTESIAN_POINT('Ctrl Pts',(149.997168971269,-80.6331138750976,44.6217191793725));
#24941=CARTESIAN_POINT('Ctrl Pts',(149.998622294847,-80.62769656615,44.5882207958789));
#24942=CARTESIAN_POINT('Ctrl Pts',(149.999384955835,-80.6248606269888,44.5543174102316));
#24943=CARTESIAN_POINT('Ctrl Pts',(149.999789923498,-80.6233547630872,44.5363149490749));
#24944=CARTESIAN_POINT('Ctrl Pts',(150.,-80.6225774829854,44.5181985965764));
#24945=CARTESIAN_POINT('Ctrl Pts',(150.,-80.6225774829854,44.5));
#24946=CARTESIAN_POINT('Origin',(0.,0.,49.5));
#24947=CARTESIAN_POINT('Origin',(147.5,-89.4427190999916,49.5));
#24948=CARTESIAN_POINT('Origin',(121.449578014911,-122.5,-32.5));
#24949=CARTESIAN_POINT('Origin',(147.5,-122.5,37.5));
#24950=CARTESIAN_POINT('Origin',(147.5,-122.5,32.5));
#24951=CARTESIAN_POINT('Origin',(147.5,-122.5,37.5));
#24952=CARTESIAN_POINT('Ctrl Pts',(145.36231884058,-88.1464478086873,49.5));
#24953=CARTESIAN_POINT('Ctrl Pts',(145.36231884058,-88.1464478086873,47.));
#24954=CARTESIAN_POINT('Ctrl Pts',(147.5,-89.4427190999916,47.));
#24955=CARTESIAN_POINT('Ctrl Pts',(145.88328041902,-87.2873300001825,49.4999999990697));
#24956=CARTESIAN_POINT('Ctrl Pts',(145.793011707092,-87.4361921450511,47.2163561992337));
#24957=CARTESIAN_POINT('Ctrl Pts',(147.764311380887,-88.5709672327986,47.));
#24958=CARTESIAN_POINT('Ctrl Pts',(146.390924783419,-86.432995377738,49.4182529717019));
#24959=CARTESIAN_POINT('Ctrl Pts',(146.25636627112,-86.6602829701382,47.3466184200069));
#24960=CARTESIAN_POINT('Ctrl Pts',(148.021866250329,-87.7040688391623,46.959126485635));
#24961=CARTESIAN_POINT('Ctrl Pts',(147.13295559207,-85.1594666843921,49.1735002410464));
#24962=CARTESIAN_POINT('Ctrl Pts',(146.95625485105,-85.4644664729224,47.393964945865));
#24963=CARTESIAN_POINT('Ctrl Pts',(148.398337763665,-86.4118117826985,46.8367501206312));
#24964=CARTESIAN_POINT('Ctrl Pts',(147.377049426154,-84.7363019818542,49.0712223542218));
#24965=CARTESIAN_POINT('Ctrl Pts',(147.185340564392,-85.0695699101127,47.3871528892726));
#24966=CARTESIAN_POINT('Ctrl Pts',(148.522179488132,-85.9824240698147,46.7856111768689));
#24967=CARTESIAN_POINT('Ctrl Pts',(147.858493843555,-83.8933928830767,48.8197197604928));
#24968=CARTESIAN_POINT('Ctrl Pts',(147.640340054158,-84.2776371924664,47.3236601563046));
#24969=CARTESIAN_POINT('Ctrl Pts',(148.766441729588,-85.1271192490123,46.6598598804885));
#24970=CARTESIAN_POINT('Ctrl Pts',(148.095887496716,-83.4735259621086,48.670309617217));
#24971=CARTESIAN_POINT('Ctrl Pts',(147.866955151253,-83.8795640251351,47.2682201155608));
#24972=CARTESIAN_POINT('Ctrl Pts',(148.886884097334,-84.7010778144719,46.5851548082849));
#24973=CARTESIAN_POINT('Ctrl Pts',(148.555727425865,-82.65238822296,48.3190668315844));
#24974=CARTESIAN_POINT('Ctrl Pts',(148.307824862021,-83.0977615436487,47.1034791582529));
#24975=CARTESIAN_POINT('Ctrl Pts',(149.120185238387,-83.867864520377,46.4095334161157));
#24976=CARTESIAN_POINT('Ctrl Pts',(148.780093861296,-82.2476812683581,48.1160600755383));
#24977=CARTESIAN_POINT('Ctrl Pts',(148.524727773055,-82.7095240936236,46.9949635047617));
#24978=CARTESIAN_POINT('Ctrl Pts',(149.234018208522,-83.457205992854,46.308030037322));
#24979=CARTESIAN_POINT('Ctrl Pts',(149.207972890121,-81.4688789012013,47.6426010624872));
#24980=CARTESIAN_POINT('Ctrl Pts',(148.93931728545,-81.9607628458225,46.713912421055));
#24981=CARTESIAN_POINT('Ctrl Pts',(149.4511038933,-82.6669506497871,46.0713005316908));
#24982=CARTESIAN_POINT('Ctrl Pts',(149.410469407752,-81.0966396786721,47.3745618678272));
#24983=CARTESIAN_POINT('Ctrl Pts',(149.13707735126,-81.6002642788733,46.5440613352092));
#24984=CARTESIAN_POINT('Ctrl Pts',(149.553841095111,-82.2892373209608,45.9372809330665));
#24985=CARTESIAN_POINT('Ctrl Pts',(149.689478100498,-80.5797647052593,46.8989514695024));
#24986=CARTESIAN_POINT('Ctrl Pts',(149.410828634125,-81.0973762069276,46.2235340082297));
#24987=CARTESIAN_POINT('Ctrl Pts',(149.695396978193,-81.7647612450649,45.6994757351747));
#24988=CARTESIAN_POINT('Ctrl Pts',(149.778860900691,-80.4134491496535,46.7265495064604));
#24989=CARTESIAN_POINT('Ctrl Pts',(149.498351131341,-80.935915280146,46.1055106385897));
#24990=CARTESIAN_POINT('Ctrl Pts',(149.74074560314,-81.5959998724055,45.6132747528471));
#24991=CARTESIAN_POINT('Ctrl Pts',(149.942345818684,-80.1081950067706,46.3555706163427));
#24992=CARTESIAN_POINT('Ctrl Pts',(149.658443692203,-80.6395711160542,45.8467452989258));
#24993=CARTESIAN_POINT('Ctrl Pts',(149.823690158896,-81.2862566980837,45.4277853085544));
#24994=CARTESIAN_POINT('Ctrl Pts',(150.016754772459,-79.9686937648418,46.1569684467915));
#24995=CARTESIAN_POINT('Ctrl Pts',(149.731542660712,-80.5037270542566,45.7060159661836));
#24996=CARTESIAN_POINT('Ctrl Pts',(149.861441758745,-81.144703967216,45.3284842231662));
#24997=CARTESIAN_POINT('Ctrl Pts',(150.145196691125,-79.7272764209246,45.7237173672864));
#24998=CARTESIAN_POINT('Ctrl Pts',(149.857607243134,-80.2688649285009,45.3951674418671));
#24999=CARTESIAN_POINT('Ctrl Pts',(149.926607145573,-80.8997363683411,45.1118586838727));
#25000=CARTESIAN_POINT('Ctrl Pts',(150.197080555724,-79.6294105444985,45.4961190800877));
#25001=CARTESIAN_POINT('Ctrl Pts',(149.908727602392,-80.1732994372084,45.2298837812697));
#25002=CARTESIAN_POINT('Ctrl Pts',(149.952930574586,-80.8004312877628,44.9980595398227));
#25003=CARTESIAN_POINT('Ctrl Pts',(150.269771338359,-79.4921496315481,45.0129350155497));
#25004=CARTESIAN_POINT('Ctrl Pts',(149.980179574577,-80.0395829024242,44.8770900280323));
#25005=CARTESIAN_POINT('Ctrl Pts',(149.989810459912,-80.6611518320492,44.756467507996));
#25006=CARTESIAN_POINT('Ctrl Pts',(150.289855071895,-79.4541343321333,44.7534294495147));
#25007=CARTESIAN_POINT('Ctrl Pts',(149.99999999943,-80.0024038110911,44.686188272212));
#25008=CARTESIAN_POINT('Ctrl Pts',(150.,-80.6225774840775,44.6267147245865));
#25009=CARTESIAN_POINT('Ctrl Pts',(150.289855072464,-79.4541343310581,44.5));
#25010=CARTESIAN_POINT('Ctrl Pts',(150.,-80.0024038100394,44.5));
#25011=CARTESIAN_POINT('Ctrl Pts',(150.,-80.6225774829855,44.5));
#25012=CARTESIAN_POINT('Origin',(152.5,-80.6225774829854,44.5));
#25013=CARTESIAN_POINT('Origin',(115.217186218029,-122.5,32.5));
#25014=CARTESIAN_POINT('Origin',(121.449578014911,-122.5,32.5));
#25015=CARTESIAN_POINT('Origin',(147.5,0.,37.5));
#25016=CARTESIAN_POINT('Ctrl Pts',(150.,-80.6225774829854,37.5));
#25017=CARTESIAN_POINT('Ctrl Pts',(150.,-80.6225774829854,37.4687656111694));
#25018=CARTESIAN_POINT('Ctrl Pts',(149.999418286665,-80.6247797743348,37.4378789835208));
#25019=CARTESIAN_POINT('Ctrl Pts',(149.998293554945,-80.6290354954266,37.407427664437));
#25020=CARTESIAN_POINT('Ctrl Pts',(149.997125538082,-80.6334549973543,37.3758044305616));
#25021=CARTESIAN_POINT('Ctrl Pts',(149.995371936956,-80.6400888791783,37.3446506435412));
#25022=CARTESIAN_POINT('Ctrl Pts',(149.993090530187,-80.6487160556982,37.3140587875661));
#25023=CARTESIAN_POINT('Ctrl Pts',(149.992231155702,-80.6519657941863,37.3025352570628));
#25024=CARTESIAN_POINT('Ctrl Pts',(149.991297028852,-80.6554978429528,37.2910914065902));
#25025=CARTESIAN_POINT('Ctrl Pts',(149.990291719683,-80.6592985775913,37.2797319931106));
#25026=CARTESIAN_POINT('Ctrl Pts',(149.987499102739,-80.6698565196466,37.2481770331612));
#25027=CARTESIAN_POINT('Ctrl Pts',(149.984157100677,-80.6824881297729,37.2172858271412));
#25028=CARTESIAN_POINT('Ctrl Pts',(149.980355786964,-80.6968505802923,37.1871743733059));
#25029=CARTESIAN_POINT('Ctrl Pts',(149.977558137322,-80.7074209008703,37.1650132720595));
#25030=CARTESIAN_POINT('Ctrl Pts',(149.974509955706,-80.7189351701335,37.1432550493073));
#25031=CARTESIAN_POINT('Ctrl Pts',(149.971243495187,-80.7312708109914,37.1219053194033));
#25032=CARTESIAN_POINT('Ctrl Pts',(149.965898079908,-80.7514575307577,37.0869674495657));
#25033=CARTESIAN_POINT('Ctrl Pts',(149.960009186179,-80.7736866486408,37.0534295032289));
#25034=CARTESIAN_POINT('Ctrl Pts',(149.953740444404,-80.7973352935607,37.0212984264036));
#25035=CARTESIAN_POINT('Ctrl Pts',(149.948225014278,-80.8181420923229,36.9930285254523));
#25036=CARTESIAN_POINT('Ctrl Pts',(149.9424154207,-80.8400482470993,36.9658474797256));
#25037=CARTESIAN_POINT('Ctrl Pts',(149.936415096464,-80.8626613647233,36.9397533647229));
#25038=CARTESIAN_POINT('Ctrl Pts',(149.930229230798,-80.8859737229196,36.9128523700934));
#25039=CARTESIAN_POINT('Ctrl Pts',(149.923781601043,-80.9102578633714,36.8868469814882));
#25040=CARTESIAN_POINT('Ctrl Pts',(149.917129634266,-80.9352949903542,36.8616578829462));
#25041=CARTESIAN_POINT('Ctrl Pts',(149.910169623638,-80.9614915538297,36.8353023103081));
#25042=CARTESIAN_POINT('Ctrl Pts',(149.902985851619,-80.9885126935505,36.8098403335412));
#25043=CARTESIAN_POINT('Ctrl Pts',(149.895629953764,-81.0161619977715,36.7851874043794));
#25044=CARTESIAN_POINT('Ctrl Pts',(149.894768894784,-81.0193985410377,36.7823016076435));
#25045=CARTESIAN_POINT('Ctrl Pts',(149.893905462669,-81.0226437475978,36.7794269040118));
#25046=CARTESIAN_POINT('Ctrl Pts',(149.893039728921,-81.0258973457795,36.7765631636536));
#25047=CARTESIAN_POINT('Ctrl Pts',(149.885294621979,-81.055004985282,36.7509433060931));
#25048=CARTESIAN_POINT('Ctrl Pts',(149.877335285324,-81.0848961910412,36.7261125791076));
#25049=CARTESIAN_POINT('Ctrl Pts',(149.869211724912,-81.1153826082176,36.7020057412078));
#25050=CARTESIAN_POINT('Ctrl Pts',(149.860756318493,-81.1471143901479,36.6769141432401));
#25051=CARTESIAN_POINT('Ctrl Pts',(149.852122887,-81.1794914280943,36.6526066770636));
#25052=CARTESIAN_POINT('Ctrl Pts',(149.843353240441,-81.2123567795935,36.6290138576965));
#25053=CARTESIAN_POINT('Ctrl Pts',(149.834033859779,-81.2472823286659,36.6039420987476));
#25054=CARTESIAN_POINT('Ctrl Pts',(149.824560562659,-81.2827596737919,36.5796772330571));
#25055=CARTESIAN_POINT('Ctrl Pts',(149.814968902639,-81.3186560159925,36.5561425173913));
#25056=CARTESIAN_POINT('Ctrl Pts',(149.814245534137,-81.3213631890216,36.5543676137774));
#25057=CARTESIAN_POINT('Ctrl Pts',(149.813521486337,-81.3240727682653,36.5525968666255));
#25058=CARTESIAN_POINT('Ctrl Pts',(149.81279677161,-81.3267847076918,36.5508302448381));
#25059=CARTESIAN_POINT('Ctrl Pts',(149.802161746897,-81.3665818053887,36.524905469683));
#25060=CARTESIAN_POINT('Ctrl Pts',(149.791378236575,-81.4068954418303,36.4998550500825));
#25061=CARTESIAN_POINT('Ctrl Pts',(149.780505488345,-81.4474999785173,36.4756491236568));
#25062=CARTESIAN_POINT('Ctrl Pts',(149.766212096436,-81.5008789903217,36.4438278411639));
#25063=CARTESIAN_POINT('Ctrl Pts',(149.75173104415,-81.5548874755345,36.4133414348087));
#25064=CARTESIAN_POINT('Ctrl Pts',(149.7370901728,-81.6094178533075,36.383984521067));
#25065=CARTESIAN_POINT('Ctrl Pts',(149.721679195218,-81.6668165155372,36.3530834408842));
#25066=CARTESIAN_POINT('Ctrl Pts',(149.706091100881,-81.7247936014325,36.3234339148145));
#25067=CARTESIAN_POINT('Ctrl Pts',(149.690345642872,-81.7832715016969,36.2948268672563));
#25068=CARTESIAN_POINT('Ctrl Pts',(149.684002656687,-81.8068290579968,36.283302648186));
#25069=CARTESIAN_POINT('Ctrl Pts',(149.67763399788,-81.8304683944409,36.2719479292514));
#25070=CARTESIAN_POINT('Ctrl Pts',(149.671240444102,-81.854186356593,36.2607502650745));
#25071=CARTESIAN_POINT('Ctrl Pts',(149.663115656512,-81.8843266214971,36.2465205196001));
#25072=CARTESIAN_POINT('Ctrl Pts',(149.654955183208,-81.9145791058626,36.2325522508595));
#25073=CARTESIAN_POINT('Ctrl Pts',(149.646761444289,-81.9449339838539,36.2188226892616));
#25074=CARTESIAN_POINT('Ctrl Pts',(149.629599044989,-82.0085145472408,36.1900650951214));
#25075=CARTESIAN_POINT('Ctrl Pts',(149.612256027528,-82.0726719053387,36.1623178493608));
#25076=CARTESIAN_POINT('Ctrl Pts',(149.594776281622,-82.1372383448972,36.1354843276864));
#25077=CARTESIAN_POINT('Ctrl Pts',(149.575926055079,-82.206867046555,36.1065469526683));
#25078=CARTESIAN_POINT('Ctrl Pts',(149.556916727546,-82.2769718987435,36.0786720183343));
#25079=CARTESIAN_POINT('Ctrl Pts',(149.537787182918,-82.3473991049671,36.0517539381005));
#25080=CARTESIAN_POINT('Ctrl Pts',(149.532245072383,-82.3678029028164,36.043955374207));
#25081=CARTESIAN_POINT('Ctrl Pts',(149.526692780135,-82.388234072127,36.0362372267063));
#25082=CARTESIAN_POINT('Ctrl Pts',(149.521131044556,-82.4086895813368,36.0285971804474));
#25083=CARTESIAN_POINT('Ctrl Pts',(149.513307047732,-82.4374654619684,36.0178495106188));
#25084=CARTESIAN_POINT('Ctrl Pts',(149.505462657808,-82.4662967316413,36.0072540693274));
#25085=CARTESIAN_POINT('Ctrl Pts',(149.497602582526,-82.4951656239004,35.9968087539209));
#25086=CARTESIAN_POINT('Ctrl Pts',(149.466886299739,-82.6079819808148,35.9559896459205));
#25087=CARTESIAN_POINT('Ctrl Pts',(149.435949796432,-82.7213062385209,35.9174537341537));
#25088=CARTESIAN_POINT('Ctrl Pts',(149.404819096531,-82.8350358342388,35.8808341283755));
#25089=CARTESIAN_POINT('Ctrl Pts',(149.382928718768,-82.9150078175565,35.8550840807832));
#25090=CARTESIAN_POINT('Ctrl Pts',(149.360942099001,-82.995181007926,35.830282544477));
#25091=CARTESIAN_POINT('Ctrl Pts',(149.338865605393,-83.0755291035976,35.806313699263));
#25092=CARTESIAN_POINT('Ctrl Pts',(149.30257270251,-83.2076182697845,35.766909843424));
#25093=CARTESIAN_POINT('Ctrl Pts',(149.266041574139,-83.3401623692397,35.7297345827405));
#25094=CARTESIAN_POINT('Ctrl Pts',(149.229255373738,-83.4732146574128,35.6944829487653));
#25095=CARTESIAN_POINT('Ctrl Pts',(149.222100057115,-83.4990947765574,35.6876261220257));
#25096=CARTESIAN_POINT('Ctrl Pts',(149.214935059986,-83.5249942184407,35.6808421975289));
#25097=CARTESIAN_POINT('Ctrl Pts',(149.207760216038,-83.5509135089673,35.6741291032872));
#25098=CARTESIAN_POINT('Ctrl Pts',(149.164019348336,-83.7089284102154,35.633203256085));
#25099=CARTESIAN_POINT('Ctrl Pts',(149.119950314816,-83.8675446159542,35.5949411222291));
#25100=CARTESIAN_POINT('Ctrl Pts',(149.075578120339,-84.026655594328,35.5589506769566));
#25101=CARTESIAN_POINT('Ctrl Pts',(149.050851325548,-84.1153215834144,35.5388946854696));
#25102=CARTESIAN_POINT('Ctrl Pts',(149.026030206988,-84.2041418314762,35.5195449132821));
#25103=CARTESIAN_POINT('Ctrl Pts',(149.001117827171,-84.2931021083258,35.5008388586839));
#25104=CARTESIAN_POINT('Ctrl Pts',(148.961812515426,-84.4334584869728,35.4713255278451));
#25105=CARTESIAN_POINT('Ctrl Pts',(148.922228706232,-84.5743409203763,35.4434175359834));
#25106=CARTESIAN_POINT('Ctrl Pts',(148.882458149795,-84.7154243069172,35.41702373575));
#25107=CARTESIAN_POINT('Ctrl Pts',(148.823378480021,-84.9250054803867,35.3778154082434));
#25108=CARTESIAN_POINT('Ctrl Pts',(148.763691428379,-85.1357176965696,35.341819392481));
#25109=CARTESIAN_POINT('Ctrl Pts',(148.703725142329,-85.3463732562435,35.3088731062242));
#25110=CARTESIAN_POINT('Ctrl Pts',(148.683093735234,-85.4188493239612,35.2975379329324));
#25111=CARTESIAN_POINT('Ctrl Pts',(148.662429146922,-85.4913191022936,35.2865639616474));
#25112=CARTESIAN_POINT('Ctrl Pts',(148.64174438629,-85.5637353575988,35.2759451993142));
#25113=CARTESIAN_POINT('Ctrl Pts',(148.565624143843,-85.8302283090543,35.2368679879471));
#25114=CARTESIAN_POINT('Ctrl Pts',(148.489028565031,-86.0967324995911,35.2024345741489));
#25115=CARTESIAN_POINT('Ctrl Pts',(148.411875341988,-86.3635238183438,35.1722187734539));
#25116=CARTESIAN_POINT('Ctrl Pts',(148.365096720961,-86.5252815453833,35.1538986899371));
#25117=CARTESIAN_POINT('Ctrl Pts',(148.318112978006,-86.6871449972432,35.1371301419325));
#25118=CARTESIAN_POINT('Ctrl Pts',(148.270904619886,-86.8491769961467,35.1218271577707));
#25119=CARTESIAN_POINT('Ctrl Pts',(148.24918654488,-86.9237193705385,35.1147870620956));
#25120=CARTESIAN_POINT('Ctrl Pts',(148.227421070419,-86.9982969676292,35.1080522041553));
#25121=CARTESIAN_POINT('Ctrl Pts',(148.205605817643,-87.0729174681581,35.1016219420904));
#25122=CARTESIAN_POINT('Ctrl Pts',(148.101900684429,-87.4276476666717,35.0710538257873));
#25123=CARTESIAN_POINT('Ctrl Pts',(147.997167488692,-87.7829762387848,35.0474026554915));
#25124=CARTESIAN_POINT('Ctrl Pts',(147.891499227194,-88.1385323929298,35.0306489701688));
#25125=CARTESIAN_POINT('Ctrl Pts',(147.785745335362,-88.4943766789275,35.0138817081711));
#25126=CARTESIAN_POINT('Ctrl Pts',(147.679054863976,-88.850448864948,35.0040231183135));
#25127=CARTESIAN_POINT('Ctrl Pts',(147.571529965732,-89.2063722196202,35.0010024709204));
#25128=CARTESIAN_POINT('Ctrl Pts',(147.547727111396,-89.2851631964492,35.0003337883076));
#25129=CARTESIAN_POINT('Ctrl Pts',(147.523883400527,-89.3639468619882,35.));
#25130=CARTESIAN_POINT('Ctrl Pts',(147.5,-89.4427190999916,35.));
#25131=CARTESIAN_POINT('Origin',(152.5,-80.6225774829854,115.));
#25132=CARTESIAN_POINT('Origin',(152.5,-80.6225774829854,37.5));
#25133=CARTESIAN_POINT('Origin',(121.449578014911,-122.5,32.5));
#25134=CARTESIAN_POINT('Origin',(121.449578014911,-122.5,32.5));
#25135=CARTESIAN_POINT('Ctrl Pts',(150.289855072464,-79.4541343310581,37.5));
#25136=CARTESIAN_POINT('Ctrl Pts',(150.,-80.0024038100394,37.5));
#25137=CARTESIAN_POINT('Ctrl Pts',(150.,-80.6225774829855,37.5));
#25138=CARTESIAN_POINT('Ctrl Pts',(150.28985506853,-79.4541343384987,37.2405761439445));
#25139=CARTESIAN_POINT('Ctrl Pts',(149.999999996126,-80.0024038172978,37.3094148175638));
#25140=CARTESIAN_POINT('Ctrl Pts',(150.,-80.6225774905387,37.370288072025));
#25141=CARTESIAN_POINT('Ctrl Pts',(150.270119749701,-79.4914922605508,36.9888304197613));
#25142=CARTESIAN_POINT('Ctrl Pts',(149.980519833119,-80.0389466368966,37.1241843229264));
#25143=CARTESIAN_POINT('Ctrl Pts',(149.989987226484,-80.6604847938369,37.2444152098049));
#25144=CARTESIAN_POINT('Ctrl Pts',(150.196231486305,-79.6310132970258,36.4987912993743));
#25145=CARTESIAN_POINT('Ctrl Pts',(149.907890955038,-80.1748646486434,36.7663952057901));
#25146=CARTESIAN_POINT('Ctrl Pts',(149.952499797667,-80.8020576101747,36.9993956497629));
#25147=CARTESIAN_POINT('Ctrl Pts',(150.143050717941,-79.7313168859281,36.2679996568594));
#25148=CARTESIAN_POINT('Ctrl Pts',(149.855501091412,-80.272795283317,36.5988602080119));
#25149=CARTESIAN_POINT('Ctrl Pts',(149.925518380098,-80.9038362519448,36.8839998280977));
#25150=CARTESIAN_POINT('Ctrl Pts',(150.01502846971,-79.971931353987,35.8382849920617));
#25151=CARTESIAN_POINT('Ctrl Pts',(149.729850869406,-80.506872138187,36.2906206072006));
#25152=CARTESIAN_POINT('Ctrl Pts',(149.860565913637,-81.1479891679691,36.6691424963629));
#25153=CARTESIAN_POINT('Ctrl Pts',(149.939105635844,-80.1142600764838,35.6362636343074));
#25154=CARTESIAN_POINT('Ctrl Pts',(149.655266820466,-80.6454659182015,36.1475015807484));
#25155=CARTESIAN_POINT('Ctrl Pts',(149.8220462428,-81.2924109599909,36.5681318166794));
#25156=CARTESIAN_POINT('Ctrl Pts',(149.775363670977,-80.4199633406152,35.2663619775736));
#25157=CARTESIAN_POINT('Ctrl Pts',(149.494928348598,-80.9422362487713,35.8896065722342));
#25158=CARTESIAN_POINT('Ctrl Pts',(149.738971273161,-81.6026098603007,36.3831809892611));
#25159=CARTESIAN_POINT('Ctrl Pts',(149.686995608736,-80.5843780010491,35.096414733337));
#25160=CARTESIAN_POINT('Ctrl Pts',(149.408398325687,-81.1018541496878,35.7733074247595));
#25161=CARTESIAN_POINT('Ctrl Pts',(149.694137478568,-81.7694423834459,36.2982073663223));
#25162=CARTESIAN_POINT('Ctrl Pts',(149.500255462679,-80.9302925286903,34.7789058669457));
#25163=CARTESIAN_POINT('Ctrl Pts',(149.226078269656,-81.4367533718067,35.5604730905987));
#25164=CARTESIAN_POINT('Ctrl Pts',(149.599394315017,-82.1204438893779,36.1394529338191));
#25165=CARTESIAN_POINT('Ctrl Pts',(149.401347886678,-81.1127763961003,34.630789292851));
#25166=CARTESIAN_POINT('Ctrl Pts',(149.129574349817,-81.6133256610688,35.4636764519996));
#25167=CARTESIAN_POINT('Ctrl Pts',(149.549213266548,-82.3056113431187,36.0653946460504));
#25168=CARTESIAN_POINT('Ctrl Pts',(149.197899201605,-81.4863922312653,34.3564485886759));
#25169=CARTESIAN_POINT('Ctrl Pts',(148.931653199894,-81.9738530462045,35.2892543852115));
#25170=CARTESIAN_POINT('Ctrl Pts',(149.445992976772,-82.684721528767,35.928224294713));
#25171=CARTESIAN_POINT('Ctrl Pts',(149.093462145135,-81.6773447374821,34.2301909539054));
#25172=CARTESIAN_POINT('Ctrl Pts',(148.830186520417,-82.1578926315274,35.2116962088616));
#25173=CARTESIAN_POINT('Ctrl Pts',(149.393006529828,-82.8784821601051,35.8650954766799));
#25174=CARTESIAN_POINT('Ctrl Pts',(148.773324875584,-82.2599185303359,33.8775006940139));
#25175=CARTESIAN_POINT('Ctrl Pts',(148.518202139789,-82.721231742148,35.0014947689296));
#25176=CARTESIAN_POINT('Ctrl Pts',(149.230583943609,-83.4696232145796,35.6887503475526));
#25177=CARTESIAN_POINT('Ctrl Pts',(148.550873607932,-82.6611103319713,33.6767887272455));
#25178=CARTESIAN_POINT('Ctrl Pts',(148.30315471628,-83.1060920248233,34.8943924369605));
#25179=CARTESIAN_POINT('Ctrl Pts',(149.117722639557,-83.8767148956951,35.5883943633349));
#25180=CARTESIAN_POINT('Ctrl Pts',(148.091214058598,-83.4818155626998,33.3265667074903));
#25181=CARTESIAN_POINT('Ctrl Pts',(147.862495369544,-83.8874214153556,34.7305155228013));
#25182=CARTESIAN_POINT('Ctrl Pts',(148.884513014786,-84.7094893209564,35.413283354033));
#25183=CARTESIAN_POINT('Ctrl Pts',(147.853104568995,-83.9028862659541,33.1771134341875));
#25184=CARTESIAN_POINT('Ctrl Pts',(147.635229789714,-84.2865819284461,34.6752930801319));
#25185=CARTESIAN_POINT('Ctrl Pts',(148.763707465283,-85.1367522404598,35.3385567168472));
#25186=CARTESIAN_POINT('Ctrl Pts',(147.37234266623,-84.7444834282146,32.926677827892));
#25187=CARTESIAN_POINT('Ctrl Pts',(147.180928816249,-85.0771956930356,34.6125828689674));
#25188=CARTESIAN_POINT('Ctrl Pts',(148.519791499647,-85.9907258315643,35.2133389141925));
#25189=CARTESIAN_POINT('Ctrl Pts',(147.128665473946,-85.166872640511,32.8248617968328));
#25190=CARTESIAN_POINT('Ctrl Pts',(146.952267516985,-85.4713149459729,34.6060731019583));
#25191=CARTESIAN_POINT('Ctrl Pts',(148.396161159612,-86.4193266499342,35.162430898305));
#25192=CARTESIAN_POINT('Ctrl Pts',(146.388097896077,-86.4377602232181,32.58126559787));
#25193=CARTESIAN_POINT('Ctrl Pts',(146.253862108749,-86.6644852388335,34.6540449090446));
#25194=CARTESIAN_POINT('Ctrl Pts',(148.020432020732,-87.7089037559046,35.0406327991578));
#25195=CARTESIAN_POINT('Ctrl Pts',(145.881711078451,-87.289917999924,32.5000000009063));
#25196=CARTESIAN_POINT('Ctrl Pts',(145.791767290438,-87.4382443129918,34.7842689266371));
#25197=CARTESIAN_POINT('Ctrl Pts',(147.763515165397,-88.573593311031,35.));
#25198=CARTESIAN_POINT('Ctrl Pts',(145.36231884058,-88.1464478086874,32.5));
#25199=CARTESIAN_POINT('Ctrl Pts',(145.36231884058,-88.1464478086874,35.0000000000001));
#25200=CARTESIAN_POINT('Ctrl Pts',(147.5,-89.4427190999917,35.));
#25201=CARTESIAN_POINT('Origin',(147.5,-89.4427190999916,32.5));
#25202=CARTESIAN_POINT('Origin',(0.,0.,32.5));
#27531=UNCERTAINTY_MEASURE_WITH_UNIT(LENGTH_MEASURE(0.01),#27542,
'DISTANCE_ACCURACY_VALUE',
'Maximum model space distance between geometric entities at asserted c
onnectivities');
#27535=UNCERTAINTY_MEASURE_WITH_UNIT(LENGTH_MEASURE(0.01),#27542,
'DISTANCE_ACCURACY_VALUE',
'Maximum model space distance between geometric entities at asserted c
onnectivities');
#27537=(
GEOMETRIC_REPRESENTATION_CONTEXT(3)
GLOBAL_UNCERTAINTY_ASSIGNED_CONTEXT((#27531))
GLOBAL_UNIT_ASSIGNED_CONTEXT((#27542,#27544,#27545))
REPRESENTATION_CONTEXT('','3D')
);
#27541=(
GEOMETRIC_REPRESENTATION_CONTEXT(3)
GLOBAL_UNCERTAINTY_ASSIGNED_CONTEXT((#27535))
GLOBAL_UNIT_ASSIGNED_CONTEXT((#27542,#27544,#27545))
REPRESENTATION_CONTEXT('','3D')
);
#27542=(
LENGTH_UNIT()
NAMED_UNIT(*)
SI_UNIT(.MILLI.,.METRE.)
);
#27544=(
NAMED_UNIT(*)
PLANE_ANGLE_UNIT()
SI_UNIT($,.RADIAN.)
);
#27545=(
NAMED_UNIT(*)
SI_UNIT($,.STERADIAN.)
SOLID_ANGLE_UNIT()
);
#27547=SHAPE_DEFINITION_REPRESENTATION(#27552,#27561);
#27552=PRODUCT_DEFINITION_SHAPE('',$,#27567);
#27561=SHAPE_REPRESENTATION('',(#11896),#27537);
#27565=PRODUCT_DEFINITION_CONTEXT('part definition',#27582,'design');
#27567=PRODUCT_DEFINITION('1. Housing','1. Housing',#27572,#27565);
#27572=PRODUCT_DEFINITION_FORMATION('',$,#27585);
#27582=APPLICATION_CONTEXT(
'Core Data for Automotive Mechanical Design Process');
#27583=PRODUCT_CONTEXT('part definition',#27582,'mechanical');
#27585=PRODUCT('1. Housing','1. Housing',$,(#27583));
#27590=PRESENTATION_STYLE_ASSIGNMENT((#27594));
#27594=SURFACE_STYLE_USAGE(.BOTH.,#27598);
#27598=SURFACE_SIDE_STYLE('',(#27602));
#27602=SURFACE_STYLE_FILL_AREA(#27606);
#27606=FILL_AREA_STYLE('Opaque(20,51,87)',(#27610));
#27610=FILL_AREA_STYLE_COLOUR('Opaque(20,51,87)',#27614);
#27614=COLOUR_RGB('Opaque(20,51,87)',0.0784313725490196,0.2,0.341176470588235);
ENDSEC;
END-ISO-10303-21;
